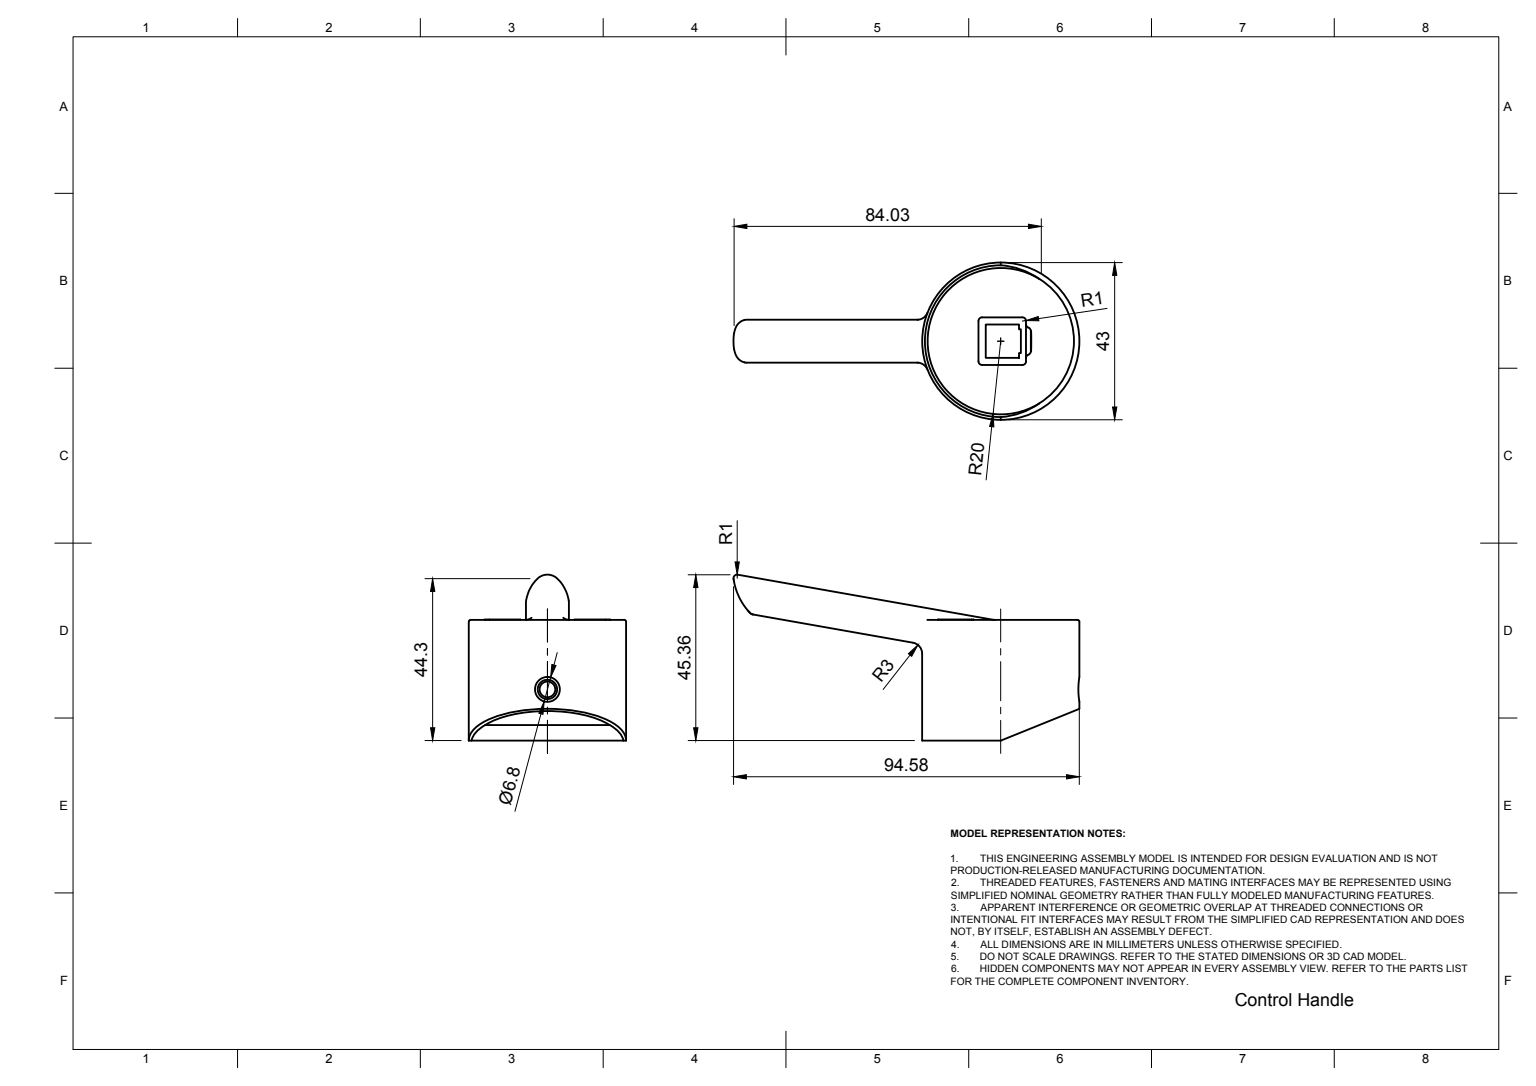
ISO-10303-21;
HEADER;
/* Generated by software containing ST-Developer
 * from STEP Tools, Inc. (www.steptools.com) 
 */

FILE_DESCRIPTION(
/* description */ ('STEP AP214'),
/* implementation_level */ '2;1');

FILE_NAME(
/* name */ 'Control Handle.step',
/* time_stamp */ '2026-10-05T23:18:41-07:00',
/* author */ (''),
/* organization */ (''),
/* preprocessor_version */ 'ST-DEVELOPER v20.2',
/* originating_system */ 'Autodesk Translation Framework v15.15.0.0',
/* authorisation */ '');

FILE_SCHEMA (('AUTOMOTIVE_DESIGN { 1 0 10303 214 3 1 1 }'));
ENDSEC;

DATA;
#10=MECHANICAL_DESIGN_GEOMETRIC_PRESENTATION_REPRESENTATION('',(#101),#221662);
#63=MANIFOLD_SOLID_BREP('Body1',#79323);
#75=SHAPE_REPRESENTATION_RELATIONSHIP('SRR','None',#221710,#88);
#88=ADVANCED_BREP_SHAPE_REPRESENTATION('',(#63),#221650);
#101=STYLED_ITEM('',(#221783),#63);
#176=B_SPLINE_SURFACE_WITH_KNOTS('',3,3,((#159336,#159337,#159338,#159339),
(#159340,#159341,#159342,#159343),(#159344,#159345,#159346,#159347),(#159348,
#159349,#159350,#159351),(#159352,#159353,#159354,#159355),(#159356,#159357,
#159358,#159359),(#159360,#159361,#159362,#159363),(#159364,#159365,#159366,
#159367),(#159368,#159369,#159370,#159371),(#159372,#159373,#159374,#159375),
(#159376,#159377,#159378,#159379),(#159380,#159381,#159382,#159383),(#159384,
#159385,#159386,#159387),(#159388,#159389,#159390,#159391),(#159392,#159393,
#159394,#159395),(#159396,#159397,#159398,#159399)),.UNSPECIFIED.,.F.,.F.,
 .F.,(4,1,1,1,1,1,1,1,1,1,1,1,1,4),(4,4),(0.,0.0631871049823428,0.143694780613763,
0.224202456245058,0.304710131876457,0.385217807507856,0.465725483139255,
0.54623315877055,0.626740834401949,0.707248510033348,0.787756185664748,
0.868263861296042,0.948771536927442,1.),(0.,1.),.UNSPECIFIED.);
#177=B_SPLINE_SURFACE_WITH_KNOTS('',3,3,((#159424,#159425,#159426,#159427),
(#159428,#159429,#159430,#159431),(#159432,#159433,#159434,#159435),(#159436,
#159437,#159438,#159439),(#159440,#159441,#159442,#159443),(#159444,#159445,
#159446,#159447),(#159448,#159449,#159450,#159451),(#159452,#159453,#159454,
#159455),(#159456,#159457,#159458,#159459),(#159460,#159461,#159462,#159463),
(#159464,#159465,#159466,#159467),(#159468,#159469,#159470,#159471),(#159472,
#159473,#159474,#159475),(#159476,#159477,#159478,#159479),(#159480,#159481,
#159482,#159483),(#159484,#159485,#159486,#159487)),.UNSPECIFIED.,.F.,.F.,
 .F.,(4,1,1,1,1,1,1,1,1,1,1,1,1,4),(4,4),(0.,0.063187150036898,0.143694817475814,
0.224202484914604,0.304710152353498,0.385217819792393,0.465725487231287,
0.546233154670077,0.626740822108972,0.707248489547867,0.787756156986761,
0.868263824425551,0.948771491864446,1.),(0.,1.),.UNSPECIFIED.);
#178=B_SPLINE_SURFACE_WITH_KNOTS('',3,1,((#159815,#159816),(#159817,#159818),
(#159819,#159820),(#159821,#159822)),.UNSPECIFIED.,.F.,.F.,.F.,(4,4),(2,
2),(0.00340538980800498,1.),(0.,1.18214433782264),.UNSPECIFIED.);
#269=FACE_BOUND('',#24594,.T.);
#270=FACE_BOUND('',#24605,.T.);
#271=FACE_BOUND('',#24611,.T.);
#272=FACE_BOUND('',#24616,.T.);
#273=FACE_BOUND('',#24644,.T.);
#274=FACE_BOUND('',#24645,.T.);
#1766=(
BOUNDED_CURVE()
B_SPLINE_CURVE(3,(#159803,#159804,#159805,#159806,#159807,#159808,#159809,
#159810,#159811,#159812,#159813),.UNSPECIFIED.,.F.,.F.)
B_SPLINE_CURVE_WITH_KNOTS((4,1,1,1,1,1,1,1,4),(0.,0.141779774422697,0.288564186808889,
0.419637721811095,0.537332459847568,0.657407795649981,0.783847578789506,
0.908572898255855,1.),.UNSPECIFIED.)
CURVE()
GEOMETRIC_REPRESENTATION_ITEM()
RATIONAL_B_SPLINE_CURVE((1.03357883859121,1.03357883859121,1.03357883859121,
1.03357883859121,1.03357883859121,1.03357883859121,1.03357883859121,1.03357883859121,
1.03357883859121,1.03357883859121,1.03357883859121))
REPRESENTATION_ITEM('')
);
#1767=(
BOUNDED_CURVE()
B_SPLINE_CURVE(3,(#159870,#159871,#159872,#159873,#159874,#159875,#159876),
 .UNSPECIFIED.,.F.,.F.)
B_SPLINE_CURVE_WITH_KNOTS((4,1,1,1,4),(0.,0.224667526957694,0.481948378364901,
0.749503179488002,1.),.UNSPECIFIED.)
CURVE()
GEOMETRIC_REPRESENTATION_ITEM()
RATIONAL_B_SPLINE_CURVE((1.24731983145218,1.24731983145218,1.24731983145218,
1.24731983145218,1.24731983145218,1.24731983145218,1.24731983145218))
REPRESENTATION_ITEM('')
);
#1768=(
BOUNDED_CURVE()
B_SPLINE_CURVE(3,(#159878,#159879,#159880,#159881,#159882,#159883,#159884,
#159885,#159886,#159887),.UNSPECIFIED.,.F.,.F.)
B_SPLINE_CURVE_WITH_KNOTS((4,1,1,1,1,1,1,4),(0.,0.122671457527971,0.275186389436719,
0.426161388513612,0.576657904418794,0.727651491077518,0.880206170558277,
1.),.UNSPECIFIED.)
CURVE()
GEOMETRIC_REPRESENTATION_ITEM()
RATIONAL_B_SPLINE_CURVE((1.26434380601904,1.26434380601904,1.26434380601904,
1.26434380601904,1.26434380601904,1.26434380601904,1.26434380601904,1.26434380601904,
1.26434380601904,1.26434380601904))
REPRESENTATION_ITEM('')
);
#1769=(
BOUNDED_CURVE()
B_SPLINE_CURVE(3,(#159888,#159889,#159890,#159891,#159892,#159893,#159894),
 .UNSPECIFIED.,.F.,.F.)
B_SPLINE_CURVE_WITH_KNOTS((4,1,1,1,4),(0.,0.253269801031687,0.52066383235046,
0.77788908313976,0.999999610731203),.UNSPECIFIED.)
CURVE()
GEOMETRIC_REPRESENTATION_ITEM()
RATIONAL_B_SPLINE_CURVE((1.24732214149726,1.24732214149726,1.24732214149726,
1.24732214149726,1.24732214149726,1.24732214149726,1.24732214149726))
REPRESENTATION_ITEM('')
);
#1878=TOROIDAL_SURFACE('',#80380,21.,0.5);
#1879=TOROIDAL_SURFACE('',#80400,18.5,1.5);
#1880=TOROIDAL_SURFACE('',#80403,2.866784855558,1.5);
#1881=TOROIDAL_SURFACE('',#80406,2.866784855558,1.5);
#1882=TOROIDAL_SURFACE('',#80441,2.866784855558,1.5);
#1883=TOROIDAL_SURFACE('',#80446,2.866784855558,1.5);
#1884=TOROIDAL_SURFACE('',#80451,2.866784855558,1.5);
#1885=TOROIDAL_SURFACE('',#80473,2.866784855558,1.5);
#1924=CONICAL_SURFACE('',#80396,20.37470056578,0.174533028825274);
#1925=CONICAL_SURFACE('',#80430,1.183506656857,0.0174532924999985);
#1926=CONICAL_SURFACE('',#80434,1.183506656857,0.0174532924999985);
#1927=CONICAL_SURFACE('',#80455,1.183506656857,0.0174532924999985);
#1928=CONICAL_SURFACE('',#80460,0.816493292676001,0.0174532924999985);
#1929=CONICAL_SURFACE('',#80464,1.189214422822,0.0174532924999985);
#1930=CONICAL_SURFACE('',#80467,1.189214422821,0.0174532924999985);
#1931=CONICAL_SURFACE('',#80476,1.183506656857,0.0174532924999985);
#1932=CONICAL_SURFACE('',#80479,0.816493289244397,0.0174532924999985);
#2150=CYLINDRICAL_SURFACE('',#80384,21.5);
#2151=CYLINDRICAL_SURFACE('',#80388,15.00000000001);
#2152=CYLINDRICAL_SURFACE('',#80389,20.);
#2153=CYLINDRICAL_SURFACE('',#80395,3.40000000000001);
#2154=CYLINDRICAL_SURFACE('',#80409,2.15);
#2155=CYLINDRICAL_SURFACE('',#80412,19.);
#2156=CYLINDRICAL_SURFACE('',#80417,17.5);
#2157=CYLINDRICAL_SURFACE('',#80423,19.);
#2158=CYLINDRICAL_SURFACE('',#80426,17.5);
#2159=CYLINDRICAL_SURFACE('',#80438,1.50000000000001);
#2160=CYLINDRICAL_SURFACE('',#80444,1.50000000000001);
#2161=CYLINDRICAL_SURFACE('',#80449,1.50000000000001);
#2162=CYLINDRICAL_SURFACE('',#80458,1.50000000000001);
#2163=CYLINDRICAL_SURFACE('',#80469,1.50000000000001);
#2164=CYLINDRICAL_SURFACE('',#80471,1.50000000000001);
#2165=CYLINDRICAL_SURFACE('',#80500,2.50000000000001);
#2166=CYLINDRICAL_SURFACE('',#80503,2.50000000000001);
#2167=CYLINDRICAL_SURFACE('',#80507,10.);
#2168=CYLINDRICAL_SURFACE('',#80512,10.);
#2169=CYLINDRICAL_SURFACE('',#80514,4.00000000000099);
#2615=(
BOUNDED_SURFACE()
B_SPLINE_SURFACE(3,3,((#159279,#159280,#159281,#159282,#159283,#159284,
#159285,#159286,#159287,#159288,#159289,#159290,#159291),(#159292,#159293,
#159294,#159295,#159296,#159297,#159298,#159299,#159300,#159301,#159302,
#159303,#159304),(#159305,#159306,#159307,#159308,#159309,#159310,#159311,
#159312,#159313,#159314,#159315,#159316,#159317),(#159318,#159319,#159320,
#159321,#159322,#159323,#159324,#159325,#159326,#159327,#159328,#159329,
#159330)),.UNSPECIFIED.,.F.,.F.,.F.)
B_SPLINE_SURFACE_WITH_KNOTS((4,4),(4,1,1,1,1,1,1,1,1,1,4),(0.,1.),(0.,0.0348134269562723,
0.158608211677217,0.280646015430893,0.400635489137686,0.518375328151176,
0.633927632286859,0.74698660160379,0.85748053072882,0.966231997819705,1.),
 .UNSPECIFIED.)
GEOMETRIC_REPRESENTATION_ITEM()
RATIONAL_B_SPLINE_SURFACE(((1.216775993711,1.216775993711,1.216775993711,
1.216775993711,1.216775993711,1.216775993711,1.216775993711,1.216775993711,
1.216775993711,1.216775993711,1.216775993711,1.216775993711,1.216775993711),
(0.9277413354296,0.9277413354296,0.9277413354296,0.9277413354296,0.9277413354296,
0.9277413354296,0.9277413354296,0.9277413354296,0.9277413354296,0.9277413354296,
0.9277413354296,0.9277413354296,0.9277413354296),(0.9277413354296,0.9277413354296,
0.9277413354296,0.9277413354296,0.9277413354296,0.9277413354296,0.9277413354296,
0.9277413354296,0.9277413354296,0.9277413354296,0.9277413354296,0.9277413354296,
0.9277413354296),(1.216775993711,1.216775993711,1.216775993711,1.216775993711,
1.216775993711,1.216775993711,1.216775993711,1.216775993711,1.216775993711,
1.216775993711,1.216775993711,1.216775993711,1.216775993711)))
REPRESENTATION_ITEM('')
SURFACE()
);
#2616=(
BOUNDED_SURFACE()
B_SPLINE_SURFACE(3,3,((#159523,#159524,#159525,#159526,#159527,#159528,
#159529,#159530,#159531,#159532,#159533,#159534,#159535),(#159536,#159537,
#159538,#159539,#159540,#159541,#159542,#159543,#159544,#159545,#159546,
#159547,#159548),(#159549,#159550,#159551,#159552,#159553,#159554,#159555,
#159556,#159557,#159558,#159559,#159560,#159561),(#159562,#159563,#159564,
#159565,#159566,#159567,#159568,#159569,#159570,#159571,#159572,#159573,
#159574)),.UNSPECIFIED.,.F.,.F.,.F.)
B_SPLINE_SURFACE_WITH_KNOTS((4,4),(4,1,1,1,1,1,1,1,1,1,4),(0.,1.),(0.,0.0348134437205886,
0.158607302135055,0.280647732326047,0.400637496360499,0.518378147625292,
0.633929635661477,0.746988357647408,0.857493579740769,0.966231987897078,
1.),.UNSPECIFIED.)
GEOMETRIC_REPRESENTATION_ITEM()
RATIONAL_B_SPLINE_SURFACE(((1.216775996933,1.216775996933,1.216775996933,
1.216775996933,1.216775996933,1.216775996933,1.216775996933,1.216775996933,
1.216775996933,1.216775996933,1.216775996933,1.216775996933,1.216775996933),
(0.9277413343557,0.9277413343557,0.9277413343557,0.9277413343557,0.9277413343557,
0.9277413343557,0.9277413343557,0.9277413343557,0.9277413343557,0.9277413343557,
0.9277413343557,0.9277413343557,0.9277413343557),(0.9277413343557,0.9277413343557,
0.9277413343557,0.9277413343557,0.9277413343557,0.9277413343557,0.9277413343557,
0.9277413343557,0.9277413343557,0.9277413343557,0.9277413343557,0.9277413343557,
0.9277413343557),(1.216775996933,1.216775996933,1.216775996933,1.216775996933,
1.216775996933,1.216775996933,1.216775996933,1.216775996933,1.216775996933,
1.216775996933,1.216775996933,1.216775996933,1.216775996933)))
REPRESENTATION_ITEM('')
SURFACE()
);
#2617=(
BOUNDED_SURFACE()
B_SPLINE_SURFACE(3,3,((#159756,#159757,#159758,#159759,#159760,#159761,
#159762,#159763,#159764,#159765,#159766),(#159767,#159768,#159769,#159770,
#159771,#159772,#159773,#159774,#159775,#159776,#159777),(#159778,#159779,
#159780,#159781,#159782,#159783,#159784,#159785,#159786,#159787,#159788),
(#159789,#159790,#159791,#159792,#159793,#159794,#159795,#159796,#159797,
#159798,#159799)),.UNSPECIFIED.,.F.,.F.,.F.)
B_SPLINE_SURFACE_WITH_KNOTS((4,4),(4,1,1,1,1,1,1,1,4),(0.,1.),(0.,0.148763869419657,
0.292686130252006,0.421203860344306,0.536603666842246,0.654337651793038,
0.778311983622731,0.900605282133238,1.),.UNSPECIFIED.)
GEOMETRIC_REPRESENTATION_ITEM()
RATIONAL_B_SPLINE_SURFACE(((1.068703746667,1.068703746667,1.068703746667,
1.068703746667,1.068703746667,1.068703746667,1.068703746667,1.068703746667,
1.068703746667,1.068703746667,1.068703746667),(0.9770987511109,0.9770987511109,
0.9770987511109,0.9770987511109,0.9770987511109,0.9770987511109,0.9770987511109,
0.9770987511109,0.9770987511109,0.9770987511109,0.9770987511109),(0.9770987511109,
0.9770987511109,0.9770987511109,0.9770987511109,0.9770987511109,0.9770987511109,
0.9770987511109,0.9770987511109,0.9770987511109,0.9770987511109,0.9770987511109),
(1.068703746667,1.068703746667,1.068703746667,1.068703746667,1.068703746667,
1.068703746667,1.068703746667,1.068703746667,1.068703746667,1.068703746667,
1.068703746667)))
REPRESENTATION_ITEM('')
SURFACE()
);
#2618=(
BOUNDED_SURFACE()
B_SPLINE_SURFACE(3,3,((#159895,#159896,#159897,#159898,#159899,#159900,
#159901,#159902,#159903,#159904),(#159905,#159906,#159907,#159908,#159909,
#159910,#159911,#159912,#159913,#159914),(#159915,#159916,#159917,#159918,
#159919,#159920,#159921,#159922,#159923,#159924),(#159925,#159926,#159927,
#159928,#159929,#159930,#159931,#159932,#159933,#159934)),.UNSPECIFIED.,
 .F.,.F.,.F.)
B_SPLINE_SURFACE_WITH_KNOTS((4,4),(4,1,1,1,1,1,1,4),(0.,1.),(0.,0.0982957502815311,
0.222717520122402,0.361997328765986,0.517413543628817,0.685998740299415,
0.858955544446863,1.),.UNSPECIFIED.)
GEOMETRIC_REPRESENTATION_ITEM()
RATIONAL_B_SPLINE_SURFACE(((1.298412003099,1.298412003099,1.298412003099,
1.298412003099,1.298412003099,1.298412003099,1.298412003099,1.298412003099,
1.298412003099,1.298412003099),(0.9005293323002,0.9005293323002,0.9005293323002,
0.9005293323002,0.9005293323002,0.9005293323002,0.9005293323002,0.9005293323002,
0.9005293323002,0.9005293323002),(0.9005293323002,0.9005293323002,0.9005293323002,
0.9005293323002,0.9005293323002,0.9005293323002,0.9005293323002,0.9005293323002,
0.9005293323002,0.9005293323002),(1.298412003099,1.298412003099,1.298412003099,
1.298412003099,1.298412003099,1.298412003099,1.298412003099,1.298412003099,
1.298412003099,1.298412003099)))
REPRESENTATION_ITEM('')
SURFACE()
);
#2619=(
BOUNDED_SURFACE()
B_SPLINE_SURFACE(3,3,((#160037,#160038,#160039,#160040,#160041,#160042,
#160043,#160044,#160045,#160046,#160047),(#160048,#160049,#160050,#160051,
#160052,#160053,#160054,#160055,#160056,#160057,#160058),(#160059,#160060,
#160061,#160062,#160063,#160064,#160065,#160066,#160067,#160068,#160069),
(#160070,#160071,#160072,#160073,#160074,#160075,#160076,#160077,#160078,
#160079,#160080)),.UNSPECIFIED.,.F.,.F.,.F.)
B_SPLINE_SURFACE_WITH_KNOTS((4,4),(4,1,1,1,1,1,1,1,4),(0.,1.),(0.,0.113847052245463,
0.256880770340595,0.393447274181346,0.529715276691642,0.664740251429543,
0.79675578013572,0.925830065497239,1.),.UNSPECIFIED.)
GEOMETRIC_REPRESENTATION_ITEM()
RATIONAL_B_SPLINE_SURFACE(((1.14428616678,1.14428616678,1.14428616678,1.14428616678,
1.14428616678,1.14428616678,1.14428616678,1.14428616678,1.14428616678,1.14428616678,
1.14428616678),(0.9519046110735,0.9519046110735,0.9519046110735,0.9519046110735,
0.9519046110735,0.9519046110735,0.9519046110735,0.9519046110735,0.9519046110735,
0.9519046110735,0.9519046110735),(0.9519046110735,0.9519046110735,0.9519046110735,
0.9519046110735,0.9519046110735,0.9519046110735,0.9519046110735,0.9519046110735,
0.9519046110735,0.9519046110735,0.9519046110735),(1.14428616678,1.14428616678,
1.14428616678,1.14428616678,1.14428616678,1.14428616678,1.14428616678,1.14428616678,
1.14428616678,1.14428616678,1.14428616678)))
REPRESENTATION_ITEM('')
SURFACE()
);
#2620=(
BOUNDED_SURFACE()
B_SPLINE_SURFACE(3,3,((#160180,#160181,#160182,#160183,#160184,#160185,
#160186,#160187,#160188,#160189,#160190),(#160191,#160192,#160193,#160194,
#160195,#160196,#160197,#160198,#160199,#160200,#160201),(#160202,#160203,
#160204,#160205,#160206,#160207,#160208,#160209,#160210,#160211,#160212),
(#160213,#160214,#160215,#160216,#160217,#160218,#160219,#160220,#160221,
#160222,#160223)),.UNSPECIFIED.,.F.,.F.,.F.)
B_SPLINE_SURFACE_WITH_KNOTS((4,4),(4,1,1,1,1,1,1,1,4),(0.,1.),(0.,0.0944145406001002,
0.22382893510453,0.356121659603939,0.491296333098967,0.627233999913856,
0.763922934472171,0.907653635910875,1.),.UNSPECIFIED.)
GEOMETRIC_REPRESENTATION_ITEM()
RATIONAL_B_SPLINE_SURFACE(((1.144284885867,1.144284885867,1.144284885867,
1.144284885867,1.144284885867,1.144284885867,1.144284885867,1.144284885867,
1.144284885867,1.144284885867,1.144284885867),(0.9519050380443,0.9519050380443,
0.9519050380443,0.9519050380443,0.9519050380443,0.9519050380443,0.9519050380443,
0.9519050380443,0.9519050380443,0.9519050380443,0.9519050380443),(0.9519050380443,
0.9519050380443,0.9519050380443,0.9519050380443,0.9519050380443,0.9519050380443,
0.9519050380443,0.9519050380443,0.9519050380443,0.9519050380443,0.9519050380443),
(1.144284885867,1.144284885867,1.144284885867,1.144284885867,1.144284885867,
1.144284885867,1.144284885867,1.144284885867,1.144284885867,1.144284885867,
1.144284885867)))
REPRESENTATION_ITEM('')
SURFACE()
);
#2621=(
BOUNDED_SURFACE()
B_SPLINE_SURFACE(3,3,((#160430,#160431,#160432,#160433,#160434,#160435,
#160436,#160437,#160438,#160439),(#160440,#160441,#160442,#160443,#160444,
#160445,#160446,#160447,#160448,#160449),(#160450,#160451,#160452,#160453,
#160454,#160455,#160456,#160457,#160458,#160459),(#160460,#160461,#160462,
#160463,#160464,#160465,#160466,#160467,#160468,#160469)),.UNSPECIFIED.,
 .F.,.F.,.F.)
B_SPLINE_SURFACE_WITH_KNOTS((4,4),(4,1,1,1,1,1,1,4),(0.,1.),(0.,0.146101495488384,
0.319452627218425,0.487967212214235,0.642996851728068,0.781791002263477,
0.905806643913708,1.),.UNSPECIFIED.)
GEOMETRIC_REPRESENTATION_ITEM()
RATIONAL_B_SPLINE_SURFACE(((1.298413325381,1.298413325381,1.298413325381,
1.298413325381,1.298413325381,1.298413325381,1.298413325381,1.298413325381,
1.298413325381,1.298413325381),(0.9005288915396,0.9005288915396,0.9005288915396,
0.9005288915396,0.9005288915396,0.9005288915396,0.9005288915396,0.9005288915396,
0.9005288915396,0.9005288915396),(0.9005288915396,0.9005288915396,0.9005288915396,
0.9005288915396,0.9005288915396,0.9005288915396,0.9005288915396,0.9005288915396,
0.9005288915396,0.9005288915396),(1.298413325381,1.298413325381,1.298413325381,
1.298413325381,1.298413325381,1.298413325381,1.298413325381,1.298413325381,
1.298413325381,1.298413325381)))
REPRESENTATION_ITEM('')
SURFACE()
);
#2622=(
BOUNDED_SURFACE()
B_SPLINE_SURFACE(3,3,((#160471,#160472,#160473,#160474,#160475,#160476,
#160477),(#160478,#160479,#160480,#160481,#160482,#160483,#160484),(#160485,
#160486,#160487,#160488,#160489,#160490,#160491),(#160492,#160493,#160494,
#160495,#160496,#160497,#160498)),.UNSPECIFIED.,.F.,.F.,.F.)
B_SPLINE_SURFACE_WITH_KNOTS((4,4),(4,1,1,1,4),(0.,1.),(0.,0.230593160213399,
0.482348490956705,0.744157121798399,1.),.UNSPECIFIED.)
GEOMETRIC_REPRESENTATION_ITEM()
RATIONAL_B_SPLINE_SURFACE(((1.353838625123,1.353838625123,1.353838625123,
1.353838625123,1.353838625123,1.353838625123,1.353838625123),(0.8820537916258,
0.8820537916258,0.8820537916258,0.8820537916258,0.8820537916258,0.8820537916258,
0.8820537916258),(0.8820537916258,0.8820537916258,0.8820537916258,0.8820537916258,
0.8820537916258,0.8820537916258,0.8820537916258),(1.353838625123,1.353838625123,
1.353838625123,1.353838625123,1.353838625123,1.353838625123,1.353838625123)))
REPRESENTATION_ITEM('')
SURFACE()
);
#2623=(
BOUNDED_SURFACE()
B_SPLINE_SURFACE(3,3,((#160516,#160517,#160518,#160519,#160520,#160521,
#160522,#160523,#160524,#160525),(#160526,#160527,#160528,#160529,#160530,
#160531,#160532,#160533,#160534,#160535),(#160536,#160537,#160538,#160539,
#160540,#160541,#160542,#160543,#160544,#160545),(#160546,#160547,#160548,
#160549,#160550,#160551,#160552,#160553,#160554,#160555)),.UNSPECIFIED.,
 .F.,.F.,.F.)
B_SPLINE_SURFACE_WITH_KNOTS((4,4),(4,1,1,1,1,1,1,4),(0.,1.),(0.,0.13457163316798,
0.282274649724905,0.428486319030034,0.574234601524777,0.720464271965091,
0.868205782040083,1.),.UNSPECIFIED.)
GEOMETRIC_REPRESENTATION_ITEM()
RATIONAL_B_SPLINE_SURFACE(((1.375941287385,1.375941287385,1.375941287385,
1.375941287385,1.375941287385,1.375941287385,1.375941287385,1.375941287385,
1.375941287385,1.375941287385),(0.8746862375382,0.8746862375382,0.8746862375382,
0.8746862375382,0.8746862375382,0.8746862375382,0.8746862375382,0.8746862375382,
0.8746862375382,0.8746862375382),(0.8746862375382,0.8746862375382,0.8746862375382,
0.8746862375382,0.8746862375382,0.8746862375382,0.8746862375382,0.8746862375382,
0.8746862375382,0.8746862375382),(1.375941287385,1.375941287385,1.375941287385,
1.375941287385,1.375941287385,1.375941287385,1.375941287385,1.375941287385,
1.375941287385,1.375941287385)))
REPRESENTATION_ITEM('')
SURFACE()
);
#2624=(
BOUNDED_SURFACE()
B_SPLINE_SURFACE(3,3,((#160619,#160620,#160621,#160622,#160623,#160624,
#160625),(#160626,#160627,#160628,#160629,#160630,#160631,#160632),(#160633,
#160634,#160635,#160636,#160637,#160638,#160639),(#160640,#160641,#160642,
#160643,#160644,#160645,#160646)),.UNSPECIFIED.,.F.,.F.,.F.)
B_SPLINE_SURFACE_WITH_KNOTS((4,4),(4,1,1,1,4),(0.,1.),(0.,0.266221048065604,
0.525168076403688,0.774267556960161,1.),.UNSPECIFIED.)
GEOMETRIC_REPRESENTATION_ITEM()
RATIONAL_B_SPLINE_SURFACE(((1.35383923737,1.35383923737,1.35383923737,1.35383923737,
1.35383923737,1.35383923737,1.35383923737),(0.8820535875433,0.8820535875433,
0.8820535875433,0.8820535875433,0.8820535875433,0.8820535875433,0.8820535875433),
(0.8820535875433,0.8820535875433,0.8820535875433,0.8820535875433,0.8820535875433,
0.8820535875433,0.8820535875433),(1.35383923737,1.35383923737,1.35383923737,
1.35383923737,1.35383923737,1.35383923737,1.35383923737)))
REPRESENTATION_ITEM('')
SURFACE()
);
#2625=(
BOUNDED_SURFACE()
B_SPLINE_SURFACE(3,3,((#160766,#160767,#160768,#160769,#160770,#160771),
(#160772,#160773,#160774,#160775,#160776,#160777),(#160778,#160779,#160780,
#160781,#160782,#160783),(#160784,#160785,#160786,#160787,#160788,#160789)),
 .UNSPECIFIED.,.F.,.F.,.F.)
B_SPLINE_SURFACE_WITH_KNOTS((4,4),(4,1,1,4),(0.,1.),(0.,0.343001553297945,
0.735822721578711,1.),.UNSPECIFIED.)
GEOMETRIC_REPRESENTATION_ITEM()
RATIONAL_B_SPLINE_SURFACE(((1.133911518843,1.133911518843,1.133911518843,
1.133911518843,1.133911518843,1.133911518843),(0.9553628270522,0.9553628270522,
0.9553628270522,0.9553628270522,0.9553628270522,0.9553628270522),(0.9553628270522,
0.9553628270522,0.9553628270522,0.9553628270522,0.9553628270522,0.9553628270522),
(1.133911518843,1.133911518843,1.133911518843,1.133911518843,1.133911518843,
1.133911518843)))
REPRESENTATION_ITEM('')
SURFACE()
);
#2626=(
BOUNDED_SURFACE()
B_SPLINE_SURFACE(3,3,((#160791,#160792,#160793,#160794,#160795,#160796),
(#160797,#160798,#160799,#160800,#160801,#160802),(#160803,#160804,#160805,
#160806,#160807,#160808),(#160809,#160810,#160811,#160812,#160813,#160814)),
 .UNSPECIFIED.,.F.,.F.,.F.)
B_SPLINE_SURFACE_WITH_KNOTS((4,4),(4,1,1,4),(0.,1.),(0.,0.326783840018485,
0.677637015410791,1.),.UNSPECIFIED.)
GEOMETRIC_REPRESENTATION_ITEM()
RATIONAL_B_SPLINE_SURFACE(((1.154127816646,1.154127816646,1.154127816646,
1.154127816646,1.154127816646,1.154127816646),(0.948624061118,0.948624061118,
0.948624061118,0.948624061118,0.948624061118,0.948624061118),(0.948624061118,
0.948624061118,0.948624061118,0.948624061118,0.948624061118,0.948624061118),
(1.154127816646,1.154127816646,1.154127816646,1.154127816646,1.154127816646,
1.154127816646)))
REPRESENTATION_ITEM('')
SURFACE()
);
#2627=(
BOUNDED_SURFACE()
B_SPLINE_SURFACE(3,3,((#160816,#160817,#160818,#160819,#160820,#160821),
(#160822,#160823,#160824,#160825,#160826,#160827),(#160828,#160829,#160830,
#160831,#160832,#160833),(#160834,#160835,#160836,#160837,#160838,#160839)),
 .UNSPECIFIED.,.F.,.F.,.F.)
B_SPLINE_SURFACE_WITH_KNOTS((4,4),(4,1,1,4),(0.,1.),(0.,0.325921012985495,
0.684444108359778,1.),.UNSPECIFIED.)
GEOMETRIC_REPRESENTATION_ITEM()
RATIONAL_B_SPLINE_SURFACE(((1.154128041374,1.154128041374,1.154128041374,
1.154128041374,1.154128041374,1.154128041374),(0.9486239862088,0.9486239862088,
0.9486239862088,0.9486239862088,0.9486239862088,0.9486239862088),(0.9486239862088,
0.9486239862088,0.9486239862088,0.9486239862088,0.9486239862088,0.9486239862088),
(1.154128041374,1.154128041374,1.154128041374,1.154128041374,1.154128041374,
1.154128041374)))
REPRESENTATION_ITEM('')
SURFACE()
);
#2628=(
BOUNDED_SURFACE()
B_SPLINE_SURFACE(3,3,((#160840,#160841,#160842,#160843,#160844,#160845),
(#160846,#160847,#160848,#160849,#160850,#160851),(#160852,#160853,#160854,
#160855,#160856,#160857),(#160858,#160859,#160860,#160861,#160862,#160863)),
 .UNSPECIFIED.,.F.,.F.,.F.)
B_SPLINE_SURFACE_WITH_KNOTS((4,4),(4,1,1,4),(0.,1.),(0.,0.298212289448515,
0.67415586424402,1.),.UNSPECIFIED.)
GEOMETRIC_REPRESENTATION_ITEM()
RATIONAL_B_SPLINE_SURFACE(((1.133911518295,1.133911518295,1.133911518295,
1.133911518295,1.133911518295,1.133911518295),(0.955362827235,0.955362827235,
0.955362827235,0.955362827235,0.955362827235,0.955362827235),(0.955362827235,
0.955362827235,0.955362827235,0.955362827235,0.955362827235,0.955362827235),
(1.133911518295,1.133911518295,1.133911518295,1.133911518295,1.133911518295,
1.133911518295)))
REPRESENTATION_ITEM('')
SURFACE()
);
#2629=(
BOUNDED_SURFACE()
B_SPLINE_SURFACE(3,3,((#161268,#161269,#161270,#161271,#161272,#161273,
#161274,#161275,#161276,#161277,#161278,#161279,#161280,#161281,#161282,
#161283,#161284,#161285,#161286,#161287,#161288,#161289,#161290,#161291,
#161292,#161293,#161294,#161295,#161296,#161297,#161298,#161299,#161300,
#161301,#161302,#161303,#161304,#161305,#161306,#161307),(#161308,#161309,
#161310,#161311,#161312,#161313,#161314,#161315,#161316,#161317,#161318,
#161319,#161320,#161321,#161322,#161323,#161324,#161325,#161326,#161327,
#161328,#161329,#161330,#161331,#161332,#161333,#161334,#161335,#161336,
#161337,#161338,#161339,#161340,#161341,#161342,#161343,#161344,#161345,
#161346,#161347),(#161348,#161349,#161350,#161351,#161352,#161353,#161354,
#161355,#161356,#161357,#161358,#161359,#161360,#161361,#161362,#161363,
#161364,#161365,#161366,#161367,#161368,#161369,#161370,#161371,#161372,
#161373,#161374,#161375,#161376,#161377,#161378,#161379,#161380,#161381,
#161382,#161383,#161384,#161385,#161386,#161387),(#161388,#161389,#161390,
#161391,#161392,#161393,#161394,#161395,#161396,#161397,#161398,#161399,
#161400,#161401,#161402,#161403,#161404,#161405,#161406,#161407,#161408,
#161409,#161410,#161411,#161412,#161413,#161414,#161415,#161416,#161417,
#161418,#161419,#161420,#161421,#161422,#161423,#161424,#161425,#161426,
#161427)),.UNSPECIFIED.,.F.,.F.,.F.)
B_SPLINE_SURFACE_WITH_KNOTS((4,4),(4,1,1,1,1,1,1,1,1,1,1,1,1,1,1,1,1,1,
1,1,1,1,1,1,1,1,1,1,1,1,1,1,1,1,1,1,1,4),(0.,1.),(0.,0.0080855657193485,
0.0596218558242468,0.106852501388389,0.150184164955898,0.19003235366263,
0.226816246755187,0.260884487830858,0.292377213220895,0.321411667226958,
0.348115402080392,0.372633477126632,0.395157121664735,0.415908415220206,
0.434997267820443,0.452409696784467,0.468313480733662,0.482712550753752,
0.495419214437213,0.507133333503985,0.519448003687265,0.533357648922,0.548832281415337,
0.566241232560042,0.585544933168279,0.606300542403394,0.628001557637231,
0.650281261920833,0.673235965567153,0.698456243264167,0.725991202217506,
0.755882932612454,0.78864738633083,0.824762418308521,0.864558914403212,
0.908348167961349,0.956921864249176,1.),.UNSPECIFIED.)
GEOMETRIC_REPRESENTATION_ITEM()
RATIONAL_B_SPLINE_SURFACE(((1.046091568931,1.046091568931,1.046091568931,
1.046091568931,1.046091568931,1.046091568931,1.046091568931,1.046091568931,
1.046091568931,1.046091568931,1.046091568931,1.046091568931,1.046091568931,
1.046091568931,1.046091568931,1.046091568931,1.046091568931,1.046091568931,
1.046091568931,1.046091568931,1.046091568931,1.046091568931,1.046091568931,
1.046091568931,1.046091568931,1.046091568931,1.046091568931,1.046091568931,
1.046091568931,1.046091568931,1.046091568931,1.046091568931,1.046091568931,
1.046091568931,1.046091568931,1.046091568931,1.046091568931,1.046091568931,
1.046091568931,1.046091568931),(0.9846361436895,0.9846361436895,0.9846361436895,
0.9846361436895,0.9846361436895,0.9846361436895,0.9846361436895,0.9846361436895,
0.9846361436895,0.9846361436895,0.9846361436895,0.9846361436895,0.9846361436895,
0.9846361436895,0.9846361436895,0.9846361436895,0.9846361436895,0.9846361436895,
0.9846361436895,0.9846361436895,0.9846361436895,0.9846361436895,0.9846361436895,
0.9846361436895,0.9846361436895,0.9846361436895,0.9846361436895,0.9846361436895,
0.9846361436895,0.9846361436895,0.9846361436895,0.9846361436895,0.9846361436895,
0.9846361436895,0.9846361436895,0.9846361436895,0.9846361436895,0.9846361436895,
0.9846361436895,0.9846361436895),(0.9846361436895,0.9846361436895,0.9846361436895,
0.9846361436895,0.9846361436895,0.9846361436895,0.9846361436895,0.9846361436895,
0.9846361436895,0.9846361436895,0.9846361436895,0.9846361436895,0.9846361436895,
0.9846361436895,0.9846361436895,0.9846361436895,0.9846361436895,0.9846361436895,
0.9846361436895,0.9846361436895,0.9846361436895,0.9846361436895,0.9846361436895,
0.9846361436895,0.9846361436895,0.9846361436895,0.9846361436895,0.9846361436895,
0.9846361436895,0.9846361436895,0.9846361436895,0.9846361436895,0.9846361436895,
0.9846361436895,0.9846361436895,0.9846361436895,0.9846361436895,0.9846361436895,
0.9846361436895,0.9846361436895),(1.046091568931,1.046091568931,1.046091568931,
1.046091568931,1.046091568931,1.046091568931,1.046091568931,1.046091568931,
1.046091568931,1.046091568931,1.046091568931,1.046091568931,1.046091568931,
1.046091568931,1.046091568931,1.046091568931,1.046091568931,1.046091568931,
1.046091568931,1.046091568931,1.046091568931,1.046091568931,1.046091568931,
1.046091568931,1.046091568931,1.046091568931,1.046091568931,1.046091568931,
1.046091568931,1.046091568931,1.046091568931,1.046091568931,1.046091568931,
1.046091568931,1.046091568931,1.046091568931,1.046091568931,1.046091568931,
1.046091568931,1.046091568931)))
REPRESENTATION_ITEM('')
SURFACE()
);
#2630=(
BOUNDED_SURFACE()
B_SPLINE_SURFACE(3,3,((#161772,#161773,#161774,#161775,#161776,#161777),
(#161778,#161779,#161780,#161781,#161782,#161783),(#161784,#161785,#161786,
#161787,#161788,#161789),(#161790,#161791,#161792,#161793,#161794,#161795)),
 .UNSPECIFIED.,.F.,.F.,.F.)
B_SPLINE_SURFACE_WITH_KNOTS((4,4),(4,1,1,4),(0.,1.),(0.,0.297847735602895,
0.685768611894679,1.),.UNSPECIFIED.)
GEOMETRIC_REPRESENTATION_ITEM()
RATIONAL_B_SPLINE_SURFACE(((1.064510917442,1.064510917442,1.064510917442,
1.064510917442,1.064510917442,1.064510917442),(0.9784963608528,0.9784963608528,
0.9784963608528,0.9784963608528,0.9784963608528,0.9784963608528),(0.9784963608528,
0.9784963608528,0.9784963608528,0.9784963608528,0.9784963608528,0.9784963608528),
(1.064510917442,1.064510917442,1.064510917442,1.064510917442,1.064510917442,
1.064510917442)))
REPRESENTATION_ITEM('')
SURFACE()
);
#2631=(
BOUNDED_SURFACE()
B_SPLINE_SURFACE(3,3,((#161798,#161799,#161800,#161801,#161802,#161803,
#161804,#161805,#161806,#161807,#161808,#161809,#161810,#161811),(#161812,
#161813,#161814,#161815,#161816,#161817,#161818,#161819,#161820,#161821,
#161822,#161823,#161824,#161825),(#161826,#161827,#161828,#161829,#161830,
#161831,#161832,#161833,#161834,#161835,#161836,#161837,#161838,#161839),
(#161840,#161841,#161842,#161843,#161844,#161845,#161846,#161847,#161848,
#161849,#161850,#161851,#161852,#161853)),.UNSPECIFIED.,.F.,.F.,.F.)
B_SPLINE_SURFACE_WITH_KNOTS((4,4),(4,1,1,1,1,1,1,1,1,1,1,4),(0.,1.),(0.,
0.0507109297548065,0.123516716092259,0.193792769620065,0.266862729149513,
0.34659901892772,0.435171212264714,0.53358024119019,0.644372653483454,0.767724369233791,
0.895033447798833,1.),.UNSPECIFIED.)
GEOMETRIC_REPRESENTATION_ITEM()
RATIONAL_B_SPLINE_SURFACE(((1.133915806589,1.133915806589,1.133915806589,
1.133915806589,1.133915806589,1.133915806589,1.133915806589,1.133915806589,
1.133915806589,1.133915806589,1.133915806589,1.133915806589,1.133915806589,
1.133915806589),(0.9553613978037,0.9553613978037,0.9553613978037,0.9553613978037,
0.9553613978037,0.9553613978037,0.9553613978037,0.9553613978037,0.9553613978037,
0.9553613978037,0.9553613978037,0.9553613978037,0.9553613978037,0.9553613978037),
(0.9553613978037,0.9553613978037,0.9553613978037,0.9553613978037,0.9553613978037,
0.9553613978037,0.9553613978037,0.9553613978037,0.9553613978037,0.9553613978037,
0.9553613978037,0.9553613978037,0.9553613978037,0.9553613978037),(1.133915806589,
1.133915806589,1.133915806589,1.133915806589,1.133915806589,1.133915806589,
1.133915806589,1.133915806589,1.133915806589,1.133915806589,1.133915806589,
1.133915806589,1.133915806589,1.133915806589)))
REPRESENTATION_ITEM('')
SURFACE()
);
#2632=(
BOUNDED_SURFACE()
B_SPLINE_SURFACE(3,3,((#161854,#161855,#161856,#161857,#161858,#161859,
#161860,#161861,#161862,#161863,#161864,#161865,#161866,#161867),(#161868,
#161869,#161870,#161871,#161872,#161873,#161874,#161875,#161876,#161877,
#161878,#161879,#161880,#161881),(#161882,#161883,#161884,#161885,#161886,
#161887,#161888,#161889,#161890,#161891,#161892,#161893,#161894,#161895),
(#161896,#161897,#161898,#161899,#161900,#161901,#161902,#161903,#161904,
#161905,#161906,#161907,#161908,#161909)),.UNSPECIFIED.,.F.,.F.,.F.)
B_SPLINE_SURFACE_WITH_KNOTS((4,4),(4,1,1,1,1,1,1,1,1,1,1,4),(0.,1.),(0.,
0.104814911231639,0.230943732857245,0.351656664711374,0.461900769684698,
0.561079572404948,0.649863357676646,0.729556548498204,0.802369461782467,
0.872320141269624,0.94477376676948,1.),.UNSPECIFIED.)
GEOMETRIC_REPRESENTATION_ITEM()
RATIONAL_B_SPLINE_SURFACE(((1.133915819794,1.133915819794,1.133915819794,
1.133915819794,1.133915819794,1.133915819794,1.133915819794,1.133915819794,
1.133915819794,1.133915819794,1.133915819794,1.133915819794,1.133915819794,
1.133915819794),(0.955361393402,0.955361393402,0.955361393402,0.955361393402,
0.955361393402,0.955361393402,0.955361393402,0.955361393402,0.955361393402,
0.955361393402,0.955361393402,0.955361393402,0.955361393402,0.955361393402),
(0.955361393402,0.955361393402,0.955361393402,0.955361393402,0.955361393402,
0.955361393402,0.955361393402,0.955361393402,0.955361393402,0.955361393402,
0.955361393402,0.955361393402,0.955361393402,0.955361393402),(1.133915819794,
1.133915819794,1.133915819794,1.133915819794,1.133915819794,1.133915819794,
1.133915819794,1.133915819794,1.133915819794,1.133915819794,1.133915819794,
1.133915819794,1.133915819794,1.133915819794)))
REPRESENTATION_ITEM('')
SURFACE()
);
#2633=(
BOUNDED_SURFACE()
B_SPLINE_SURFACE(3,3,((#161911,#161912,#161913,#161914,#161915,#161916),
(#161917,#161918,#161919,#161920,#161921,#161922),(#161923,#161924,#161925,
#161926,#161927,#161928),(#161929,#161930,#161931,#161932,#161933,#161934)),
 .UNSPECIFIED.,.F.,.F.,.F.)
B_SPLINE_SURFACE_WITH_KNOTS((4,4),(4,1,1,4),(0.,1.),(0.,0.325174256189807,
0.72869537342957,1.),.UNSPECIFIED.)
GEOMETRIC_REPRESENTATION_ITEM()
RATIONAL_B_SPLINE_SURFACE(((1.064511164288,1.064511164288,1.064511164288,
1.064511164288,1.064511164288,1.064511164288),(0.9784962785707,0.9784962785707,
0.9784962785707,0.9784962785707,0.9784962785707,0.9784962785707),(0.9784962785707,
0.9784962785707,0.9784962785707,0.9784962785707,0.9784962785707,0.9784962785707),
(1.064511164288,1.064511164288,1.064511164288,1.064511164288,1.064511164288,
1.064511164288)))
REPRESENTATION_ITEM('')
SURFACE()
);
#2683=ELLIPSE('',#80385,23.1884969675686,21.5);
#2684=ELLIPSE('',#80387,23.1884969675686,21.5);
#2685=ELLIPSE('',#80391,21.5706948535507,20.0000000000001);
#2686=ELLIPSE('',#80394,21.5706948535507,20.0000000000001);
#2687=ELLIPSE('',#80397,22.4931093186433,20.8022577124141);
#2688=ELLIPSE('',#80399,22.4931093186513,20.8022577124259);
#2689=ELLIPSE('',#80461,1.38995187870583,0.982694699824574);
#2690=ELLIPSE('',#80465,1.42205238917504,1.00538969185979);
#2691=ELLIPSE('',#80468,1.42205238916912,1.00538969185822);
#2692=ELLIPSE('',#80480,1.38995186236733,0.982694649787225);
#2693=ELLIPSE('',#80508,57.0184616553497,7.46584982016915);
#2694=ELLIPSE('',#80513,64.4723561020752,8.58068888240209);
#2695=ELLIPSE('',#80518,60.7406503949971,10.3416271531119);
#2696=ELLIPSE('',#80520,62.3232622923384,10.641597160497);
#2956=LINE('',#158442,#10023);
#2957=LINE('',#158463,#10024);
#2958=LINE('',#158665,#10025);
#2959=LINE('',#158710,#10026);
#2960=LINE('',#158718,#10027);
#2961=LINE('',#158739,#10028);
#2962=LINE('',#158764,#10029);
#2963=LINE('',#159026,#10030);
#2964=LINE('',#159059,#10031);
#2965=LINE('',#159061,#10032);
#2966=LINE('',#159063,#10033);
#2967=LINE('',#159064,#10034);
#2968=LINE('',#159070,#10035);
#2969=LINE('',#159074,#10036);
#2970=LINE('',#159078,#10037);
#2971=LINE('',#159080,#10038);
#2972=LINE('',#159086,#10039);
#2973=LINE('',#159089,#10040);
#2974=LINE('',#159092,#10041);
#2975=LINE('',#159094,#10042);
#2976=LINE('',#159098,#10043);
#2977=LINE('',#159099,#10044);
#2978=LINE('',#159102,#10045);
#2979=LINE('',#159105,#10046);
#2980=LINE('',#159109,#10047);
#2981=LINE('',#159111,#10048);
#2982=LINE('',#159113,#10049);
#2983=LINE('',#159114,#10050);
#2984=LINE('',#159119,#10051);
#2985=LINE('',#159123,#10052);
#2986=LINE('',#159125,#10053);
#2987=LINE('',#159126,#10054);
#2988=LINE('',#159131,#10055);
#2989=LINE('',#159135,#10056);
#2990=LINE('',#159137,#10057);
#2991=LINE('',#159138,#10058);
#2992=LINE('',#159144,#10059);
#2993=LINE('',#159152,#10060);
#2994=LINE('',#159160,#10061);
#2995=LINE('',#159169,#10062);
#2996=LINE('',#159173,#10063);
#2997=LINE('',#159175,#10064);
#2998=LINE('',#159176,#10065);
#2999=LINE('',#159334,#10066);
#3000=LINE('',#159510,#10067);
#3001=LINE('',#159512,#10068);
#3002=LINE('',#159516,#10069);
#3003=LINE('',#159517,#10070);
#3004=LINE('',#159518,#10071);
#3005=LINE('',#159522,#10072);
#3006=LINE('',#159685,#10073);
#3007=LINE('',#159692,#10074);
#3008=LINE('',#159695,#10075);
#3009=LINE('',#159696,#10076);
#3010=LINE('',#159700,#10077);
#3011=LINE('',#159704,#10078);
#3012=LINE('',#159706,#10079);
#3013=LINE('',#159708,#10080);
#3014=LINE('',#159710,#10081);
#3015=LINE('',#159712,#10082);
#3016=LINE('',#159714,#10083);
#3017=LINE('',#159716,#10084);
#3018=LINE('',#159717,#10085);
#3019=LINE('',#159720,#10086);
#3020=LINE('',#159722,#10087);
#3021=LINE('',#159723,#10088);
#3022=LINE('',#159726,#10089);
#3023=LINE('',#159727,#10090);
#3024=LINE('',#159730,#10091);
#3025=LINE('',#159731,#10092);
#3026=LINE('',#159734,#10093);
#3027=LINE('',#159735,#10094);
#3028=LINE('',#159738,#10095);
#3029=LINE('',#159739,#10096);
#3030=LINE('',#159742,#10097);
#3031=LINE('',#159743,#10098);
#3032=LINE('',#159746,#10099);
#3033=LINE('',#159747,#10100);
#3034=LINE('',#159749,#10101);
#3035=LINE('',#159753,#10102);
#3036=LINE('',#159754,#10103);
#3037=LINE('',#160179,#10104);
#3038=LINE('',#160332,#10105);
#3039=LINE('',#160675,#10106);
#3040=LINE('',#160980,#10107);
#10023=VECTOR('',#88225,21.5);
#10024=VECTOR('',#88226,21.5);
#10025=VECTOR('',#88235,10.);
#10026=VECTOR('',#88236,10.);
#10027=VECTOR('',#88243,20.);
#10028=VECTOR('',#88244,20.);
#10029=VECTOR('',#88253,3.40000000000001);
#10030=VECTOR('',#88282,2.15);
#10031=VECTOR('',#88287,1000.);
#10032=VECTOR('',#88288,1000.);
#10033=VECTOR('',#88289,1000.);
#10034=VECTOR('',#88290,1000.);
#10035=VECTOR('',#88297,1000.);
#10036=VECTOR('',#88302,1000.);
#10037=VECTOR('',#88307,1000.);
#10038=VECTOR('',#88310,1000.);
#10039=VECTOR('',#88315,1000.);
#10040=VECTOR('',#88318,1000.);
#10041=VECTOR('',#88321,1000.);
#10042=VECTOR('',#88322,1000.);
#10043=VECTOR('',#88327,1000.);
#10044=VECTOR('',#88328,1000.);
#10045=VECTOR('',#88331,1000.);
#10046=VECTOR('',#88336,1000.);
#10047=VECTOR('',#88339,1000.);
#10048=VECTOR('',#88340,1000.);
#10049=VECTOR('',#88341,1000.);
#10050=VECTOR('',#88342,1000.);
#10051=VECTOR('',#88347,1000.);
#10052=VECTOR('',#88352,1000.);
#10053=VECTOR('',#88353,1000.);
#10054=VECTOR('',#88354,1000.);
#10055=VECTOR('',#88359,1000.);
#10056=VECTOR('',#88364,1000.);
#10057=VECTOR('',#88365,1000.);
#10058=VECTOR('',#88366,1000.);
#10059=VECTOR('',#88373,1000.);
#10060=VECTOR('',#88384,1000.);
#10061=VECTOR('',#88395,1000.);
#10062=VECTOR('',#88406,1000.);
#10063=VECTOR('',#88411,1000.);
#10064=VECTOR('',#88412,1000.);
#10065=VECTOR('',#88413,1000.);
#10066=VECTOR('',#88420,1000.);
#10067=VECTOR('',#88429,1000.);
#10068=VECTOR('',#88430,1000.);
#10069=VECTOR('',#88435,1000.);
#10070=VECTOR('',#88436,1000.);
#10071=VECTOR('',#88437,1000.);
#10072=VECTOR('',#88444,1000.);
#10073=VECTOR('',#88451,1000.);
#10074=VECTOR('',#88462,1000.);
#10075=VECTOR('',#88465,1000.);
#10076=VECTOR('',#88466,1000.);
#10077=VECTOR('',#88473,1000.);
#10078=VECTOR('',#88476,1000.);
#10079=VECTOR('',#88477,1000.);
#10080=VECTOR('',#88478,1000.);
#10081=VECTOR('',#88479,1000.);
#10082=VECTOR('',#88480,1000.);
#10083=VECTOR('',#88481,1000.);
#10084=VECTOR('',#88482,1000.);
#10085=VECTOR('',#88483,1000.);
#10086=VECTOR('',#88486,1000.);
#10087=VECTOR('',#88487,1000.);
#10088=VECTOR('',#88488,1000.);
#10089=VECTOR('',#88491,1000.);
#10090=VECTOR('',#88492,1000.);
#10091=VECTOR('',#88495,1000.);
#10092=VECTOR('',#88496,1000.);
#10093=VECTOR('',#88499,1000.);
#10094=VECTOR('',#88500,1000.);
#10095=VECTOR('',#88503,1000.);
#10096=VECTOR('',#88504,1000.);
#10097=VECTOR('',#88507,1000.);
#10098=VECTOR('',#88508,1000.);
#10099=VECTOR('',#88511,1000.);
#10100=VECTOR('',#88512,1000.);
#10101=VECTOR('',#88515,1000.);
#10102=VECTOR('',#88522,1000.);
#10103=VECTOR('',#88523,1000.);
#10104=VECTOR('',#88538,1000.);
#10105=VECTOR('',#88545,1000.);
#10106=VECTOR('',#88554,1000.);
#10107=VECTOR('',#88567,1000.);
#16916=PLANE('',#80411);
#16917=PLANE('',#80415);
#16918=PLANE('',#80419);
#16919=PLANE('',#80420);
#16920=PLANE('',#80425);
#16921=PLANE('',#80428);
#16922=PLANE('',#80429);
#16923=PLANE('',#80433);
#16924=PLANE('',#80437);
#16925=PLANE('',#80457);
#16926=PLANE('',#80466);
#16927=PLANE('',#80478);
#16928=PLANE('',#80481);
#16929=PLANE('',#80482);
#16930=PLANE('',#80483);
#16931=PLANE('',#80484);
#16932=PLANE('',#80485);
#16933=PLANE('',#80486);
#16934=PLANE('',#80487);
#16935=PLANE('',#80488);
#16936=PLANE('',#80489);
#16937=PLANE('',#80490);
#16938=PLANE('',#80491);
#16939=PLANE('',#80492);
#16940=PLANE('',#80493);
#16941=PLANE('',#80494);
#16942=PLANE('',#80521);
#20515=FACE_OUTER_BOUND('',#24554,.T.);
#20516=FACE_OUTER_BOUND('',#24555,.T.);
#20517=FACE_OUTER_BOUND('',#24556,.T.);
#20518=FACE_OUTER_BOUND('',#24557,.T.);
#20519=FACE_OUTER_BOUND('',#24558,.T.);
#20520=FACE_OUTER_BOUND('',#24559,.T.);
#20521=FACE_OUTER_BOUND('',#24560,.T.);
#20522=FACE_OUTER_BOUND('',#24561,.T.);
#20523=FACE_OUTER_BOUND('',#24562,.T.);
#20524=FACE_OUTER_BOUND('',#24563,.T.);
#20525=FACE_OUTER_BOUND('',#24564,.T.);
#20526=FACE_OUTER_BOUND('',#24565,.T.);
#20527=FACE_OUTER_BOUND('',#24566,.T.);
#20528=FACE_OUTER_BOUND('',#24567,.T.);
#20529=FACE_OUTER_BOUND('',#24568,.T.);
#20530=FACE_OUTER_BOUND('',#24569,.T.);
#20531=FACE_OUTER_BOUND('',#24570,.T.);
#20532=FACE_OUTER_BOUND('',#24571,.T.);
#20533=FACE_OUTER_BOUND('',#24572,.T.);
#20534=FACE_OUTER_BOUND('',#24573,.T.);
#20535=FACE_OUTER_BOUND('',#24574,.T.);
#20536=FACE_OUTER_BOUND('',#24575,.T.);
#20537=FACE_OUTER_BOUND('',#24576,.T.);
#20538=FACE_OUTER_BOUND('',#24577,.T.);
#20539=FACE_OUTER_BOUND('',#24578,.T.);
#20540=FACE_OUTER_BOUND('',#24579,.T.);
#20541=FACE_OUTER_BOUND('',#24580,.T.);
#20542=FACE_OUTER_BOUND('',#24581,.T.);
#20543=FACE_OUTER_BOUND('',#24582,.T.);
#20544=FACE_OUTER_BOUND('',#24583,.T.);
#20545=FACE_OUTER_BOUND('',#24584,.T.);
#20546=FACE_OUTER_BOUND('',#24585,.T.);
#20547=FACE_OUTER_BOUND('',#24586,.T.);
#20548=FACE_OUTER_BOUND('',#24587,.T.);
#20549=FACE_OUTER_BOUND('',#24588,.T.);
#20550=FACE_OUTER_BOUND('',#24589,.T.);
#20551=FACE_OUTER_BOUND('',#24590,.T.);
#20552=FACE_OUTER_BOUND('',#24591,.T.);
#20553=FACE_OUTER_BOUND('',#24592,.T.);
#20554=FACE_OUTER_BOUND('',#24593,.T.);
#20555=FACE_OUTER_BOUND('',#24595,.T.);
#20556=FACE_OUTER_BOUND('',#24596,.T.);
#20557=FACE_OUTER_BOUND('',#24597,.T.);
#20558=FACE_OUTER_BOUND('',#24598,.T.);
#20559=FACE_OUTER_BOUND('',#24599,.T.);
#20560=FACE_OUTER_BOUND('',#24600,.T.);
#20561=FACE_OUTER_BOUND('',#24601,.T.);
#20562=FACE_OUTER_BOUND('',#24602,.T.);
#20563=FACE_OUTER_BOUND('',#24603,.T.);
#20564=FACE_OUTER_BOUND('',#24604,.T.);
#20565=FACE_OUTER_BOUND('',#24606,.T.);
#20566=FACE_OUTER_BOUND('',#24607,.T.);
#20567=FACE_OUTER_BOUND('',#24608,.T.);
#20568=FACE_OUTER_BOUND('',#24609,.T.);
#20569=FACE_OUTER_BOUND('',#24610,.T.);
#20570=FACE_OUTER_BOUND('',#24612,.T.);
#20571=FACE_OUTER_BOUND('',#24613,.T.);
#20572=FACE_OUTER_BOUND('',#24614,.T.);
#20573=FACE_OUTER_BOUND('',#24615,.T.);
#20574=FACE_OUTER_BOUND('',#24617,.T.);
#20575=FACE_OUTER_BOUND('',#24618,.T.);
#20576=FACE_OUTER_BOUND('',#24619,.T.);
#20577=FACE_OUTER_BOUND('',#24620,.T.);
#20578=FACE_OUTER_BOUND('',#24621,.T.);
#20579=FACE_OUTER_BOUND('',#24622,.T.);
#20580=FACE_OUTER_BOUND('',#24623,.T.);
#20581=FACE_OUTER_BOUND('',#24624,.T.);
#20582=FACE_OUTER_BOUND('',#24625,.T.);
#20583=FACE_OUTER_BOUND('',#24626,.T.);
#20584=FACE_OUTER_BOUND('',#24627,.T.);
#20585=FACE_OUTER_BOUND('',#24628,.T.);
#20586=FACE_OUTER_BOUND('',#24629,.T.);
#20587=FACE_OUTER_BOUND('',#24630,.T.);
#20588=FACE_OUTER_BOUND('',#24631,.T.);
#20589=FACE_OUTER_BOUND('',#24632,.T.);
#20590=FACE_OUTER_BOUND('',#24633,.T.);
#20591=FACE_OUTER_BOUND('',#24634,.T.);
#20592=FACE_OUTER_BOUND('',#24635,.T.);
#20593=FACE_OUTER_BOUND('',#24636,.T.);
#20594=FACE_OUTER_BOUND('',#24637,.T.);
#20595=FACE_OUTER_BOUND('',#24638,.T.);
#20596=FACE_OUTER_BOUND('',#24639,.T.);
#20597=FACE_OUTER_BOUND('',#24640,.T.);
#20598=FACE_OUTER_BOUND('',#24641,.T.);
#20599=FACE_OUTER_BOUND('',#24642,.T.);
#20600=FACE_OUTER_BOUND('',#24643,.T.);
#24554=EDGE_LOOP('',(#55523,#55524,#55525,#55526,#55527));
#24555=EDGE_LOOP('',(#55528,#55529,#55530,#55531,#55532,#55533,#55534,#55535,
#55536,#55537,#55538,#55539,#55540,#55541,#55542,#55543,#55544));
#24556=EDGE_LOOP('',(#55545,#55546,#55547,#55548,#55549,#55550));
#24557=EDGE_LOOP('',(#55551,#55552,#55553,#55554,#55555,#55556,#55557,#55558,
#55559,#55560,#55561));
#24558=EDGE_LOOP('',(#55562,#55563,#55564,#55565,#55566,#55567));
#24559=EDGE_LOOP('',(#55568,#55569,#55570,#55571));
#24560=EDGE_LOOP('',(#55572,#55573,#55574,#55575,#55576));
#24561=EDGE_LOOP('',(#55577,#55578,#55579,#55580,#55581));
#24562=EDGE_LOOP('',(#55582,#55583,#55584,#55585,#55586));
#24563=EDGE_LOOP('',(#55587,#55588,#55589,#55590,#55591));
#24564=EDGE_LOOP('',(#55592,#55593,#55594,#55595));
#24565=EDGE_LOOP('',(#55596,#55597,#55598,#55599));
#24566=EDGE_LOOP('',(#55600,#55601,#55602,#55603));
#24567=EDGE_LOOP('',(#55604,#55605,#55606,#55607));
#24568=EDGE_LOOP('',(#55608,#55609,#55610,#55611));
#24569=EDGE_LOOP('',(#55612,#55613,#55614,#55615));
#24570=EDGE_LOOP('',(#55616,#55617,#55618,#55619));
#24571=EDGE_LOOP('',(#55620,#55621,#55622,#55623));
#24572=EDGE_LOOP('',(#55624,#55625,#55626,#55627));
#24573=EDGE_LOOP('',(#55628,#55629,#55630,#55631));
#24574=EDGE_LOOP('',(#55632,#55633,#55634,#55635));
#24575=EDGE_LOOP('',(#55636,#55637,#55638,#55639));
#24576=EDGE_LOOP('',(#55640,#55641,#55642,#55643));
#24577=EDGE_LOOP('',(#55644,#55645,#55646,#55647));
#24578=EDGE_LOOP('',(#55648,#55649,#55650,#55651));
#24579=EDGE_LOOP('',(#55652,#55653,#55654,#55655));
#24580=EDGE_LOOP('',(#55656,#55657,#55658,#55659));
#24581=EDGE_LOOP('',(#55660,#55661,#55662,#55663));
#24582=EDGE_LOOP('',(#55664,#55665,#55666,#55667));
#24583=EDGE_LOOP('',(#55668,#55669,#55670,#55671));
#24584=EDGE_LOOP('',(#55672,#55673,#55674,#55675));
#24585=EDGE_LOOP('',(#55676,#55677,#55678,#55679));
#24586=EDGE_LOOP('',(#55680,#55681,#55682,#55683));
#24587=EDGE_LOOP('',(#55684,#55685,#55686,#55687));
#24588=EDGE_LOOP('',(#55688,#55689,#55690));
#24589=EDGE_LOOP('',(#55691,#55692,#55693,#55694));
#24590=EDGE_LOOP('',(#55695,#55696,#55697,#55698));
#24591=EDGE_LOOP('',(#55699,#55700,#55701,#55702));
#24592=EDGE_LOOP('',(#55703,#55704,#55705,#55706));
#24593=EDGE_LOOP('',(#55707,#55708,#55709,#55710));
#24594=EDGE_LOOP('',(#55711,#55712));
#24595=EDGE_LOOP('',(#55713,#55714,#55715,#55716));
#24596=EDGE_LOOP('',(#55717,#55718,#55719,#55720));
#24597=EDGE_LOOP('',(#55721,#55722,#55723));
#24598=EDGE_LOOP('',(#55724,#55725,#55726,#55727));
#24599=EDGE_LOOP('',(#55728,#55729,#55730,#55731));
#24600=EDGE_LOOP('',(#55732,#55733,#55734,#55735));
#24601=EDGE_LOOP('',(#55736,#55737,#55738,#55739));
#24602=EDGE_LOOP('',(#55740,#55741,#55742,#55743));
#24603=EDGE_LOOP('',(#55744,#55745,#55746,#55747,#55748,#55749));
#24604=EDGE_LOOP('',(#55750,#55751,#55752,#55753,#55754,#55755,#55756,#55757,
#55758,#55759));
#24605=EDGE_LOOP('',(#55760,#55761,#55762,#55763,#55764,#55765,#55766,#55767));
#24606=EDGE_LOOP('',(#55768,#55769,#55770,#55771));
#24607=EDGE_LOOP('',(#55772,#55773,#55774,#55775));
#24608=EDGE_LOOP('',(#55776,#55777,#55778,#55779));
#24609=EDGE_LOOP('',(#55780,#55781,#55782,#55783));
#24610=EDGE_LOOP('',(#55784,#55785,#55786,#55787));
#24611=EDGE_LOOP('',(#55788));
#24612=EDGE_LOOP('',(#55789,#55790,#55791,#55792));
#24613=EDGE_LOOP('',(#55793,#55794,#55795,#55796));
#24614=EDGE_LOOP('',(#55797,#55798,#55799,#55800));
#24615=EDGE_LOOP('',(#55801));
#24616=EDGE_LOOP('',(#55802,#55803,#55804,#55805,#55806,#55807,#55808,#55809,
#55810,#55811,#55812,#55813,#55814,#55815));
#24617=EDGE_LOOP('',(#55816,#55817,#55818,#55819,#55820,#55821,#55822,#55823));
#24618=EDGE_LOOP('',(#55824,#55825,#55826,#55827,#55828,#55829,#55830,#55831));
#24619=EDGE_LOOP('',(#55832,#55833,#55834,#55835));
#24620=EDGE_LOOP('',(#55836,#55837,#55838,#55839,#55840));
#24621=EDGE_LOOP('',(#55841,#55842,#55843,#55844,#55845,#55846));
#24622=EDGE_LOOP('',(#55847,#55848,#55849,#55850));
#24623=EDGE_LOOP('',(#55851,#55852,#55853,#55854));
#24624=EDGE_LOOP('',(#55855,#55856,#55857,#55858));
#24625=EDGE_LOOP('',(#55859,#55860,#55861,#55862));
#24626=EDGE_LOOP('',(#55863,#55864,#55865,#55866));
#24627=EDGE_LOOP('',(#55867,#55868,#55869,#55870));
#24628=EDGE_LOOP('',(#55871,#55872,#55873,#55874));
#24629=EDGE_LOOP('',(#55875,#55876,#55877,#55878));
#24630=EDGE_LOOP('',(#55879,#55880,#55881,#55882));
#24631=EDGE_LOOP('',(#55883,#55884,#55885,#55886,#55887,#55888));
#24632=EDGE_LOOP('',(#55889,#55890,#55891,#55892));
#24633=EDGE_LOOP('',(#55893,#55894,#55895,#55896));
#24634=EDGE_LOOP('',(#55897,#55898,#55899,#55900));
#24635=EDGE_LOOP('',(#55901,#55902,#55903,#55904));
#24636=EDGE_LOOP('',(#55905,#55906,#55907,#55908,#55909,#55910));
#24637=EDGE_LOOP('',(#55911,#55912,#55913,#55914));
#24638=EDGE_LOOP('',(#55915,#55916,#55917,#55918));
#24639=EDGE_LOOP('',(#55919,#55920,#55921,#55922));
#24640=EDGE_LOOP('',(#55923,#55924,#55925,#55926));
#24641=EDGE_LOOP('',(#55927,#55928,#55929,#55930));
#24642=EDGE_LOOP('',(#55931,#55932,#55933,#55934));
#24643=EDGE_LOOP('',(#55935,#55936,#55937,#55938));
#24644=EDGE_LOOP('',(#55939,#55940,#55941,#55942));
#24645=EDGE_LOOP('',(#55943,#55944,#55945,#55946));
#30078=B_SPLINE_CURVE_WITH_KNOTS('',3,(#158211,#158212,#158213,#158214,
#158215,#158216,#158217,#158218,#158219,#158220,#158221,#158222,#158223,
#158224,#158225,#158226,#158227,#158228,#158229,#158230,#158231,#158232,
#158233,#158234,#158235,#158236,#158237,#158238,#158239,#158240,#158241,
#158242,#158243,#158244,#158245,#158246,#158247,#158248,#158249,#158250),
 .UNSPECIFIED.,.F.,.F.,(4,3,3,3,3,3,3,3,3,3,3,3,3,4),(2.84045680779053E-7,
0.0708895786428518,0.143736697789595,0.219098426622223,0.25,0.341086442232413,
0.42712793766834,0.5,0.591704542904046,0.681910213301737,0.75,0.837802729425135,
0.925712313270966,1.),.UNSPECIFIED.);
#30079=B_SPLINE_CURVE_WITH_KNOTS('',3,(#158254,#158255,#158256,#158257,
#158258,#158259,#158260,#158261,#158262,#158263,#158264,#158265,#158266,
#158267,#158268,#158269,#158270,#158271,#158272,#158273,#158274,#158275,
#158276,#158277,#158278,#158279,#158280,#158281,#158282,#158283,#158284,
#158285,#158286,#158287,#158288,#158289,#158290,#158291,#158292,#158293),
 .UNSPECIFIED.,.F.,.F.,(4,3,3,3,3,3,3,3,3,3,3,3,3,4),(1.58810254343732E-6,
0.0878641086721794,0.175637059567264,0.25,0.340009209441351,0.431407081049676,
0.5,0.585248315379607,0.675577235252377,0.75,0.82515554011605,0.898549327885159,
0.968977560346211,0.999999710276602),.UNSPECIFIED.);
#30080=B_SPLINE_CURVE_WITH_KNOTS('',3,(#158298,#158299,#158300,#158301,
#158302,#158303,#158304,#158305,#158306,#158307,#158308,#158309,#158310,
#158311,#158312,#158313,#158314,#158315,#158316),.UNSPECIFIED.,.F.,.F.,
(4,3,3,3,3,3,4),(0.,0.181023284717183,0.362342525582545,0.544428388735039,
0.727084718844238,0.910885371459506,1.),.UNSPECIFIED.);
#30081=B_SPLINE_CURVE_WITH_KNOTS('',3,(#158318,#158319,#158320,#158321,
#158322,#158323,#158324,#158325,#158326,#158327,#158328,#158329,#158330,
#158331,#158332,#158333,#158334,#158335,#158336,#158337,#158338,#158339,
#158340,#158341,#158342,#158343,#158344,#158345,#158346,#158347,#158348,
#158349,#158350,#158351,#158352,#158353,#158354,#158355,#158356,#158357,
#158358,#158359,#158360,#158361,#158362,#158363,#158364,#158365,#158366,
#158367,#158368,#158369,#158370,#158371,#158372,#158373,#158374,#158375,
#158376,#158377,#158378,#158379,#158380,#158381,#158382,#158383,#158384,
#158385,#158386,#158387,#158388,#158389,#158390,#158391,#158392,#158393,
#158394,#158395,#158396,#158397,#158398,#158399,#158400,#158401,#158402,
#158403,#158404,#158405,#158406,#158407,#158408,#158409,#158410,#158411,
#158412,#158413,#158414,#158415,#158416,#158417,#158418,#158419,#158420,
#158421,#158422,#158423,#158424,#158425,#158426,#158427),.UNSPECIFIED.,
 .F.,.F.,(4,2,2,2,2,2,1,2,2,2,2,2,2,1,2,2,2,2,1,2,2,2,2,1,1,2,2,2,2,2,1,
2,2,2,2,1,2,2,2,1,1,1,2,2,2,2,1,1,1,1,2,2,2,2,2,2,2,2,1,1,2,2,4),(0.,0.0625000000001419,
0.0937500000002126,0.125000000000283,0.187500000000425,0.21875000000049,
0.234375000000523,0.24218750000054,0.250000000000556,0.281250000000613,
0.296875000000641,0.312500000000669,0.343750000000725,0.359375000000754,
0.367187500000772,0.375000000000791,0.406250000000858,0.421875000000896,
0.429687500000909,0.43359375000091,0.437500000000912,0.46875000000088,0.484375000000864,
0.492187500000856,0.496093750000852,0.498046875000846,0.500000000000841,
0.531250000000882,0.546875000000903,0.550781250000911,0.554687500000918,
0.56250000000094,0.578125000000991,0.585937500001011,0.587890625001022,
0.589843750001033,0.593750000001075,0.60937500000126,0.617187500001356,
0.621093750001404,0.623046875001428,0.62402343750144,0.624511718751444,
0.625000000001447,0.687500000000793,0.718750000000462,0.734375000000297,
0.742187500000214,0.746093750000173,0.748046875000155,0.749023437500146,
0.750000000000137,0.781250000000108,0.796875000000098,0.804687500000092,
0.812500000000087,0.843750000000052,0.859375000000034,0.867187500000022,
0.87109375000002,0.873046875000015,0.87500000000001,1.),.UNSPECIFIED.);
#30082=B_SPLINE_CURVE_WITH_KNOTS('',3,(#158428,#158429,#158430,#158431,
#158432,#158433,#158434,#158435,#158436,#158437,#158438,#158439,#158440),
 .UNSPECIFIED.,.F.,.F.,(4,3,3,3,4),(2.68456744279971E-6,0.320124870241623,
0.652764750436627,0.752696531034302,0.999999999255413),.UNSPECIFIED.);
#30083=B_SPLINE_CURVE_WITH_KNOTS('',3,(#158444,#158445,#158446,#158447,
#158448,#158449,#158450,#158451,#158452,#158453,#158454,#158455,#158456,
#158457,#158458,#158459,#158460,#158461),.UNSPECIFIED.,.F.,.F.,(4,2,2,2,
2,2,2,2,4),(0.51322060328706,0.641524368772129,0.769828134257199,0.898134670047327,
1.02644120583745,1.15474774162758,1.28305427741771,1.41135804290278,1.53966180838785),
 .UNSPECIFIED.);
#30084=B_SPLINE_CURVE_WITH_KNOTS('',3,(#158469,#158470,#158471,#158472,
#158473,#158474,#158475,#158476,#158477,#158478,#158479,#158480,#158481,
#158482,#158483,#158484,#158485,#158486,#158487),.UNSPECIFIED.,.F.,.F.,
(4,2,2,2,3,2,2,2,4),(1.53966180838785,1.66796557393431,1.79626933948077,
1.92457587533228,2.0528824111838,2.18118894703532,2.30949548288683,2.43779924843329,
2.56610301397975),.UNSPECIFIED.);
#30085=B_SPLINE_CURVE_WITH_KNOTS('',3,(#158489,#158490,#158491,#158492,
#158493,#158494,#158495,#158496,#158497,#158498),.UNSPECIFIED.,.F.,.F.,
(4,3,3,4),(0.,0.403447226841839,0.793186801599581,1.),.UNSPECIFIED.);
#30086=B_SPLINE_CURVE_WITH_KNOTS('',3,(#158500,#158501,#158502,#158503,
#158504,#158505,#158506,#158507,#158508,#158509,#158510,#158511,#158512,
#158513,#158514,#158515,#158516,#158517,#158518,#158519,#158520,#158521,
#158522,#158523,#158524,#158525,#158526,#158527,#158528,#158529,#158530,
#158531,#158532,#158533,#158534,#158535,#158536,#158537,#158538,#158539,
#158540,#158541,#158542,#158543,#158544,#158545,#158546,#158547,#158548,
#158549,#158550,#158551,#158552,#158553,#158554,#158555,#158556,#158557,
#158558,#158559,#158560,#158561,#158562,#158563,#158564,#158565,#158566,
#158567,#158568,#158569,#158570,#158571,#158572,#158573,#158574,#158575,
#158576,#158577,#158578,#158579,#158580,#158581,#158582,#158583,#158584,
#158585,#158586,#158587,#158588,#158589,#158590,#158591,#158592,#158593,
#158594,#158595,#158596,#158597,#158598,#158599,#158600,#158601,#158602,
#158603,#158604,#158605,#158606,#158607,#158608),.UNSPECIFIED.,.F.,.F.,
(4,3,3,3,3,3,3,3,3,3,3,3,3,3,3,3,3,3,3,3,3,3,3,3,3,3,3,3,3,3,3,3,3,3,3,
3,4),(0.,0.0624999999999996,0.0937499999999992,0.109374999999997,0.123111553381916,
0.124999999999994,0.187499999999983,0.218749999999978,0.234374999999976,
0.242187499999971,0.246093749999972,0.248046874999973,0.249999999999973,
0.297621066886665,0.346682799104137,0.374999999999908,0.424324169177522,
0.437499999999879,0.468749999999865,0.484374999999863,0.492187499999863,
0.496093749999862,0.499999999999862,0.556713517041172,0.562499999999931,
0.612693929493909,0.624999999999999,0.674000499948216,0.687500000000068,
0.718750000000097,0.734375000000107,0.742187500000111,0.750000000000116,
0.815478788185251,0.878658773482917,0.939329386741458,1.),.UNSPECIFIED.);
#30087=B_SPLINE_CURVE_WITH_KNOTS('',3,(#158609,#158610,#158611,#158612,
#158613,#158614,#158615,#158616,#158617,#158618,#158619,#158620,#158621,
#158622,#158623,#158624,#158625,#158626,#158627),.UNSPECIFIED.,.F.,.F.,
(4,3,3,3,3,3,4),(9.58549878410965E-9,0.18399938603316,0.367063643664044,
0.549112471565754,0.730714957127349,0.911898041126138,1.),.UNSPECIFIED.);
#30088=B_SPLINE_CURVE_WITH_KNOTS('',3,(#158631,#158632,#158633,#158634,
#158635,#158636,#158637,#158638,#158639,#158640,#158641,#158642,#158643,
#158644,#158645,#158646),.UNSPECIFIED.,.F.,.F.,(4,3,3,3,3,4),(0.,0.232374498505923,
0.466846360420569,0.702548243138269,0.940039941077079,1.),.UNSPECIFIED.);
#30089=B_SPLINE_CURVE_WITH_KNOTS('',3,(#158648,#158649,#158650,#158651,
#158652,#158653,#158654,#158655,#158656,#158657,#158658,#158659,#158660,
#158661,#158662,#158663),.UNSPECIFIED.,.F.,.F.,(4,3,3,3,3,4),(0.,0.25,0.485488277204038,
0.719726015794557,0.952254864143456,1.),.UNSPECIFIED.);
#30090=B_SPLINE_CURVE_WITH_KNOTS('',3,(#158667,#158668,#158669,#158670,
#158671,#158672,#158673,#158674,#158675,#158676,#158677,#158678,#158679,
#158680),.UNSPECIFIED.,.F.,.F.,(4,2,2,1,1,1,1,2,4),(0.,0.232087643384168,
0.348131465076251,0.406153375922293,0.435164331345314,0.449669809056824,
0.456922547912579,0.460548917340457,0.464175286768335),.UNSPECIFIED.);
#30091=B_SPLINE_CURVE_WITH_KNOTS('',3,(#158682,#158683,#158684,#158685,
#158686,#158687,#158688,#158689,#158690,#158691,#158692,#158693,#158694,
#158695,#158696,#158697,#158698,#158699,#158700,#158701,#158702,#158703,
#158704,#158705,#158706,#158707,#158708,#158709),.UNSPECIFIED.,.F.,.F.,
(4,3,3,3,3,3,3,3,3,4),(0.464175286768335,0.507402740532681,0.575182101073047,
0.642961461613413,0.711443014313486,0.779924567013559,0.846485208441788,
0.909070904439081,0.97458738612463,1.),.UNSPECIFIED.);
#30092=B_SPLINE_CURVE_WITH_KNOTS('',3,(#158720,#158721,#158722,#158723,
#158724,#158725,#158726,#158727,#158728,#158729,#158730,#158731,#158732,
#158733,#158734,#158735,#158736,#158737),.UNSPECIFIED.,.F.,.F.,(4,2,2,2,
2,2,2,2,4),(0.51336686968484,0.64170672987966,0.77004659007448,0.89839016472208,
1.02673373936968,1.15507731401728,1.28342088866488,1.4117607488597,1.54010060905452),
 .UNSPECIFIED.);
#30093=B_SPLINE_CURVE_WITH_KNOTS('',3,(#158743,#158744,#158745,#158746,
#158747,#158748,#158749,#158750,#158751,#158752,#158753,#158754,#158755,
#158756,#158757,#158758,#158759,#158760,#158761),.UNSPECIFIED.,.F.,.F.,
(4,2,2,2,3,2,2,2,4),(-0.513366869684842,-0.385027009490022,-0.256687149295202,
-0.128343574647601,0.,0.1283435746476,0.256687149295201,0.38502700949002,
0.51336686968484),.UNSPECIFIED.);
#30094=B_SPLINE_CURVE_WITH_KNOTS('',3,(#158778,#158779,#158780,#158781,
#158782,#158783,#158784,#158785,#158786,#158787,#158788,#158789,#158790,
#158791,#158792,#158793,#158794,#158795,#158796,#158797,#158798,#158799,
#158800,#158801,#158802,#158803,#158804,#158805),.UNSPECIFIED.,.F.,.F.,
(4,3,3,3,3,3,3,3,3,4),(0.,0.0692777929336496,0.139135815966921,0.209342132953863,
0.25,0.334195898995659,0.41802748141099,0.5,0.583268776058614,0.611956694219027),
 .UNSPECIFIED.);
#30095=B_SPLINE_CURVE_WITH_KNOTS('',3,(#158807,#158808,#158809,#158810,
#158811),.UNSPECIFIED.,.F.,.F.,(4,1,4),(0.61195669421903,0.75,1.),
 .UNSPECIFIED.);
#30096=B_SPLINE_CURVE_WITH_KNOTS('',3,(#158813,#158814,#158815,#158816,
#158817,#158818,#158819,#158820,#158821,#158822,#158823,#158824,#158825,
#158826,#158827,#158828,#158829,#158830,#158831,#158832,#158833,#158834,
#158835,#158836,#158837,#158838,#158839,#158840,#158841,#158842,#158843,
#158844,#158845,#158846,#158847,#158848,#158849,#158850,#158851,#158852,
#158853,#158854,#158855,#158856,#158857,#158858,#158859,#158860,#158861),
 .UNSPECIFIED.,.F.,.F.,(4,3,3,3,3,3,3,3,3,3,3,3,3,3,3,3,4),(3.20680933356649E-11,
0.0721626588620015,0.144249523483548,0.216264815990394,0.25,0.3125,0.37457156013175,
0.437285780065875,0.5,0.566086889009772,0.632312810085566,0.698659995783495,
0.75,0.816474333249973,0.883044627621702,0.949906691452303,0.999998850808007),
 .UNSPECIFIED.);
#30097=B_SPLINE_CURVE_WITH_KNOTS('',3,(#158868,#158869,#158870,#158871,
#158872),.UNSPECIFIED.,.F.,.F.,(4,1,4),(0.,0.25,0.389921870034298),
 .UNSPECIFIED.);
#30098=B_SPLINE_CURVE_WITH_KNOTS('',3,(#158874,#158875,#158876,#158877,
#158878,#158879,#158880,#158881,#158882,#158883,#158884,#158885,#158886,
#158887,#158888,#158889,#158890,#158891,#158892,#158893,#158894,#158895,
#158896,#158897,#158898,#158899,#158900,#158901),.UNSPECIFIED.,.F.,.F.,
(4,3,3,3,3,3,3,3,3,4),(0.389921870034299,0.47318252991096,0.5,0.583741991428506,
0.667878721710084,0.75,0.820206723618715,0.890218982451227,0.959387708460516,
1.),.UNSPECIFIED.);
#30099=B_SPLINE_CURVE_WITH_KNOTS('',3,(#158906,#158907,#158908,#158909,
#158910,#158911,#158912,#158913,#158914,#158915,#158916,#158917,#158918,
#158919,#158920,#158921,#158922,#158923,#158924,#158925,#158926,#158927,
#158928,#158929,#158930,#158931,#158932,#158933,#158934,#158935,#158936,
#158937,#158938,#158939,#158940,#158941,#158942,#158943,#158944,#158945,
#158946,#158947,#158948,#158949,#158950,#158951,#158952,#158953,#158954,
#158955,#158956,#158957,#158958,#158959,#158960,#158961,#158962,#158963,
#158964,#158965,#158966,#158967,#158968,#158969,#158970,#158971,#158972,
#158973,#158974,#158975,#158976,#158977,#158978,#158979,#158980,#158981,
#158982,#158983,#158984,#158985,#158986,#158987,#158988,#158989,#158990,
#158991,#158992,#158993),.UNSPECIFIED.,.F.,.F.,(4,3,3,3,3,3,3,3,3,3,3,3,
3,3,3,3,3,3,3,3,3,3,3,3,3,3,3,3,3,4),(1.32079360702953E-6,0.0634845576880265,
0.125515787929973,0.187757893964395,0.249999999998816,0.307401094352583,
0.363909034203173,0.419246044651787,0.437499999997953,0.468749999997809,
0.484374999997749,0.492187499997707,0.496093749997697,0.499293107485499,
0.499999999997688,0.53960553479907,0.578426698983766,0.615841437993178,
0.652408482162967,0.687620805096765,0.718749999998711,0.734374999998786,
0.742609120743371,0.749999999998861,0.791313621232325,0.833775310097632,
0.87810969517575,0.923492227091124,0.970483197925126,0.999999999951529),
 .UNSPECIFIED.);
#30100=B_SPLINE_CURVE_WITH_KNOTS('',3,(#158997,#158998,#158999,#159000,
#159001,#159002,#159003,#159004,#159005,#159006,#159007,#159008,#159009,
#159010,#159011,#159012,#159013,#159014,#159015,#159016,#159017,#159018,
#159019,#159020,#159021,#159022,#159023,#159024),.UNSPECIFIED.,.F.,.F.,
(4,2,2,2,2,2,2,2,2,2,2,2,2,4),(2.81817193270301E-5,0.0404457711470591,0.0821080166266323,
0.110432701109432,0.148650946238688,0.169579357071198,0.211681646196492,
0.296346265170852,0.338302678525459,0.422553326948518,0.464657288078779,
0.549286472942467,0.61432552910643,0.676705893035455),.UNSPECIFIED.);
#30101=B_SPLINE_CURVE_WITH_KNOTS('',3,(#159028,#159029,#159030,#159031,
#159032,#159033,#159034,#159035,#159036,#159037,#159038,#159039,#159040,
#159041,#159042,#159043,#159044,#159045,#159046,#159047,#159048,#159049,
#159050,#159051,#159052,#159053,#159054,#159055),.UNSPECIFIED.,.F.,.F.,
(4,2,2,2,2,2,2,2,2,2,2,2,2,4),(2.89082885123981E-5,0.0404449424899443,0.0821047169019943,
0.110431583524439,0.148652542514045,0.169585165239432,0.211678148580102,
0.296322903616727,0.338268652222239,0.422497424572656,0.464590884909859,
0.549204383970884,0.614271515124411,0.676678486418186),.UNSPECIFIED.);
#30102=B_SPLINE_CURVE_WITH_KNOTS('',3,(#159178,#159179,#159180,#159181),
 .UNSPECIFIED.,.F.,.F.,(4,4),(6.8213951312265E-9,1.),.UNSPECIFIED.);
#30103=B_SPLINE_CURVE_WITH_KNOTS('',3,(#159182,#159183,#159184,#159185,
#159186,#159187,#159188,#159189,#159190,#159191,#159192,#159193,#159194,
#159195,#159196,#159197,#159198,#159199,#159200,#159201,#159202,#159203,
#159204,#159205,#159206,#159207,#159208,#159209,#159210,#159211,#159212,
#159213,#159214,#159215,#159216,#159217,#159218,#159219,#159220,#159221,
#159222,#159223,#159224,#159225,#159226,#159227,#159228,#159229,#159230,
#159231,#159232,#159233,#159234,#159235,#159236,#159237,#159238,#159239,
#159240,#159241,#159242,#159243,#159244,#159245,#159246,#159247,#159248,
#159249,#159250,#159251,#159252,#159253,#159254,#159255,#159256,#159257,
#159258,#159259,#159260,#159261,#159262,#159263,#159264,#159265,#159266,
#159267,#159268,#159269,#159270,#159271,#159272,#159273,#159274,#159275,
#159276,#159277,#159278),.UNSPECIFIED.,.F.,.F.,(4,3,3,3,3,3,3,3,3,3,3,3,
3,3,3,3,3,3,3,3,3,3,3,3,3,3,3,3,3,3,3,3,4),(1.50075895639123E-11,0.000238979584925606,
0.0558987779250573,0.0977547066978565,0.142061784128592,0.187141708528323,
0.20732602029247,0.249999999999667,0.299653723551624,0.335843648311373,
0.37499999999951,0.427633424273377,0.437499999999434,0.468749999999395,
0.484374999999356,0.492187499999339,0.496093749999349,0.499650467854497,
0.49999999999936,0.500176177799037,0.554344798352206,0.606121874922227,
0.61934335806653,0.670016874088742,0.719933839051705,0.742243911611287,
0.74999999999968,0.800995588371744,0.854431348938874,0.868854865545914,
0.922079159827303,0.977549834363125,1.),.UNSPECIFIED.);
#30104=B_SPLINE_CURVE_WITH_KNOTS('',3,(#159404,#159405,#159406,#159407,
#159408,#159409,#159410,#159411,#159412,#159413,#159414,#159415,#159416,
#159417,#159418,#159419,#159420,#159421,#159422,#159423),.UNSPECIFIED.,
 .F.,.F.,(4,2,2,2,2,2,2,2,2,4),(3.59015293165016E-5,0.104891984779917,0.190225981061743,
0.26444222512504,0.33832214678602,0.41214617480156,0.486142936498696,0.573670416532694,
0.630728791195145,0.686453015103136),.UNSPECIFIED.);
#30105=B_SPLINE_CURVE_WITH_KNOTS('',3,(#159488,#159489,#159490,#159491,
#159492,#159493,#159494,#159495,#159496,#159497,#159498,#159499,#159500,
#159501,#159502,#159503,#159504,#159505,#159506,#159507),.UNSPECIFIED.,
 .F.,.F.,(4,2,2,2,2,2,2,2,2,4),(3.6508494893667E-5,0.104892585500239,0.190226574989672,
0.264442813369599,0.338322729362654,0.412146751705904,0.486143507715768,
0.5736709810378,0.630729019146168,0.686453571241528),.UNSPECIFIED.);
#30106=B_SPLINE_CURVE_WITH_KNOTS('',3,(#159576,#159577,#159578,#159579,
#159580,#159581,#159582,#159583,#159584,#159585,#159586,#159587,#159588,
#159589,#159590,#159591,#159592,#159593,#159594,#159595,#159596,#159597,
#159598,#159599,#159600,#159601,#159602,#159603,#159604,#159605,#159606,
#159607,#159608,#159609,#159610,#159611,#159612,#159613,#159614,#159615,
#159616,#159617,#159618,#159619,#159620,#159621,#159622,#159623,#159624,
#159625,#159626,#159627,#159628,#159629,#159630,#159631,#159632,#159633,
#159634,#159635,#159636,#159637,#159638,#159639,#159640,#159641,#159642,
#159643,#159644,#159645,#159646,#159647,#159648,#159649,#159650,#159651,
#159652,#159653,#159654,#159655,#159656,#159657,#159658,#159659,#159660,
#159661,#159662,#159663,#159664,#159665,#159666,#159667,#159668,#159669,
#159670,#159671,#159672,#159673,#159674,#159675),.UNSPECIFIED.,.F.,.F.,
(4,3,3,3,3,3,3,3,3,3,3,3,3,3,3,3,3,3,3,3,3,3,3,3,3,3,3,3,3,3,3,3,3,4),(0.,
0.0557515009067887,0.109134396540876,0.131151604238023,0.184820483632369,
0.235915446823191,0.250000000000389,0.257780850626982,0.307754474945911,
0.358372863084605,0.375000000000583,0.380667131633151,0.432389024101429,
0.437500000000679,0.468750000000728,0.484375000000739,0.492187500000756,
0.496093750000777,0.499385919082227,0.49972917749395,0.500000000000798,
0.555330908565005,0.609768022337765,0.660505155979448,0.664205136110525,
0.713728196959825,0.750000000000399,0.792718751150899,0.837891574655351,
0.882239272625951,0.902271834341869,0.955075233491463,0.999761056440961,
0.999999999988578),.UNSPECIFIED.);
#30107=B_SPLINE_CURVE_WITH_KNOTS('',3,(#159679,#159680,#159681,#159682),
 .UNSPECIFIED.,.F.,.F.,(4,4),(0.,0.999999998785804),.UNSPECIFIED.);
#30108=B_SPLINE_CURVE_WITH_KNOTS('',3,(#159824,#159825,#159826,#159827,
#159828,#159829,#159830,#159831,#159832,#159833,#159834,#159835,#159836,
#159837,#159838,#159839,#159840,#159841,#159842,#159843,#159844,#159845),
 .UNSPECIFIED.,.F.,.F.,(4,3,3,3,3,3,3,4),(0.,0.0750543931589244,0.206343465886641,
0.353310648156244,0.51730486526382,0.695194909544737,0.877697846671489,
0.999999999887282),.UNSPECIFIED.);
#30109=B_SPLINE_CURVE_WITH_KNOTS('',3,(#159847,#159848,#159849,#159850,
#159851,#159852,#159853,#159854,#159855,#159856,#159857,#159858,#159859,
#159860,#159861,#159862,#159863,#159864,#159865,#159866,#159867,#159868),
 .UNSPECIFIED.,.F.,.F.,(4,3,3,3,3,3,3,4),(0.,0.127557126282854,0.310458518240933,
0.488256908441061,0.651827440567707,0.798268038187216,0.929115949337431,
1.),.UNSPECIFIED.);
#30110=B_SPLINE_CURVE_WITH_KNOTS('',3,(#159937,#159938,#159939,#159940,
#159941,#159942,#159943,#159944,#159945,#159946,#159947,#159948,#159949,
#159950,#159951,#159952,#159953,#159954,#159955,#159956,#159957,#159958,
#159959,#159960,#159961,#159962,#159963,#159964,#159965,#159966,#159967,
#159968,#159969,#159970,#159971,#159972,#159973,#159974,#159975,#159976,
#159977,#159978,#159979,#159980,#159981,#159982,#159983,#159984,#159985,
#159986,#159987,#159988,#159989,#159990,#159991,#159992,#159993,#159994,
#159995,#159996,#159997,#159998,#159999,#160000,#160001,#160002,#160003,
#160004,#160005,#160006,#160007,#160008,#160009,#160010,#160011,#160012,
#160013,#160014,#160015,#160016,#160017,#160018,#160019,#160020,#160021,
#160022,#160023,#160024,#160025,#160026,#160027,#160028,#160029,#160030,
#160031,#160032,#160033,#160034,#160035,#160036),.UNSPECIFIED.,.F.,.F.,
(4,3,3,3,3,3,3,3,3,3,3,3,3,3,3,3,3,3,3,3,3,3,3,3,3,3,3,3,3,3,3,3,3,4),(0.,
0.0637983485556601,0.126550304599327,0.188275152299192,0.249999999999057,
0.308956613413127,0.367063086841327,0.424032424344218,0.43749999999836,
0.468749999998245,0.484374999998192,0.492187499998172,0.496093749998165,
0.498046874998163,0.499999999998161,0.53394514537071,0.567537891023036,
0.60037914982785,0.632691384971143,0.664083874098615,0.687499999998855,
0.718749999998964,0.734374999999016,0.74218749999905,0.747353760782758,
0.749999999999083,0.785423610256769,0.821544299578016,0.858755278828813,
0.874999999999542,0.913784018887876,0.953334061394135,0.993917181375185,
0.999999999998668),.UNSPECIFIED.);
#30111=B_SPLINE_CURVE_WITH_KNOTS('',3,(#160083,#160084,#160085,#160086,
#160087,#160088,#160089,#160090,#160091,#160092,#160093,#160094,#160095,
#160096,#160097,#160098,#160099,#160100,#160101,#160102,#160103,#160104,
#160105,#160106,#160107,#160108,#160109,#160110,#160111,#160112,#160113,
#160114,#160115,#160116,#160117,#160118,#160119,#160120,#160121,#160122,
#160123,#160124,#160125,#160126,#160127,#160128,#160129,#160130,#160131,
#160132,#160133,#160134,#160135,#160136,#160137,#160138,#160139,#160140,
#160141,#160142,#160143,#160144,#160145,#160146,#160147,#160148,#160149,
#160150,#160151,#160152,#160153,#160154,#160155,#160156,#160157,#160158,
#160159,#160160,#160161,#160162,#160163,#160164,#160165,#160166,#160167,
#160168,#160169,#160170,#160171,#160172,#160173,#160174,#160175,#160176),
 .UNSPECIFIED.,.F.,.F.,(4,3,3,3,3,3,3,3,3,3,3,3,3,3,3,3,3,3,3,3,3,3,3,3,
3,3,3,3,3,3,3,4),(0.,0.0712138616603836,0.0959974304540653,0.163570456441593,
0.230073164868291,0.238936586100471,0.249999999999584,0.32929390933836,
0.374999999999386,0.376333406220443,0.437499999999286,0.468749999999227,
0.484374999999198,0.492187499999174,0.496093749999172,0.499075981956204,
0.499999999999169,0.522267304887566,0.573723493912687,0.62315099740726,
0.669708470515297,0.700946575201161,0.745077730004171,0.749999999999585,
0.791696967031908,0.832303089116417,0.838388393259743,0.878729024470567,
0.918083425162144,0.953549722072797,0.991458140984172,0.999999999987821),
 .UNSPECIFIED.);
#30112=B_SPLINE_CURVE_WITH_KNOTS('',3,(#160226,#160227,#160228,#160229,
#160230,#160231,#160232,#160233,#160234,#160235,#160236,#160237,#160238,
#160239,#160240,#160241,#160242,#160243,#160244,#160245,#160246,#160247,
#160248,#160249,#160250,#160251,#160252,#160253,#160254,#160255,#160256,
#160257,#160258,#160259,#160260,#160261,#160262,#160263,#160264,#160265,
#160266,#160267,#160268,#160269,#160270,#160271,#160272,#160273,#160274,
#160275,#160276,#160277,#160278,#160279,#160280,#160281,#160282,#160283,
#160284,#160285,#160286,#160287,#160288,#160289,#160290,#160291,#160292,
#160293,#160294,#160295,#160296,#160297,#160298,#160299,#160300,#160301,
#160302,#160303,#160304,#160305,#160306,#160307,#160308,#160309,#160310,
#160311,#160312,#160313,#160314,#160315,#160316,#160317,#160318,#160319,
#160320,#160321,#160322,#160323,#160324,#160325,#160326,#160327,#160328),
 .UNSPECIFIED.,.F.,.F.,(4,3,3,3,3,3,3,3,3,3,3,3,3,3,3,3,3,3,3,3,3,3,3,3,
3,3,3,3,3,3,3,3,3,3,4),(0.,0.029481217809345,0.0602385454853888,0.0686801150520231,
0.100978168772228,0.125000000000109,0.159373975577551,0.187500000000164,
0.194690117654056,0.200802070347523,0.203125000000173,0.218750000000182,
0.222426540538282,0.25000000000021,0.293843807324644,0.338816651531641,
0.353275723840616,0.375000000000334,0.423151004836134,0.437500000000387,
0.468750000000404,0.484375000000411,0.492187500000405,0.497285529739406,
0.500000000000398,0.507014931348073,0.584324663738214,0.644386345777789,
0.714267082163826,0.750000000000199,0.781872567237418,0.849296687796906,
0.917966672394119,0.925357651915143,0.999999999997567),.UNSPECIFIED.);
#30113=B_SPLINE_CURVE_WITH_KNOTS('',3,(#160333,#160334,#160335,#160336,
#160337,#160338,#160339,#160340,#160341,#160342,#160343,#160344,#160345,
#160346,#160347,#160348,#160349,#160350,#160351,#160352,#160353,#160354,
#160355,#160356,#160357,#160358,#160359,#160360,#160361,#160362,#160363,
#160364,#160365,#160366,#160367,#160368,#160369,#160370,#160371,#160372,
#160373,#160374,#160375,#160376,#160377,#160378,#160379,#160380,#160381,
#160382,#160383,#160384,#160385,#160386,#160387,#160388,#160389,#160390,
#160391,#160392,#160393,#160394,#160395,#160396,#160397,#160398,#160399,
#160400,#160401,#160402,#160403,#160404,#160405,#160406,#160407,#160408,
#160409,#160410,#160411,#160412,#160413,#160414,#160415,#160416,#160417,
#160418,#160419,#160420,#160421,#160422,#160423,#160424,#160425,#160426,
#160427,#160428,#160429),.UNSPECIFIED.,.F.,.F.,(4,3,3,3,3,3,3,3,3,3,3,3,
3,3,3,3,3,3,3,3,3,3,3,3,3,3,3,3,3,3,3,3,4),(5.99380613808649E-13,0.0403188271445495,
0.0798755860320985,0.118348163388507,0.125000000000114,0.162224576751813,
0.19831761361769,0.218750000000206,0.234375000000222,0.242187500000228,
0.247459770958609,0.250000000000234,0.279672982211991,0.310049892003495,
0.341912419002755,0.374007078695027,0.406978512859473,0.437500000000535,
0.468750000000584,0.484375000000598,0.492187500000601,0.496093750000596,
0.498046875000589,0.500000000000582,0.555864552409697,0.613054399144187,
0.671034612436339,0.73022202415885,0.750000000000291,0.812500000000179,
0.874695238678225,0.938574052066678,0.999999999999844),.UNSPECIFIED.);
#30114=B_SPLINE_CURVE_WITH_KNOTS('',3,(#160501,#160502,#160503,#160504,
#160505,#160506,#160507,#160508,#160509,#160510,#160511,#160512,#160513,
#160514,#160515),.UNSPECIFIED.,.F.,.F.,(4,2,2,1,1,1,2,2,4),(0.,0.249999999999863,
0.37499999999979,0.437499999999753,0.468749999999736,0.484374999999732,
0.492187499999731,0.499999999999731,1.),.UNSPECIFIED.);
#30115=B_SPLINE_CURVE_WITH_KNOTS('',3,(#160558,#160559,#160560,#160561,
#160562,#160563,#160564,#160565,#160566,#160567,#160568,#160569,#160570,
#160571,#160572,#160573,#160574,#160575,#160576,#160577,#160578,#160579,
#160580,#160581,#160582,#160583,#160584,#160585,#160586,#160587,#160588,
#160589,#160590,#160591,#160592,#160593,#160594,#160595,#160596,#160597,
#160598,#160599,#160600,#160601,#160602,#160603,#160604,#160605,#160606,
#160607,#160608,#160609,#160610,#160611,#160612,#160613,#160614,#160615,
#160616,#160617,#160618),.UNSPECIFIED.,.F.,.F.,(4,3,3,3,3,3,3,3,3,3,3,3,
3,3,3,3,3,3,3,3,4),(1.12835699204868E-7,0.0630290528050693,0.120826709348546,
0.186129648127262,0.25,0.273112941507023,0.341600487464973,0.411837351393341,
0.425308806931081,0.495917670505428,0.5,0.570579142873041,0.57752795855047,
0.647780195209018,0.716295689304132,0.72972590512184,0.75,0.816009649590574,
0.882019299181147,0.945231797138478,1.),.UNSPECIFIED.);
#30116=B_SPLINE_CURVE_WITH_KNOTS('',3,(#160647,#160648,#160649,#160650,
#160651,#160652,#160653,#160654,#160655,#160656,#160657,#160658,#160659,
#160660,#160661),.UNSPECIFIED.,.F.,.F.,(4,2,2,1,1,1,2,2,4),(0.,0.249999999999984,
0.374999999999977,0.437499999999977,0.468749999999978,0.484374999999972,
0.492187499999968,0.499999999999964,1.),.UNSPECIFIED.);
#30117=B_SPLINE_CURVE_WITH_KNOTS('',3,(#160664,#160665,#160666,#160667,
#160668,#160669,#160670,#160671,#160672,#160673),.UNSPECIFIED.,.F.,.F.,
(4,3,3,4),(0.,0.3333333333333,0.6666666666667,0.999999999699132),
 .UNSPECIFIED.);
#30118=B_SPLINE_CURVE_WITH_KNOTS('',3,(#160678,#160679,#160680,#160681,
#160682,#160683,#160684,#160685,#160686,#160687,#160688,#160689,#160690,
#160691,#160692,#160693,#160694,#160695,#160696,#160697,#160698,#160699,
#160700,#160701,#160702,#160703,#160704,#160705,#160706,#160707,#160708,
#160709,#160710,#160711,#160712,#160713,#160714,#160715,#160716,#160717,
#160718,#160719,#160720,#160721,#160722,#160723,#160724,#160725,#160726,
#160727,#160728,#160729,#160730,#160731,#160732,#160733,#160734,#160735,
#160736,#160737,#160738,#160739,#160740,#160741,#160742,#160743,#160744,
#160745,#160746,#160747,#160748,#160749,#160750,#160751,#160752,#160753,
#160754,#160755,#160756,#160757,#160758,#160759,#160760,#160761,#160762,
#160763,#160764,#160765),.UNSPECIFIED.,.F.,.F.,(4,3,3,3,3,3,3,3,3,3,3,3,
3,3,3,3,3,3,3,3,3,3,3,3,3,3,3,3,3,4),(3.0518593689493E-11,0.0861618174244873,
0.124999999999937,0.1874999999999,0.218749999999882,0.234374999999876,0.242187499999873,
0.249999999999871,0.312499999999858,0.343749999999858,0.359374999999852,
0.374999999999845,0.437499999999816,0.468749999999801,0.484374999999793,
0.492187499999794,0.499999999999796,0.56249999999989,0.593749999999938,
0.609374999999962,0.617187499999974,0.624999999999986,0.687500000000037,
0.718750000000062,0.734375000000069,0.742187500000067,0.749396528653654,
0.750000000000064,0.874999986397288,0.999999972794511),.UNSPECIFIED.);
#30119=B_SPLINE_CURVE_WITH_KNOTS('',3,(#160866,#160867,#160868,#160869,
#160870,#160871,#160872,#160873,#160874,#160875,#160876,#160877,#160878,
#160879,#160880,#160881),.UNSPECIFIED.,.F.,.F.,(4,3,3,3,3,4),(0.,0.279637227187237,
0.3333333333333,0.6666666666667,0.692929821402801,0.999995691343251),
 .UNSPECIFIED.);
#30120=B_SPLINE_CURVE_WITH_KNOTS('',3,(#160884,#160885,#160886,#160887,
#160888,#160889,#160890,#160891,#160892,#160893,#160894,#160895,#160896,
#160897,#160898,#160899,#160900,#160901,#160902,#160903,#160904,#160905,
#160906,#160907,#160908,#160909,#160910,#160911,#160912,#160913,#160914,
#160915,#160916,#160917,#160918,#160919,#160920,#160921,#160922,#160923,
#160924,#160925,#160926,#160927,#160928,#160929,#160930,#160931,#160932,
#160933,#160934,#160935,#160936,#160937,#160938,#160939,#160940,#160941,
#160942,#160943,#160944,#160945,#160946,#160947,#160948,#160949,#160950,
#160951,#160952,#160953,#160954,#160955,#160956,#160957,#160958,#160959,
#160960,#160961,#160962,#160963,#160964,#160965,#160966,#160967,#160968,
#160969,#160970,#160971,#160972,#160973,#160974,#160975,#160976,#160977),
 .UNSPECIFIED.,.F.,.F.,(4,3,3,3,3,3,3,3,3,3,3,3,3,3,3,3,3,3,3,3,3,3,3,3,
3,3,3,3,3,3,3,4),(0.,0.0625000000000142,0.0937500000000213,0.109375000000025,
0.120030834327565,0.125000000000029,0.187500000000019,0.218750000000021,
0.234375000000022,0.242187500000023,0.249602352649526,0.250000000000024,
0.312500000000072,0.343750000000095,0.359375000000101,0.367187500000099,
0.374597896383853,0.375000000000096,0.437500000000043,0.468750000000023,
0.484375000000018,0.498281689012045,0.500000000000012,0.583999870627186,
0.668503420094752,0.687500000000055,0.71875000000006,0.734375000000059,
0.750000000000058,0.836055337224158,0.922187361649025,0.999999999918209),
 .UNSPECIFIED.);
#30121=B_SPLINE_CURVE_WITH_KNOTS('',3,(#160982,#160983,#160984,#160985,
#160986,#160987,#160988,#160989,#160990,#160991,#160992,#160993,#160994,
#160995,#160996,#160997,#160998,#160999,#161000,#161001,#161002,#161003,
#161004,#161005,#161006,#161007,#161008,#161009,#161010,#161011,#161012,
#161013,#161014,#161015,#161016,#161017,#161018,#161019,#161020,#161021,
#161022,#161023,#161024,#161025,#161026,#161027,#161028,#161029,#161030,
#161031,#161032,#161033,#161034,#161035,#161036,#161037,#161038,#161039,
#161040,#161041,#161042,#161043,#161044,#161045,#161046,#161047,#161048,
#161049,#161050,#161051,#161052,#161053,#161054,#161055,#161056,#161057,
#161058,#161059,#161060,#161061,#161062,#161063,#161064,#161065,#161066,
#161067,#161068,#161069,#161070,#161071,#161072,#161073,#161074,#161075,
#161076,#161077,#161078,#161079,#161080,#161081,#161082,#161083,#161084,
#161085,#161086,#161087,#161088,#161089,#161090,#161091,#161092,#161093,
#161094,#161095,#161096,#161097,#161098,#161099,#161100,#161101,#161102,
#161103,#161104,#161105,#161106,#161107,#161108,#161109,#161110,#161111,
#161112,#161113,#161114,#161115,#161116,#161117,#161118,#161119,#161120,
#161121,#161122,#161123,#161124,#161125,#161126,#161127,#161128,#161129,
#161130,#161131,#161132,#161133,#161134,#161135,#161136,#161137,#161138,
#161139,#161140,#161141,#161142,#161143,#161144,#161145,#161146,#161147,
#161148,#161149,#161150,#161151,#161152,#161153,#161154,#161155,#161156,
#161157,#161158,#161159,#161160,#161161,#161162,#161163,#161164,#161165,
#161166,#161167,#161168,#161169,#161170,#161171,#161172,#161173,#161174,
#161175,#161176,#161177,#161178,#161179,#161180,#161181,#161182,#161183,
#161184,#161185,#161186,#161187,#161188,#161189,#161190,#161191,#161192,
#161193,#161194,#161195,#161196,#161197,#161198,#161199,#161200,#161201,
#161202,#161203,#161204,#161205,#161206,#161207,#161208,#161209,#161210,
#161211,#161212,#161213,#161214,#161215,#161216,#161217,#161218,#161219,
#161220,#161221,#161222,#161223,#161224,#161225,#161226,#161227,#161228,
#161229,#161230,#161231,#161232,#161233,#161234,#161235,#161236,#161237,
#161238,#161239,#161240,#161241,#161242,#161243,#161244,#161245,#161246,
#161247,#161248,#161249,#161250,#161251,#161252,#161253,#161254,#161255,
#161256,#161257,#161258,#161259,#161260,#161261,#161262,#161263,#161264,
#161265,#161266,#161267),.UNSPECIFIED.,.F.,.F.,(4,3,3,3,3,3,3,3,3,3,3,3,
3,3,3,3,3,3,3,3,3,3,3,3,3,3,3,3,3,3,3,3,3,3,3,3,3,3,3,3,3,3,3,3,3,3,3,3,
3,3,3,3,3,3,3,3,3,3,3,3,3,3,3,3,3,3,3,3,3,3,3,3,3,3,3,3,3,3,3,3,3,3,3,3,
3,3,3,3,3,3,3,3,3,3,3,4),(1.01228942666207E-13,0.0258517188462294,0.0291944722982846,
0.0539167902517146,0.0583388729783417,0.0819837452472311,0.0867941512072641,
0.109368785932464,0.114710180560498,0.124999999999964,0.14228679457853,
0.162838950593894,0.169724963574536,0.187499999999946,0.197102796308362,
0.215442428354756,0.218749999999937,0.224501124246269,0.234374999999933,
0.242187499999931,0.24609374999993,0.248046874999929,0.249999999999929,
0.251854256678714,0.267164879481683,0.277122765238224,0.291428278200627,
0.302730930762253,0.31600929783533,0.328978329984541,0.340881913919205,
0.35344885723419,0.35614179665251,0.367162819454531,0.374999999999932,0.384425830148499,
0.395213261190277,0.407256750918518,0.414246739447086,0.424887397515132,
0.436707838233527,0.437499999999933,0.445291520326618,0.457020760163276,
0.467982121877994,0.468749999999933,0.475797933560337,0.487960486538108,
0.499999999999934,0.505117363585142,0.518189178195458,0.531700070758596,
0.534549590305634,0.548524795152785,0.559882688873538,0.562499999999935,
0.563805319330323,0.57511664286713,0.585492659469396,0.591852345706755,
0.593749999999936,0.605206908028143,0.609374999999936,0.617187499999937,
0.619227423581006,0.621093749999937,0.623657692195749,0.624999999999937,
0.638897705866528,0.648439480043727,0.663784977517374,0.677550678837764,
0.687499999999947,0.702962444654866,0.705331409608235,0.722208861060543,
0.731604666063896,0.749999999999958,0.756846444820027,0.775981773237512,
0.78257796017835,0.802738978947917,0.80863570172481,0.829821062713248,0.834983243688876,
0.857208050362122,0.861970014046411,0.885261265678161,0.88982978307567,
0.914216652890968,0.91863289448201,0.944143940103395,0.948414026215984,
0.975074204659781,0.979491551762633,0.999999934582838),.UNSPECIFIED.);
#30122=B_SPLINE_CURVE_WITH_KNOTS('',3,(#161432,#161433,#161434,#161435,
#161436,#161437,#161438,#161439,#161440,#161441,#161442,#161443,#161444,
#161445,#161446,#161447,#161448,#161449,#161450,#161451,#161452,#161453,
#161454,#161455,#161456,#161457,#161458,#161459,#161460,#161461,#161462,
#161463,#161464,#161465,#161466,#161467,#161468,#161469,#161470,#161471,
#161472,#161473,#161474,#161475,#161476,#161477,#161478,#161479,#161480,
#161481,#161482,#161483,#161484,#161485,#161486,#161487,#161488,#161489,
#161490,#161491,#161492,#161493,#161494,#161495,#161496,#161497,#161498,
#161499,#161500,#161501,#161502,#161503,#161504,#161505,#161506,#161507,
#161508,#161509,#161510,#161511,#161512,#161513,#161514,#161515,#161516,
#161517,#161518,#161519,#161520,#161521,#161522,#161523,#161524,#161525,
#161526,#161527,#161528,#161529,#161530,#161531,#161532,#161533,#161534,
#161535,#161536,#161537,#161538,#161539,#161540,#161541,#161542,#161543,
#161544,#161545,#161546,#161547,#161548,#161549,#161550,#161551,#161552,
#161553,#161554,#161555,#161556,#161557,#161558,#161559,#161560,#161561,
#161562,#161563,#161564,#161565,#161566,#161567,#161568,#161569,#161570,
#161571,#161572,#161573,#161574,#161575,#161576,#161577,#161578,#161579,
#161580,#161581,#161582,#161583,#161584,#161585,#161586,#161587,#161588,
#161589,#161590,#161591,#161592,#161593,#161594,#161595,#161596,#161597,
#161598,#161599,#161600,#161601,#161602,#161603,#161604,#161605,#161606,
#161607,#161608,#161609,#161610,#161611,#161612,#161613,#161614,#161615,
#161616,#161617,#161618,#161619,#161620,#161621,#161622,#161623,#161624,
#161625,#161626,#161627,#161628,#161629,#161630,#161631,#161632,#161633,
#161634,#161635,#161636,#161637,#161638,#161639,#161640,#161641,#161642,
#161643,#161644,#161645,#161646,#161647,#161648,#161649,#161650,#161651,
#161652,#161653,#161654,#161655,#161656,#161657,#161658,#161659,#161660,
#161661,#161662,#161663,#161664,#161665,#161666,#161667,#161668,#161669,
#161670,#161671,#161672,#161673,#161674,#161675,#161676,#161677,#161678,
#161679,#161680,#161681,#161682,#161683,#161684,#161685,#161686,#161687,
#161688,#161689,#161690,#161691,#161692,#161693,#161694,#161695,#161696,
#161697,#161698,#161699,#161700,#161701,#161702,#161703,#161704,#161705,
#161706,#161707,#161708,#161709,#161710,#161711,#161712,#161713,#161714,
#161715,#161716,#161717,#161718,#161719,#161720,#161721,#161722,#161723,
#161724,#161725,#161726,#161727,#161728,#161729,#161730,#161731,#161732,
#161733,#161734,#161735,#161736,#161737,#161738,#161739,#161740,#161741,
#161742,#161743,#161744,#161745,#161746,#161747,#161748,#161749,#161750,
#161751,#161752,#161753,#161754,#161755,#161756,#161757,#161758,#161759,
#161760,#161761,#161762,#161763,#161764,#161765,#161766,#161767,#161768,
#161769,#161770,#161771),.UNSPECIFIED.,.F.,.F.,(4,3,3,3,3,3,3,3,3,3,3,3,
3,3,3,3,3,3,3,3,3,3,3,3,3,3,3,3,3,3,3,3,3,3,3,3,3,3,3,3,3,3,3,3,3,3,3,3,
3,3,3,3,3,3,3,3,3,3,3,3,3,3,3,3,3,3,3,3,3,3,3,3,3,3,3,3,3,3,3,3,3,3,3,3,
3,3,3,3,3,3,3,3,3,3,3,3,3,3,3,3,3,3,3,3,3,3,3,3,3,3,3,3,3,4),(0.,0.0200355867142946,
0.0273934559852642,0.02777777777778,0.0523571512332771,0.0554778740025501,
0.05555555555556,0.0780129429070063,0.08333333333333,0.0835626833505441,
0.105775578670446,0.1111111111111,0.111647540558516,0.132756838179549,0.1388888888889,
0.139731706177186,0.158229694933432,0.1666666666667,0.16781571188038,0.185503873437475,
0.1944444444444,0.195900322246756,0.212581714497131,0.2222222222222,0.223984844942246,
0.239668353537612,0.25,0.25206969643164,0.266829520339375,0.2777777777778,
0.280154959579243,0.294004855399001,0.3055555555556,0.308238363387252,0.320785848360276,
0.3333333333333,0.33631798841208,0.346836434794149,0.357823186972442,0.3611111111111,
0.364404840781021,0.374276807137445,0.384994346725833,0.3888888888889,0.392483554061635,
0.401252108118,0.410562749498785,0.4166666666667,0.420542409231562,0.427797937356122,
0.435140251960111,0.442644355403895,0.4444444444444,0.448642742632016,0.455753384099796,
0.463226096058239,0.471202663316992,0.4722222222222,0.476778765924896,0.483477707510161,
0.490325972528195,0.497204379959601,0.5,0.504840583711416,0.512744519139026,
0.520447152811956,0.5277777777778,0.532869464526171,0.540810626085051,0.548620408076424,
0.5555555555556,0.561003783620005,0.572168558476653,0.581785957831427,0.5833333333333,
0.589072583566232,0.599528783954322,0.609285938807755,0.6111111111111,0.617146865199343,
0.628017877044121,0.6388888888889,0.645234800695991,0.656989588181199,0.6666666666667,
0.673328052991939,0.687201179480869,0.6944444444444,0.701409633095276,0.716402048341608,
0.7222222222222,0.729573556853193,0.744017066992862,0.75,0.757556694920181,
0.776654469077291,0.7777777777778,0.785669915631699,0.803449019432371,0.8055555555556,
0.813769928908346,0.8333333333333,0.841844335008108,0.8611111111111,0.869925239036782,
0.8888888888889,0.898008744487289,0.9166666666667,0.926101900071302,0.9444444444444,
0.954197326598602,0.9722222222222,0.982241351582234,0.999999988745194),
 .UNSPECIFIED.);
#31123=CIRCLE('',#80381,21.5);
#31124=CIRCLE('',#80382,21.);
#31125=CIRCLE('',#80383,21.5);
#31126=CIRCLE('',#80386,21.5);
#31127=CIRCLE('',#80390,20.);
#31128=CIRCLE('',#80392,20.);
#31129=CIRCLE('',#80393,20.);
#31130=CIRCLE('',#80398,20.74940226558);
#31131=CIRCLE('',#80401,1.5);
#31132=CIRCLE('',#80402,18.49999990017);
#31133=CIRCLE('',#80404,1.367013312824);
#31134=CIRCLE('',#80405,1.50000000000001);
#31135=CIRCLE('',#80407,1.50000000000001);
#31136=CIRCLE('',#80408,1.367013312824);
#31137=CIRCLE('',#80410,2.15);
#31138=CIRCLE('',#80413,19.);
#31139=CIRCLE('',#80414,19.);
#31140=CIRCLE('',#80416,17.5);
#31141=CIRCLE('',#80418,17.5);
#31142=CIRCLE('',#80421,19.);
#31143=CIRCLE('',#80422,17.5);
#31144=CIRCLE('',#80424,19.);
#31145=CIRCLE('',#80427,17.5);
#31146=CIRCLE('',#80431,1.);
#31147=CIRCLE('',#80432,1.367013307544);
#31148=CIRCLE('',#80435,0.999999999999999);
#31149=CIRCLE('',#80436,1.367013307544);
#31150=CIRCLE('',#80439,1.50000000000001);
#31151=CIRCLE('',#80440,1.50000000000001);
#31152=CIRCLE('',#80442,1.50000000000001);
#31153=CIRCLE('',#80443,2.866767200355);
#31154=CIRCLE('',#80445,1.50000000000001);
#31155=CIRCLE('',#80447,1.50000000000001);
#31156=CIRCLE('',#80448,2.866767200355);
#31157=CIRCLE('',#80450,1.50000000000001);
#31158=CIRCLE('',#80452,1.50000000000001);
#31159=CIRCLE('',#80453,1.367013307544);
#31160=CIRCLE('',#80454,2.866767200355);
#31161=CIRCLE('',#80456,0.999999999999999);
#31162=CIRCLE('',#80459,0.6329865970941);
#31163=CIRCLE('',#80462,260.049496473139);
#31164=CIRCLE('',#80463,263.669169655306);
#31165=CIRCLE('',#80470,0.632986597024199);
#31166=CIRCLE('',#80472,1.50000000000001);
#31167=CIRCLE('',#80474,1.367013307544);
#31168=CIRCLE('',#80475,2.866767200355);
#31169=CIRCLE('',#80477,1.);
#31170=CIRCLE('',#80495,0.99994027564094);
#31171=CIRCLE('',#80496,1.00013699839423);
#31172=CIRCLE('',#80497,1.00004072258415);
#31173=CIRCLE('',#80498,2.99994768942185);
#31174=CIRCLE('',#80499,2.99994973931572);
#31175=CIRCLE('',#80501,3.00000436884464);
#31176=CIRCLE('',#80502,2.99998510560444);
#31177=CIRCLE('',#80504,0.999982594817338);
#31178=CIRCLE('',#80505,0.99999946824157);
#31179=CIRCLE('',#80506,0.999999991421499);
#31180=CIRCLE('',#80509,2.999999936398);
#31181=CIRCLE('',#80510,2.999999257509);
#31182=CIRCLE('',#80511,2.999979963362);
#31183=CIRCLE('',#80515,3.000001934398);
#31184=CIRCLE('',#80516,3.00003905154638);
#31185=CIRCLE('',#80517,2.99998878091108);
#31186=CIRCLE('',#80519,3.00001995803758);
#34493=VERTEX_POINT('',#158207);
#34494=VERTEX_POINT('',#158208);
#34495=VERTEX_POINT('',#158210);
#34496=VERTEX_POINT('',#158251);
#34497=VERTEX_POINT('',#158253);
#34498=VERTEX_POINT('',#158296);
#34499=VERTEX_POINT('',#158297);
#34500=VERTEX_POINT('',#158317);
#34501=VERTEX_POINT('',#158441);
#34502=VERTEX_POINT('',#158443);
#34503=VERTEX_POINT('',#158462);
#34504=VERTEX_POINT('',#158464);
#34505=VERTEX_POINT('',#158466);
#34506=VERTEX_POINT('',#158488);
#34507=VERTEX_POINT('',#158499);
#34508=VERTEX_POINT('',#158629);
#34509=VERTEX_POINT('',#158630);
#34510=VERTEX_POINT('',#158647);
#34511=VERTEX_POINT('',#158664);
#34512=VERTEX_POINT('',#158666);
#34513=VERTEX_POINT('',#158681);
#34514=VERTEX_POINT('',#158712);
#34515=VERTEX_POINT('',#158713);
#34516=VERTEX_POINT('',#158715);
#34517=VERTEX_POINT('',#158717);
#34518=VERTEX_POINT('',#158719);
#34519=VERTEX_POINT('',#158738);
#34520=VERTEX_POINT('',#158740);
#34521=VERTEX_POINT('',#158766);
#34522=VERTEX_POINT('',#158768);
#34523=VERTEX_POINT('',#158772);
#34524=VERTEX_POINT('',#158776);
#34525=VERTEX_POINT('',#158777);
#34526=VERTEX_POINT('',#158806);
#34527=VERTEX_POINT('',#158812);
#34528=VERTEX_POINT('',#158862);
#34529=VERTEX_POINT('',#158866);
#34530=VERTEX_POINT('',#158867);
#34531=VERTEX_POINT('',#158873);
#34532=VERTEX_POINT('',#158902);
#34533=VERTEX_POINT('',#158904);
#34534=VERTEX_POINT('',#158995);
#34535=VERTEX_POINT('',#158996);
#34536=VERTEX_POINT('',#159025);
#34537=VERTEX_POINT('',#159057);
#34538=VERTEX_POINT('',#159058);
#34539=VERTEX_POINT('',#159060);
#34540=VERTEX_POINT('',#159062);
#34541=VERTEX_POINT('',#159066);
#34542=VERTEX_POINT('',#159068);
#34543=VERTEX_POINT('',#159072);
#34544=VERTEX_POINT('',#159076);
#34545=VERTEX_POINT('',#159082);
#34546=VERTEX_POINT('',#159083);
#34547=VERTEX_POINT('',#159085);
#34548=VERTEX_POINT('',#159087);
#34549=VERTEX_POINT('',#159091);
#34550=VERTEX_POINT('',#159093);
#34551=VERTEX_POINT('',#159097);
#34552=VERTEX_POINT('',#159101);
#34553=VERTEX_POINT('',#159107);
#34554=VERTEX_POINT('',#159108);
#34555=VERTEX_POINT('',#159110);
#34556=VERTEX_POINT('',#159112);
#34557=VERTEX_POINT('',#159116);
#34558=VERTEX_POINT('',#159118);
#34559=VERTEX_POINT('',#159122);
#34560=VERTEX_POINT('',#159124);
#34561=VERTEX_POINT('',#159128);
#34562=VERTEX_POINT('',#159130);
#34563=VERTEX_POINT('',#159134);
#34564=VERTEX_POINT('',#159136);
#34565=VERTEX_POINT('',#159140);
#34566=VERTEX_POINT('',#159142);
#34567=VERTEX_POINT('',#159146);
#34568=VERTEX_POINT('',#159150);
#34569=VERTEX_POINT('',#159154);
#34570=VERTEX_POINT('',#159158);
#34571=VERTEX_POINT('',#159162);
#34572=VERTEX_POINT('',#159163);
#34573=VERTEX_POINT('',#159168);
#34574=VERTEX_POINT('',#159172);
#34575=VERTEX_POINT('',#159174);
#34576=VERTEX_POINT('',#159333);
#34577=VERTEX_POINT('',#159400);
#34578=VERTEX_POINT('',#159402);
#34579=VERTEX_POINT('',#159509);
#34580=VERTEX_POINT('',#159511);
#34581=VERTEX_POINT('',#159515);
#34582=VERTEX_POINT('',#159575);
#34583=VERTEX_POINT('',#159678);
#34584=VERTEX_POINT('',#159683);
#34585=VERTEX_POINT('',#159690);
#34586=VERTEX_POINT('',#159694);
#34587=VERTEX_POINT('',#159702);
#34588=VERTEX_POINT('',#159703);
#34589=VERTEX_POINT('',#159705);
#34590=VERTEX_POINT('',#159707);
#34591=VERTEX_POINT('',#159709);
#34592=VERTEX_POINT('',#159711);
#34593=VERTEX_POINT('',#159713);
#34594=VERTEX_POINT('',#159715);
#34595=VERTEX_POINT('',#159719);
#34596=VERTEX_POINT('',#159721);
#34597=VERTEX_POINT('',#159725);
#34598=VERTEX_POINT('',#159729);
#34599=VERTEX_POINT('',#159733);
#34600=VERTEX_POINT('',#159737);
#34601=VERTEX_POINT('',#159741);
#34602=VERTEX_POINT('',#159745);
#34603=VERTEX_POINT('',#159800);
#34604=VERTEX_POINT('',#159802);
#34605=VERTEX_POINT('',#159823);
#34606=VERTEX_POINT('',#159846);
#34607=VERTEX_POINT('',#159869);
#34608=VERTEX_POINT('',#159877);
#34609=VERTEX_POINT('',#159935);
#34610=VERTEX_POINT('',#160082);
#34611=VERTEX_POINT('',#160224);
#34612=VERTEX_POINT('',#160331);
#34613=VERTEX_POINT('',#160499);
#34614=VERTEX_POINT('',#160556);
#34615=VERTEX_POINT('',#160663);
#34616=VERTEX_POINT('',#160674);
#34617=VERTEX_POINT('',#160676);
#34618=VERTEX_POINT('',#160864);
#34619=VERTEX_POINT('',#160883);
#34620=VERTEX_POINT('',#160978);
#34621=VERTEX_POINT('',#161428);
#34622=VERTEX_POINT('',#161430);
#42594=EDGE_CURVE('',#34493,#34494,#31123,.T.);
#42595=EDGE_CURVE('',#34495,#34493,#30078,.T.);
#42596=EDGE_CURVE('',#34496,#34495,#31124,.T.);
#42597=EDGE_CURVE('',#34497,#34496,#30079,.T.);
#42598=EDGE_CURVE('',#34494,#34497,#31125,.T.);
#42599=EDGE_CURVE('',#34498,#34499,#30080,.T.);
#42600=EDGE_CURVE('',#34500,#34498,#30081,.T.);
#42601=EDGE_CURVE('',#34493,#34500,#30082,.T.);
#42602=EDGE_CURVE('',#34494,#34501,#2956,.T.);
#42603=EDGE_CURVE('',#34501,#34502,#30083,.T.);
#42604=EDGE_CURVE('',#34502,#34503,#2957,.T.);
#42605=EDGE_CURVE('',#34503,#34504,#2683,.T.);
#42606=EDGE_CURVE('',#34504,#34505,#31126,.T.);
#42607=EDGE_CURVE('',#34505,#34503,#2684,.T.);
#42608=EDGE_CURVE('',#34502,#34501,#30084,.T.);
#42609=EDGE_CURVE('',#34506,#34497,#30085,.T.);
#42610=EDGE_CURVE('',#34507,#34506,#30086,.T.);
#42611=EDGE_CURVE('',#34499,#34507,#30087,.T.);
#42612=EDGE_CURVE('',#34508,#34509,#30088,.T.);
#42613=EDGE_CURVE('',#34509,#34510,#30089,.T.);
#42614=EDGE_CURVE('',#34510,#34511,#2958,.T.);
#42615=EDGE_CURVE('',#34511,#34512,#30090,.T.);
#42616=EDGE_CURVE('',#34512,#34513,#30091,.T.);
#42617=EDGE_CURVE('',#34508,#34513,#2959,.T.);
#42618=EDGE_CURVE('',#34514,#34515,#31127,.T.);
#42619=EDGE_CURVE('',#34516,#34514,#2685,.T.);
#42620=EDGE_CURVE('',#34516,#34517,#2960,.T.);
#42621=EDGE_CURVE('',#34517,#34518,#30092,.T.);
#42622=EDGE_CURVE('',#34518,#34519,#2961,.T.);
#42623=EDGE_CURVE('',#34520,#34519,#31128,.T.);
#42624=EDGE_CURVE('',#34519,#34520,#31129,.T.);
#42625=EDGE_CURVE('',#34518,#34517,#30093,.T.);
#42626=EDGE_CURVE('',#34515,#34516,#2686,.T.);
#42627=EDGE_CURVE('',#34501,#34518,#2962,.T.);
#42628=EDGE_CURVE('',#34515,#34521,#2687,.T.);
#42629=EDGE_CURVE('',#34522,#34521,#31130,.T.);
#42630=EDGE_CURVE('',#34522,#34514,#2688,.T.);
#42631=EDGE_CURVE('',#34520,#34523,#31131,.T.);
#42632=EDGE_CURVE('',#34523,#34523,#31132,.T.);
#42633=EDGE_CURVE('',#34524,#34525,#30094,.T.);
#42634=EDGE_CURVE('',#34525,#34526,#30095,.T.);
#42635=EDGE_CURVE('',#34526,#34527,#30096,.T.);
#42636=EDGE_CURVE('',#34528,#34527,#31133,.T.);
#42637=EDGE_CURVE('',#34524,#34528,#31134,.T.);
#42638=EDGE_CURVE('',#34529,#34530,#30097,.T.);
#42639=EDGE_CURVE('',#34530,#34531,#30098,.T.);
#42640=EDGE_CURVE('',#34531,#34532,#31135,.T.);
#42641=EDGE_CURVE('',#34533,#34532,#31136,.T.);
#42642=EDGE_CURVE('',#34533,#34529,#30099,.T.);
#42643=EDGE_CURVE('',#34534,#34535,#30100,.T.);
#42644=EDGE_CURVE('',#34534,#34536,#2963,.T.);
#42645=EDGE_CURVE('',#34536,#34536,#31137,.T.);
#42646=EDGE_CURVE('',#34535,#34534,#30101,.T.);
#42647=EDGE_CURVE('',#34537,#34538,#2964,.T.);
#42648=EDGE_CURVE('',#34539,#34538,#2965,.T.);
#42649=EDGE_CURVE('',#34540,#34539,#2966,.T.);
#42650=EDGE_CURVE('',#34540,#34537,#2967,.T.);
#42651=EDGE_CURVE('',#34541,#34537,#31138,.T.);
#42652=EDGE_CURVE('',#34542,#34540,#31139,.T.);
#42653=EDGE_CURVE('',#34542,#34541,#2968,.T.);
#42654=EDGE_CURVE('',#34538,#34543,#31140,.T.);
#42655=EDGE_CURVE('',#34543,#34541,#2969,.T.);
#42656=EDGE_CURVE('',#34544,#34539,#31141,.T.);
#42657=EDGE_CURVE('',#34544,#34543,#2970,.T.);
#42658=EDGE_CURVE('',#34544,#34542,#2971,.T.);
#42659=EDGE_CURVE('',#34545,#34546,#31142,.T.);
#42660=EDGE_CURVE('',#34546,#34547,#2972,.T.);
#42661=EDGE_CURVE('',#34547,#34548,#31143,.T.);
#42662=EDGE_CURVE('',#34548,#34545,#2973,.T.);
#42663=EDGE_CURVE('',#34549,#34546,#2974,.T.);
#42664=EDGE_CURVE('',#34550,#34545,#2975,.T.);
#42665=EDGE_CURVE('',#34550,#34549,#31144,.T.);
#42666=EDGE_CURVE('',#34551,#34547,#2976,.T.);
#42667=EDGE_CURVE('',#34549,#34551,#2977,.T.);
#42668=EDGE_CURVE('',#34552,#34548,#2978,.T.);
#42669=EDGE_CURVE('',#34552,#34551,#31145,.T.);
#42670=EDGE_CURVE('',#34552,#34550,#2979,.T.);
#42671=EDGE_CURVE('',#34553,#34554,#2980,.T.);
#42672=EDGE_CURVE('',#34553,#34555,#2981,.T.);
#42673=EDGE_CURVE('',#34555,#34556,#2982,.T.);
#42674=EDGE_CURVE('',#34556,#34554,#2983,.T.);
#42675=EDGE_CURVE('',#34555,#34557,#31146,.T.);
#42676=EDGE_CURVE('',#34557,#34558,#2984,.T.);
#42677=EDGE_CURVE('',#34558,#34556,#31147,.T.);
#42678=EDGE_CURVE('',#34557,#34559,#2985,.T.);
#42679=EDGE_CURVE('',#34559,#34560,#2986,.T.);
#42680=EDGE_CURVE('',#34560,#34558,#2987,.T.);
#42681=EDGE_CURVE('',#34559,#34561,#31148,.T.);
#42682=EDGE_CURVE('',#34561,#34562,#2988,.T.);
#42683=EDGE_CURVE('',#34562,#34560,#31149,.T.);
#42684=EDGE_CURVE('',#34561,#34563,#2989,.T.);
#42685=EDGE_CURVE('',#34563,#34564,#2990,.T.);
#42686=EDGE_CURVE('',#34564,#34562,#2991,.T.);
#42687=EDGE_CURVE('',#34565,#34562,#31150,.T.);
#42688=EDGE_CURVE('',#34566,#34564,#31151,.T.);
#42689=EDGE_CURVE('',#34566,#34565,#2992,.T.);
#42690=EDGE_CURVE('',#34567,#34560,#31152,.T.);
#42691=EDGE_CURVE('',#34565,#34567,#31153,.T.);
#42692=EDGE_CURVE('',#34568,#34558,#31154,.T.);
#42693=EDGE_CURVE('',#34567,#34568,#2993,.T.);
#42694=EDGE_CURVE('',#34569,#34556,#31155,.T.);
#42695=EDGE_CURVE('',#34568,#34569,#31156,.T.);
#42696=EDGE_CURVE('',#34570,#34554,#31157,.T.);
#42697=EDGE_CURVE('',#34569,#34570,#2994,.T.);
#42698=EDGE_CURVE('',#34571,#34572,#31158,.T.);
#42699=EDGE_CURVE('',#34554,#34572,#31159,.T.);
#42700=EDGE_CURVE('',#34570,#34571,#31160,.T.);
#42701=EDGE_CURVE('',#34573,#34572,#2995,.T.);
#42702=EDGE_CURVE('',#34573,#34553,#31161,.T.);
#42703=EDGE_CURVE('',#34572,#34574,#2996,.T.);
#42704=EDGE_CURVE('',#34574,#34575,#2997,.T.);
#42705=EDGE_CURVE('',#34575,#34573,#2998,.T.);
#42706=EDGE_CURVE('',#34571,#34529,#30102,.T.);
#42707=EDGE_CURVE('',#34529,#34574,#30103,.T.);
#42708=EDGE_CURVE('',#34533,#34574,#31162,.T.);
#42709=EDGE_CURVE('',#34533,#34576,#2999,.T.);
#42710=EDGE_CURVE('',#34576,#34575,#2689,.T.);
#42711=EDGE_CURVE('',#34534,#34577,#31163,.T.);
#42712=EDGE_CURVE('',#34535,#34578,#31164,.T.);
#42713=EDGE_CURVE('',#34577,#34578,#30104,.T.);
#42714=EDGE_CURVE('',#34578,#34577,#30105,.T.);
#42715=EDGE_CURVE('',#34579,#34528,#3000,.T.);
#42716=EDGE_CURVE('',#34527,#34580,#3001,.T.);
#42717=EDGE_CURVE('',#34580,#34579,#2690,.T.);
#42718=EDGE_CURVE('',#34581,#34532,#3002,.T.);
#42719=EDGE_CURVE('',#34532,#34528,#3003,.T.);
#42720=EDGE_CURVE('',#34579,#34581,#3004,.T.);
#42721=EDGE_CURVE('',#34581,#34576,#2691,.T.);
#42722=EDGE_CURVE('',#34531,#34524,#3005,.T.);
#42723=EDGE_CURVE('',#34582,#34526,#30106,.T.);
#42724=EDGE_CURVE('',#34582,#34527,#31165,.T.);
#42725=EDGE_CURVE('',#34526,#34583,#30107,.T.);
#42726=EDGE_CURVE('',#34583,#34584,#31166,.T.);
#42727=EDGE_CURVE('',#34582,#34584,#3006,.T.);
#42728=EDGE_CURVE('',#34584,#34564,#31167,.T.);
#42729=EDGE_CURVE('',#34583,#34566,#31168,.T.);
#42730=EDGE_CURVE('',#34563,#34585,#31169,.T.);
#42731=EDGE_CURVE('',#34585,#34584,#3007,.T.);
#42732=EDGE_CURVE('',#34582,#34586,#3008,.T.);
#42733=EDGE_CURVE('',#34585,#34586,#3009,.T.);
#42734=EDGE_CURVE('',#34586,#34580,#2692,.T.);
#42735=EDGE_CURVE('',#34586,#34575,#3010,.T.);
#42736=EDGE_CURVE('',#34587,#34588,#3011,.T.);
#42737=EDGE_CURVE('',#34589,#34587,#3012,.T.);
#42738=EDGE_CURVE('',#34590,#34589,#3013,.T.);
#42739=EDGE_CURVE('',#34591,#34590,#3014,.T.);
#42740=EDGE_CURVE('',#34592,#34591,#3015,.T.);
#42741=EDGE_CURVE('',#34593,#34592,#3016,.T.);
#42742=EDGE_CURVE('',#34594,#34593,#3017,.T.);
#42743=EDGE_CURVE('',#34588,#34594,#3018,.T.);
#42744=EDGE_CURVE('',#34587,#34595,#3019,.T.);
#42745=EDGE_CURVE('',#34588,#34596,#3020,.T.);
#42746=EDGE_CURVE('',#34596,#34595,#3021,.T.);
#42747=EDGE_CURVE('',#34589,#34597,#3022,.T.);
#42748=EDGE_CURVE('',#34595,#34597,#3023,.T.);
#42749=EDGE_CURVE('',#34590,#34598,#3024,.T.);
#42750=EDGE_CURVE('',#34597,#34598,#3025,.T.);
#42751=EDGE_CURVE('',#34591,#34599,#3026,.T.);
#42752=EDGE_CURVE('',#34598,#34599,#3027,.T.);
#42753=EDGE_CURVE('',#34592,#34600,#3028,.T.);
#42754=EDGE_CURVE('',#34599,#34600,#3029,.T.);
#42755=EDGE_CURVE('',#34593,#34601,#3030,.T.);
#42756=EDGE_CURVE('',#34600,#34601,#3031,.T.);
#42757=EDGE_CURVE('',#34594,#34602,#3032,.T.);
#42758=EDGE_CURVE('',#34601,#34602,#3033,.T.);
#42759=EDGE_CURVE('',#34602,#34596,#3034,.T.);
#42760=EDGE_CURVE('',#34522,#34504,#3035,.T.);
#42761=EDGE_CURVE('',#34505,#34521,#3036,.T.);
#42762=EDGE_CURVE('',#34511,#34603,#31170,.T.);
#42763=EDGE_CURVE('',#34603,#34604,#1766,.T.);
#42764=EDGE_CURVE('',#34513,#34604,#31171,.T.);
#42765=EDGE_CURVE('',#34604,#34605,#30108,.T.);
#42766=EDGE_CURVE('',#34606,#34603,#30109,.T.);
#42767=EDGE_CURVE('',#34607,#34606,#1767,.T.);
#42768=EDGE_CURVE('',#34608,#34607,#1768,.T.);
#42769=EDGE_CURVE('',#34605,#34608,#1769,.T.);
#42770=EDGE_CURVE('',#34609,#34605,#31172,.T.);
#42771=EDGE_CURVE('',#34513,#34609,#30110,.T.);
#42772=EDGE_CURVE('',#34498,#34508,#31173,.T.);
#42773=EDGE_CURVE('',#34610,#34508,#30111,.T.);
#42774=EDGE_CURVE('',#34500,#34610,#31174,.T.);
#42775=EDGE_CURVE('',#34610,#34609,#3037,.T.);
#42776=EDGE_CURVE('',#34506,#34611,#31175,.T.);
#42777=EDGE_CURVE('',#34510,#34611,#30112,.T.);
#42778=EDGE_CURVE('',#34507,#34510,#31176,.T.);
#42779=EDGE_CURVE('',#34611,#34612,#3038,.T.);
#42780=EDGE_CURVE('',#34612,#34511,#30113,.T.);
#42781=EDGE_CURVE('',#34612,#34606,#31177,.T.);
#42782=EDGE_CURVE('',#34613,#34607,#31178,.T.);
#42783=EDGE_CURVE('',#34613,#34612,#30114,.T.);
#42784=EDGE_CURVE('',#34614,#34608,#31179,.T.);
#42785=EDGE_CURVE('',#34614,#34613,#30115,.T.);
#42786=EDGE_CURVE('',#34609,#34614,#30116,.T.);
#42787=EDGE_CURVE('',#34615,#34610,#30117,.T.);
#42788=EDGE_CURVE('',#34616,#34614,#3039,.T.);
#42789=EDGE_CURVE('',#34616,#34617,#2693,.T.);
#42790=EDGE_CURVE('',#34617,#34615,#30118,.T.);
#42791=EDGE_CURVE('',#34493,#34615,#31180,.T.);
#42792=EDGE_CURVE('',#34499,#34509,#31181,.T.);
#42793=EDGE_CURVE('',#34497,#34618,#31182,.T.);
#42794=EDGE_CURVE('',#34611,#34618,#30119,.T.);
#42795=EDGE_CURVE('',#34618,#34619,#30120,.T.);
#42796=EDGE_CURVE('',#34619,#34620,#2694,.T.);
#42797=EDGE_CURVE('',#34620,#34613,#3040,.T.);
#42798=EDGE_CURVE('',#34620,#34616,#30121,.T.);
#42799=EDGE_CURVE('',#34621,#34616,#31183,.T.);
#42800=EDGE_CURVE('',#34622,#34620,#31184,.T.);
#42801=EDGE_CURVE('',#34622,#34621,#30122,.T.);
#42802=EDGE_CURVE('',#34495,#34617,#31185,.T.);
#42803=EDGE_CURVE('',#34621,#34495,#2695,.T.);
#42804=EDGE_CURVE('',#34496,#34619,#31186,.T.);
#42805=EDGE_CURVE('',#34496,#34622,#2696,.T.);
#55523=ORIENTED_EDGE('',*,*,#42594,.F.);
#55524=ORIENTED_EDGE('',*,*,#42595,.F.);
#55525=ORIENTED_EDGE('',*,*,#42596,.F.);
#55526=ORIENTED_EDGE('',*,*,#42597,.F.);
#55527=ORIENTED_EDGE('',*,*,#42598,.F.);
#55528=ORIENTED_EDGE('',*,*,#42599,.F.);
#55529=ORIENTED_EDGE('',*,*,#42600,.F.);
#55530=ORIENTED_EDGE('',*,*,#42601,.F.);
#55531=ORIENTED_EDGE('',*,*,#42594,.T.);
#55532=ORIENTED_EDGE('',*,*,#42602,.T.);
#55533=ORIENTED_EDGE('',*,*,#42603,.T.);
#55534=ORIENTED_EDGE('',*,*,#42604,.T.);
#55535=ORIENTED_EDGE('',*,*,#42605,.T.);
#55536=ORIENTED_EDGE('',*,*,#42606,.T.);
#55537=ORIENTED_EDGE('',*,*,#42607,.T.);
#55538=ORIENTED_EDGE('',*,*,#42604,.F.);
#55539=ORIENTED_EDGE('',*,*,#42608,.T.);
#55540=ORIENTED_EDGE('',*,*,#42602,.F.);
#55541=ORIENTED_EDGE('',*,*,#42598,.T.);
#55542=ORIENTED_EDGE('',*,*,#42609,.F.);
#55543=ORIENTED_EDGE('',*,*,#42610,.F.);
#55544=ORIENTED_EDGE('',*,*,#42611,.F.);
#55545=ORIENTED_EDGE('',*,*,#42612,.T.);
#55546=ORIENTED_EDGE('',*,*,#42613,.T.);
#55547=ORIENTED_EDGE('',*,*,#42614,.T.);
#55548=ORIENTED_EDGE('',*,*,#42615,.T.);
#55549=ORIENTED_EDGE('',*,*,#42616,.T.);
#55550=ORIENTED_EDGE('',*,*,#42617,.F.);
#55551=ORIENTED_EDGE('',*,*,#42618,.F.);
#55552=ORIENTED_EDGE('',*,*,#42619,.F.);
#55553=ORIENTED_EDGE('',*,*,#42620,.T.);
#55554=ORIENTED_EDGE('',*,*,#42621,.T.);
#55555=ORIENTED_EDGE('',*,*,#42622,.T.);
#55556=ORIENTED_EDGE('',*,*,#42623,.F.);
#55557=ORIENTED_EDGE('',*,*,#42624,.F.);
#55558=ORIENTED_EDGE('',*,*,#42622,.F.);
#55559=ORIENTED_EDGE('',*,*,#42625,.T.);
#55560=ORIENTED_EDGE('',*,*,#42620,.F.);
#55561=ORIENTED_EDGE('',*,*,#42626,.F.);
#55562=ORIENTED_EDGE('',*,*,#42603,.F.);
#55563=ORIENTED_EDGE('',*,*,#42627,.T.);
#55564=ORIENTED_EDGE('',*,*,#42621,.F.);
#55565=ORIENTED_EDGE('',*,*,#42625,.F.);
#55566=ORIENTED_EDGE('',*,*,#42627,.F.);
#55567=ORIENTED_EDGE('',*,*,#42608,.F.);
#55568=ORIENTED_EDGE('',*,*,#42618,.T.);
#55569=ORIENTED_EDGE('',*,*,#42628,.T.);
#55570=ORIENTED_EDGE('',*,*,#42629,.F.);
#55571=ORIENTED_EDGE('',*,*,#42630,.T.);
#55572=ORIENTED_EDGE('',*,*,#42623,.T.);
#55573=ORIENTED_EDGE('',*,*,#42624,.T.);
#55574=ORIENTED_EDGE('',*,*,#42631,.T.);
#55575=ORIENTED_EDGE('',*,*,#42632,.F.);
#55576=ORIENTED_EDGE('',*,*,#42631,.F.);
#55577=ORIENTED_EDGE('',*,*,#42633,.T.);
#55578=ORIENTED_EDGE('',*,*,#42634,.T.);
#55579=ORIENTED_EDGE('',*,*,#42635,.T.);
#55580=ORIENTED_EDGE('',*,*,#42636,.F.);
#55581=ORIENTED_EDGE('',*,*,#42637,.F.);
#55582=ORIENTED_EDGE('',*,*,#42638,.T.);
#55583=ORIENTED_EDGE('',*,*,#42639,.T.);
#55584=ORIENTED_EDGE('',*,*,#42640,.T.);
#55585=ORIENTED_EDGE('',*,*,#42641,.F.);
#55586=ORIENTED_EDGE('',*,*,#42642,.T.);
#55587=ORIENTED_EDGE('',*,*,#42643,.F.);
#55588=ORIENTED_EDGE('',*,*,#42644,.T.);
#55589=ORIENTED_EDGE('',*,*,#42645,.T.);
#55590=ORIENTED_EDGE('',*,*,#42644,.F.);
#55591=ORIENTED_EDGE('',*,*,#42646,.F.);
#55592=ORIENTED_EDGE('',*,*,#42647,.T.);
#55593=ORIENTED_EDGE('',*,*,#42648,.F.);
#55594=ORIENTED_EDGE('',*,*,#42649,.F.);
#55595=ORIENTED_EDGE('',*,*,#42650,.T.);
#55596=ORIENTED_EDGE('',*,*,#42651,.T.);
#55597=ORIENTED_EDGE('',*,*,#42650,.F.);
#55598=ORIENTED_EDGE('',*,*,#42652,.F.);
#55599=ORIENTED_EDGE('',*,*,#42653,.T.);
#55600=ORIENTED_EDGE('',*,*,#42654,.F.);
#55601=ORIENTED_EDGE('',*,*,#42647,.F.);
#55602=ORIENTED_EDGE('',*,*,#42651,.F.);
#55603=ORIENTED_EDGE('',*,*,#42655,.F.);
#55604=ORIENTED_EDGE('',*,*,#42656,.T.);
#55605=ORIENTED_EDGE('',*,*,#42648,.T.);
#55606=ORIENTED_EDGE('',*,*,#42654,.T.);
#55607=ORIENTED_EDGE('',*,*,#42657,.F.);
#55608=ORIENTED_EDGE('',*,*,#42655,.T.);
#55609=ORIENTED_EDGE('',*,*,#42653,.F.);
#55610=ORIENTED_EDGE('',*,*,#42658,.F.);
#55611=ORIENTED_EDGE('',*,*,#42657,.T.);
#55612=ORIENTED_EDGE('',*,*,#42659,.T.);
#55613=ORIENTED_EDGE('',*,*,#42660,.T.);
#55614=ORIENTED_EDGE('',*,*,#42661,.T.);
#55615=ORIENTED_EDGE('',*,*,#42662,.T.);
#55616=ORIENTED_EDGE('',*,*,#42663,.T.);
#55617=ORIENTED_EDGE('',*,*,#42659,.F.);
#55618=ORIENTED_EDGE('',*,*,#42664,.F.);
#55619=ORIENTED_EDGE('',*,*,#42665,.T.);
#55620=ORIENTED_EDGE('',*,*,#42666,.T.);
#55621=ORIENTED_EDGE('',*,*,#42660,.F.);
#55622=ORIENTED_EDGE('',*,*,#42663,.F.);
#55623=ORIENTED_EDGE('',*,*,#42667,.T.);
#55624=ORIENTED_EDGE('',*,*,#42668,.T.);
#55625=ORIENTED_EDGE('',*,*,#42661,.F.);
#55626=ORIENTED_EDGE('',*,*,#42666,.F.);
#55627=ORIENTED_EDGE('',*,*,#42669,.F.);
#55628=ORIENTED_EDGE('',*,*,#42664,.T.);
#55629=ORIENTED_EDGE('',*,*,#42662,.F.);
#55630=ORIENTED_EDGE('',*,*,#42668,.F.);
#55631=ORIENTED_EDGE('',*,*,#42670,.T.);
#55632=ORIENTED_EDGE('',*,*,#42671,.F.);
#55633=ORIENTED_EDGE('',*,*,#42672,.T.);
#55634=ORIENTED_EDGE('',*,*,#42673,.T.);
#55635=ORIENTED_EDGE('',*,*,#42674,.T.);
#55636=ORIENTED_EDGE('',*,*,#42673,.F.);
#55637=ORIENTED_EDGE('',*,*,#42675,.T.);
#55638=ORIENTED_EDGE('',*,*,#42676,.T.);
#55639=ORIENTED_EDGE('',*,*,#42677,.T.);
#55640=ORIENTED_EDGE('',*,*,#42676,.F.);
#55641=ORIENTED_EDGE('',*,*,#42678,.T.);
#55642=ORIENTED_EDGE('',*,*,#42679,.T.);
#55643=ORIENTED_EDGE('',*,*,#42680,.T.);
#55644=ORIENTED_EDGE('',*,*,#42679,.F.);
#55645=ORIENTED_EDGE('',*,*,#42681,.T.);
#55646=ORIENTED_EDGE('',*,*,#42682,.T.);
#55647=ORIENTED_EDGE('',*,*,#42683,.T.);
#55648=ORIENTED_EDGE('',*,*,#42682,.F.);
#55649=ORIENTED_EDGE('',*,*,#42684,.T.);
#55650=ORIENTED_EDGE('',*,*,#42685,.T.);
#55651=ORIENTED_EDGE('',*,*,#42686,.T.);
#55652=ORIENTED_EDGE('',*,*,#42687,.T.);
#55653=ORIENTED_EDGE('',*,*,#42686,.F.);
#55654=ORIENTED_EDGE('',*,*,#42688,.F.);
#55655=ORIENTED_EDGE('',*,*,#42689,.T.);
#55656=ORIENTED_EDGE('',*,*,#42690,.T.);
#55657=ORIENTED_EDGE('',*,*,#42683,.F.);
#55658=ORIENTED_EDGE('',*,*,#42687,.F.);
#55659=ORIENTED_EDGE('',*,*,#42691,.T.);
#55660=ORIENTED_EDGE('',*,*,#42692,.T.);
#55661=ORIENTED_EDGE('',*,*,#42680,.F.);
#55662=ORIENTED_EDGE('',*,*,#42690,.F.);
#55663=ORIENTED_EDGE('',*,*,#42693,.T.);
#55664=ORIENTED_EDGE('',*,*,#42694,.T.);
#55665=ORIENTED_EDGE('',*,*,#42677,.F.);
#55666=ORIENTED_EDGE('',*,*,#42692,.F.);
#55667=ORIENTED_EDGE('',*,*,#42695,.T.);
#55668=ORIENTED_EDGE('',*,*,#42696,.T.);
#55669=ORIENTED_EDGE('',*,*,#42674,.F.);
#55670=ORIENTED_EDGE('',*,*,#42694,.F.);
#55671=ORIENTED_EDGE('',*,*,#42697,.T.);
#55672=ORIENTED_EDGE('',*,*,#42698,.T.);
#55673=ORIENTED_EDGE('',*,*,#42699,.F.);
#55674=ORIENTED_EDGE('',*,*,#42696,.F.);
#55675=ORIENTED_EDGE('',*,*,#42700,.T.);
#55676=ORIENTED_EDGE('',*,*,#42701,.F.);
#55677=ORIENTED_EDGE('',*,*,#42702,.T.);
#55678=ORIENTED_EDGE('',*,*,#42671,.T.);
#55679=ORIENTED_EDGE('',*,*,#42699,.T.);
#55680=ORIENTED_EDGE('',*,*,#42701,.T.);
#55681=ORIENTED_EDGE('',*,*,#42703,.T.);
#55682=ORIENTED_EDGE('',*,*,#42704,.T.);
#55683=ORIENTED_EDGE('',*,*,#42705,.T.);
#55684=ORIENTED_EDGE('',*,*,#42698,.F.);
#55685=ORIENTED_EDGE('',*,*,#42706,.T.);
#55686=ORIENTED_EDGE('',*,*,#42707,.T.);
#55687=ORIENTED_EDGE('',*,*,#42703,.F.);
#55688=ORIENTED_EDGE('',*,*,#42707,.F.);
#55689=ORIENTED_EDGE('',*,*,#42642,.F.);
#55690=ORIENTED_EDGE('',*,*,#42708,.T.);
#55691=ORIENTED_EDGE('',*,*,#42704,.F.);
#55692=ORIENTED_EDGE('',*,*,#42708,.F.);
#55693=ORIENTED_EDGE('',*,*,#42709,.T.);
#55694=ORIENTED_EDGE('',*,*,#42710,.T.);
#55695=ORIENTED_EDGE('',*,*,#42711,.F.);
#55696=ORIENTED_EDGE('',*,*,#42643,.T.);
#55697=ORIENTED_EDGE('',*,*,#42712,.T.);
#55698=ORIENTED_EDGE('',*,*,#42713,.F.);
#55699=ORIENTED_EDGE('',*,*,#42712,.F.);
#55700=ORIENTED_EDGE('',*,*,#42646,.T.);
#55701=ORIENTED_EDGE('',*,*,#42711,.T.);
#55702=ORIENTED_EDGE('',*,*,#42714,.F.);
#55703=ORIENTED_EDGE('',*,*,#42715,.T.);
#55704=ORIENTED_EDGE('',*,*,#42636,.T.);
#55705=ORIENTED_EDGE('',*,*,#42716,.T.);
#55706=ORIENTED_EDGE('',*,*,#42717,.T.);
#55707=ORIENTED_EDGE('',*,*,#42718,.T.);
#55708=ORIENTED_EDGE('',*,*,#42719,.T.);
#55709=ORIENTED_EDGE('',*,*,#42715,.F.);
#55710=ORIENTED_EDGE('',*,*,#42720,.T.);
#55711=ORIENTED_EDGE('',*,*,#42713,.T.);
#55712=ORIENTED_EDGE('',*,*,#42714,.T.);
#55713=ORIENTED_EDGE('',*,*,#42709,.F.);
#55714=ORIENTED_EDGE('',*,*,#42641,.T.);
#55715=ORIENTED_EDGE('',*,*,#42718,.F.);
#55716=ORIENTED_EDGE('',*,*,#42721,.T.);
#55717=ORIENTED_EDGE('',*,*,#42637,.T.);
#55718=ORIENTED_EDGE('',*,*,#42719,.F.);
#55719=ORIENTED_EDGE('',*,*,#42640,.F.);
#55720=ORIENTED_EDGE('',*,*,#42722,.T.);
#55721=ORIENTED_EDGE('',*,*,#42635,.F.);
#55722=ORIENTED_EDGE('',*,*,#42723,.F.);
#55723=ORIENTED_EDGE('',*,*,#42724,.T.);
#55724=ORIENTED_EDGE('',*,*,#42723,.T.);
#55725=ORIENTED_EDGE('',*,*,#42725,.T.);
#55726=ORIENTED_EDGE('',*,*,#42726,.T.);
#55727=ORIENTED_EDGE('',*,*,#42727,.F.);
#55728=ORIENTED_EDGE('',*,*,#42688,.T.);
#55729=ORIENTED_EDGE('',*,*,#42728,.F.);
#55730=ORIENTED_EDGE('',*,*,#42726,.F.);
#55731=ORIENTED_EDGE('',*,*,#42729,.T.);
#55732=ORIENTED_EDGE('',*,*,#42685,.F.);
#55733=ORIENTED_EDGE('',*,*,#42730,.T.);
#55734=ORIENTED_EDGE('',*,*,#42731,.T.);
#55735=ORIENTED_EDGE('',*,*,#42728,.T.);
#55736=ORIENTED_EDGE('',*,*,#42732,.F.);
#55737=ORIENTED_EDGE('',*,*,#42727,.T.);
#55738=ORIENTED_EDGE('',*,*,#42731,.F.);
#55739=ORIENTED_EDGE('',*,*,#42733,.T.);
#55740=ORIENTED_EDGE('',*,*,#42716,.F.);
#55741=ORIENTED_EDGE('',*,*,#42724,.F.);
#55742=ORIENTED_EDGE('',*,*,#42732,.T.);
#55743=ORIENTED_EDGE('',*,*,#42734,.T.);
#55744=ORIENTED_EDGE('',*,*,#42735,.T.);
#55745=ORIENTED_EDGE('',*,*,#42710,.F.);
#55746=ORIENTED_EDGE('',*,*,#42721,.F.);
#55747=ORIENTED_EDGE('',*,*,#42720,.F.);
#55748=ORIENTED_EDGE('',*,*,#42717,.F.);
#55749=ORIENTED_EDGE('',*,*,#42734,.F.);
#55750=ORIENTED_EDGE('',*,*,#42733,.F.);
#55751=ORIENTED_EDGE('',*,*,#42730,.F.);
#55752=ORIENTED_EDGE('',*,*,#42684,.F.);
#55753=ORIENTED_EDGE('',*,*,#42681,.F.);
#55754=ORIENTED_EDGE('',*,*,#42678,.F.);
#55755=ORIENTED_EDGE('',*,*,#42675,.F.);
#55756=ORIENTED_EDGE('',*,*,#42672,.F.);
#55757=ORIENTED_EDGE('',*,*,#42702,.F.);
#55758=ORIENTED_EDGE('',*,*,#42705,.F.);
#55759=ORIENTED_EDGE('',*,*,#42735,.F.);
#55760=ORIENTED_EDGE('',*,*,#42736,.F.);
#55761=ORIENTED_EDGE('',*,*,#42737,.F.);
#55762=ORIENTED_EDGE('',*,*,#42738,.F.);
#55763=ORIENTED_EDGE('',*,*,#42739,.F.);
#55764=ORIENTED_EDGE('',*,*,#42740,.F.);
#55765=ORIENTED_EDGE('',*,*,#42741,.F.);
#55766=ORIENTED_EDGE('',*,*,#42742,.F.);
#55767=ORIENTED_EDGE('',*,*,#42743,.F.);
#55768=ORIENTED_EDGE('',*,*,#42744,.F.);
#55769=ORIENTED_EDGE('',*,*,#42736,.T.);
#55770=ORIENTED_EDGE('',*,*,#42745,.T.);
#55771=ORIENTED_EDGE('',*,*,#42746,.T.);
#55772=ORIENTED_EDGE('',*,*,#42747,.F.);
#55773=ORIENTED_EDGE('',*,*,#42737,.T.);
#55774=ORIENTED_EDGE('',*,*,#42744,.T.);
#55775=ORIENTED_EDGE('',*,*,#42748,.T.);
#55776=ORIENTED_EDGE('',*,*,#42749,.F.);
#55777=ORIENTED_EDGE('',*,*,#42738,.T.);
#55778=ORIENTED_EDGE('',*,*,#42747,.T.);
#55779=ORIENTED_EDGE('',*,*,#42750,.T.);
#55780=ORIENTED_EDGE('',*,*,#42751,.F.);
#55781=ORIENTED_EDGE('',*,*,#42739,.T.);
#55782=ORIENTED_EDGE('',*,*,#42749,.T.);
#55783=ORIENTED_EDGE('',*,*,#42752,.T.);
#55784=ORIENTED_EDGE('',*,*,#42753,.F.);
#55785=ORIENTED_EDGE('',*,*,#42740,.T.);
#55786=ORIENTED_EDGE('',*,*,#42751,.T.);
#55787=ORIENTED_EDGE('',*,*,#42754,.T.);
#55788=ORIENTED_EDGE('',*,*,#42645,.F.);
#55789=ORIENTED_EDGE('',*,*,#42755,.F.);
#55790=ORIENTED_EDGE('',*,*,#42741,.T.);
#55791=ORIENTED_EDGE('',*,*,#42753,.T.);
#55792=ORIENTED_EDGE('',*,*,#42756,.T.);
#55793=ORIENTED_EDGE('',*,*,#42757,.F.);
#55794=ORIENTED_EDGE('',*,*,#42742,.T.);
#55795=ORIENTED_EDGE('',*,*,#42755,.T.);
#55796=ORIENTED_EDGE('',*,*,#42758,.T.);
#55797=ORIENTED_EDGE('',*,*,#42745,.F.);
#55798=ORIENTED_EDGE('',*,*,#42743,.T.);
#55799=ORIENTED_EDGE('',*,*,#42757,.T.);
#55800=ORIENTED_EDGE('',*,*,#42759,.T.);
#55801=ORIENTED_EDGE('',*,*,#42632,.T.);
#55802=ORIENTED_EDGE('',*,*,#42697,.F.);
#55803=ORIENTED_EDGE('',*,*,#42695,.F.);
#55804=ORIENTED_EDGE('',*,*,#42693,.F.);
#55805=ORIENTED_EDGE('',*,*,#42691,.F.);
#55806=ORIENTED_EDGE('',*,*,#42689,.F.);
#55807=ORIENTED_EDGE('',*,*,#42729,.F.);
#55808=ORIENTED_EDGE('',*,*,#42725,.F.);
#55809=ORIENTED_EDGE('',*,*,#42634,.F.);
#55810=ORIENTED_EDGE('',*,*,#42633,.F.);
#55811=ORIENTED_EDGE('',*,*,#42722,.F.);
#55812=ORIENTED_EDGE('',*,*,#42639,.F.);
#55813=ORIENTED_EDGE('',*,*,#42638,.F.);
#55814=ORIENTED_EDGE('',*,*,#42706,.F.);
#55815=ORIENTED_EDGE('',*,*,#42700,.F.);
#55816=ORIENTED_EDGE('',*,*,#42758,.F.);
#55817=ORIENTED_EDGE('',*,*,#42756,.F.);
#55818=ORIENTED_EDGE('',*,*,#42754,.F.);
#55819=ORIENTED_EDGE('',*,*,#42752,.F.);
#55820=ORIENTED_EDGE('',*,*,#42750,.F.);
#55821=ORIENTED_EDGE('',*,*,#42748,.F.);
#55822=ORIENTED_EDGE('',*,*,#42746,.F.);
#55823=ORIENTED_EDGE('',*,*,#42759,.F.);
#55824=ORIENTED_EDGE('',*,*,#42626,.T.);
#55825=ORIENTED_EDGE('',*,*,#42619,.T.);
#55826=ORIENTED_EDGE('',*,*,#42630,.F.);
#55827=ORIENTED_EDGE('',*,*,#42760,.T.);
#55828=ORIENTED_EDGE('',*,*,#42605,.F.);
#55829=ORIENTED_EDGE('',*,*,#42607,.F.);
#55830=ORIENTED_EDGE('',*,*,#42761,.T.);
#55831=ORIENTED_EDGE('',*,*,#42628,.F.);
#55832=ORIENTED_EDGE('',*,*,#42606,.F.);
#55833=ORIENTED_EDGE('',*,*,#42760,.F.);
#55834=ORIENTED_EDGE('',*,*,#42629,.T.);
#55835=ORIENTED_EDGE('',*,*,#42761,.F.);
#55836=ORIENTED_EDGE('',*,*,#42762,.T.);
#55837=ORIENTED_EDGE('',*,*,#42763,.T.);
#55838=ORIENTED_EDGE('',*,*,#42764,.F.);
#55839=ORIENTED_EDGE('',*,*,#42616,.F.);
#55840=ORIENTED_EDGE('',*,*,#42615,.F.);
#55841=ORIENTED_EDGE('',*,*,#42765,.F.);
#55842=ORIENTED_EDGE('',*,*,#42763,.F.);
#55843=ORIENTED_EDGE('',*,*,#42766,.F.);
#55844=ORIENTED_EDGE('',*,*,#42767,.F.);
#55845=ORIENTED_EDGE('',*,*,#42768,.F.);
#55846=ORIENTED_EDGE('',*,*,#42769,.F.);
#55847=ORIENTED_EDGE('',*,*,#42764,.T.);
#55848=ORIENTED_EDGE('',*,*,#42765,.T.);
#55849=ORIENTED_EDGE('',*,*,#42770,.F.);
#55850=ORIENTED_EDGE('',*,*,#42771,.F.);
#55851=ORIENTED_EDGE('',*,*,#42772,.T.);
#55852=ORIENTED_EDGE('',*,*,#42773,.F.);
#55853=ORIENTED_EDGE('',*,*,#42774,.F.);
#55854=ORIENTED_EDGE('',*,*,#42600,.T.);
#55855=ORIENTED_EDGE('',*,*,#42617,.T.);
#55856=ORIENTED_EDGE('',*,*,#42771,.T.);
#55857=ORIENTED_EDGE('',*,*,#42775,.F.);
#55858=ORIENTED_EDGE('',*,*,#42773,.T.);
#55859=ORIENTED_EDGE('',*,*,#42776,.T.);
#55860=ORIENTED_EDGE('',*,*,#42777,.F.);
#55861=ORIENTED_EDGE('',*,*,#42778,.F.);
#55862=ORIENTED_EDGE('',*,*,#42610,.T.);
#55863=ORIENTED_EDGE('',*,*,#42779,.T.);
#55864=ORIENTED_EDGE('',*,*,#42780,.T.);
#55865=ORIENTED_EDGE('',*,*,#42614,.F.);
#55866=ORIENTED_EDGE('',*,*,#42777,.T.);
#55867=ORIENTED_EDGE('',*,*,#42781,.T.);
#55868=ORIENTED_EDGE('',*,*,#42766,.T.);
#55869=ORIENTED_EDGE('',*,*,#42762,.F.);
#55870=ORIENTED_EDGE('',*,*,#42780,.F.);
#55871=ORIENTED_EDGE('',*,*,#42782,.T.);
#55872=ORIENTED_EDGE('',*,*,#42767,.T.);
#55873=ORIENTED_EDGE('',*,*,#42781,.F.);
#55874=ORIENTED_EDGE('',*,*,#42783,.F.);
#55875=ORIENTED_EDGE('',*,*,#42784,.T.);
#55876=ORIENTED_EDGE('',*,*,#42768,.T.);
#55877=ORIENTED_EDGE('',*,*,#42782,.F.);
#55878=ORIENTED_EDGE('',*,*,#42785,.F.);
#55879=ORIENTED_EDGE('',*,*,#42770,.T.);
#55880=ORIENTED_EDGE('',*,*,#42769,.T.);
#55881=ORIENTED_EDGE('',*,*,#42784,.F.);
#55882=ORIENTED_EDGE('',*,*,#42786,.F.);
#55883=ORIENTED_EDGE('',*,*,#42787,.T.);
#55884=ORIENTED_EDGE('',*,*,#42775,.T.);
#55885=ORIENTED_EDGE('',*,*,#42786,.T.);
#55886=ORIENTED_EDGE('',*,*,#42788,.F.);
#55887=ORIENTED_EDGE('',*,*,#42789,.T.);
#55888=ORIENTED_EDGE('',*,*,#42790,.T.);
#55889=ORIENTED_EDGE('',*,*,#42774,.T.);
#55890=ORIENTED_EDGE('',*,*,#42787,.F.);
#55891=ORIENTED_EDGE('',*,*,#42791,.F.);
#55892=ORIENTED_EDGE('',*,*,#42601,.T.);
#55893=ORIENTED_EDGE('',*,*,#42792,.T.);
#55894=ORIENTED_EDGE('',*,*,#42612,.F.);
#55895=ORIENTED_EDGE('',*,*,#42772,.F.);
#55896=ORIENTED_EDGE('',*,*,#42599,.T.);
#55897=ORIENTED_EDGE('',*,*,#42778,.T.);
#55898=ORIENTED_EDGE('',*,*,#42613,.F.);
#55899=ORIENTED_EDGE('',*,*,#42792,.F.);
#55900=ORIENTED_EDGE('',*,*,#42611,.T.);
#55901=ORIENTED_EDGE('',*,*,#42793,.T.);
#55902=ORIENTED_EDGE('',*,*,#42794,.F.);
#55903=ORIENTED_EDGE('',*,*,#42776,.F.);
#55904=ORIENTED_EDGE('',*,*,#42609,.T.);
#55905=ORIENTED_EDGE('',*,*,#42795,.T.);
#55906=ORIENTED_EDGE('',*,*,#42796,.T.);
#55907=ORIENTED_EDGE('',*,*,#42797,.T.);
#55908=ORIENTED_EDGE('',*,*,#42783,.T.);
#55909=ORIENTED_EDGE('',*,*,#42779,.F.);
#55910=ORIENTED_EDGE('',*,*,#42794,.T.);
#55911=ORIENTED_EDGE('',*,*,#42788,.T.);
#55912=ORIENTED_EDGE('',*,*,#42785,.T.);
#55913=ORIENTED_EDGE('',*,*,#42797,.F.);
#55914=ORIENTED_EDGE('',*,*,#42798,.T.);
#55915=ORIENTED_EDGE('',*,*,#42799,.T.);
#55916=ORIENTED_EDGE('',*,*,#42798,.F.);
#55917=ORIENTED_EDGE('',*,*,#42800,.F.);
#55918=ORIENTED_EDGE('',*,*,#42801,.T.);
#55919=ORIENTED_EDGE('',*,*,#42802,.T.);
#55920=ORIENTED_EDGE('',*,*,#42789,.F.);
#55921=ORIENTED_EDGE('',*,*,#42799,.F.);
#55922=ORIENTED_EDGE('',*,*,#42803,.T.);
#55923=ORIENTED_EDGE('',*,*,#42791,.T.);
#55924=ORIENTED_EDGE('',*,*,#42790,.F.);
#55925=ORIENTED_EDGE('',*,*,#42802,.F.);
#55926=ORIENTED_EDGE('',*,*,#42595,.T.);
#55927=ORIENTED_EDGE('',*,*,#42804,.T.);
#55928=ORIENTED_EDGE('',*,*,#42795,.F.);
#55929=ORIENTED_EDGE('',*,*,#42793,.F.);
#55930=ORIENTED_EDGE('',*,*,#42597,.T.);
#55931=ORIENTED_EDGE('',*,*,#42800,.T.);
#55932=ORIENTED_EDGE('',*,*,#42796,.F.);
#55933=ORIENTED_EDGE('',*,*,#42804,.F.);
#55934=ORIENTED_EDGE('',*,*,#42805,.T.);
#55935=ORIENTED_EDGE('',*,*,#42596,.T.);
#55936=ORIENTED_EDGE('',*,*,#42803,.F.);
#55937=ORIENTED_EDGE('',*,*,#42801,.F.);
#55938=ORIENTED_EDGE('',*,*,#42805,.F.);
#55939=ORIENTED_EDGE('',*,*,#42652,.T.);
#55940=ORIENTED_EDGE('',*,*,#42649,.T.);
#55941=ORIENTED_EDGE('',*,*,#42656,.F.);
#55942=ORIENTED_EDGE('',*,*,#42658,.T.);
#55943=ORIENTED_EDGE('',*,*,#42669,.T.);
#55944=ORIENTED_EDGE('',*,*,#42667,.F.);
#55945=ORIENTED_EDGE('',*,*,#42665,.F.);
#55946=ORIENTED_EDGE('',*,*,#42670,.F.);
#75945=ADVANCED_FACE('',(#20515),#1878,.T.);
#75946=ADVANCED_FACE('',(#20516),#2150,.T.);
#75947=ADVANCED_FACE('',(#20517),#2151,.T.);
#75948=ADVANCED_FACE('',(#20518),#2152,.F.);
#75949=ADVANCED_FACE('',(#20519),#2153,.F.);
#75950=ADVANCED_FACE('',(#20520),#1924,.F.);
#75951=ADVANCED_FACE('',(#20521),#1879,.F.);
#75952=ADVANCED_FACE('',(#20522),#1880,.F.);
#75953=ADVANCED_FACE('',(#20523),#1881,.F.);
#75954=ADVANCED_FACE('',(#20524),#2154,.F.);
#75955=ADVANCED_FACE('',(#20525),#16916,.F.);
#75956=ADVANCED_FACE('',(#20526),#2155,.T.);
#75957=ADVANCED_FACE('',(#20527),#16917,.F.);
#75958=ADVANCED_FACE('',(#20528),#2156,.F.);
#75959=ADVANCED_FACE('',(#20529),#16918,.F.);
#75960=ADVANCED_FACE('',(#20530),#16919,.T.);
#75961=ADVANCED_FACE('',(#20531),#2157,.T.);
#75962=ADVANCED_FACE('',(#20532),#16920,.T.);
#75963=ADVANCED_FACE('',(#20533),#2158,.F.);
#75964=ADVANCED_FACE('',(#20534),#16921,.T.);
#75965=ADVANCED_FACE('',(#20535),#16922,.T.);
#75966=ADVANCED_FACE('',(#20536),#1925,.T.);
#75967=ADVANCED_FACE('',(#20537),#16923,.T.);
#75968=ADVANCED_FACE('',(#20538),#1926,.T.);
#75969=ADVANCED_FACE('',(#20539),#16924,.T.);
#75970=ADVANCED_FACE('',(#20540),#2159,.F.);
#75971=ADVANCED_FACE('',(#20541),#1882,.F.);
#75972=ADVANCED_FACE('',(#20542),#2160,.F.);
#75973=ADVANCED_FACE('',(#20543),#1883,.F.);
#75974=ADVANCED_FACE('',(#20544),#2161,.F.);
#75975=ADVANCED_FACE('',(#20545),#1884,.F.);
#75976=ADVANCED_FACE('',(#20546),#1927,.T.);
#75977=ADVANCED_FACE('',(#20547),#16925,.T.);
#75978=ADVANCED_FACE('',(#20548),#2162,.F.);
#75979=ADVANCED_FACE('',(#20549),#2615,.F.);
#75980=ADVANCED_FACE('',(#20550),#1928,.F.);
#75981=ADVANCED_FACE('',(#20551),#176,.F.);
#75982=ADVANCED_FACE('',(#20552),#177,.F.);
#75983=ADVANCED_FACE('',(#20553),#1929,.T.);
#75984=ADVANCED_FACE('',(#20554,#269),#16926,.T.);
#75985=ADVANCED_FACE('',(#20555),#1930,.T.);
#75986=ADVANCED_FACE('',(#20556),#2163,.F.);
#75987=ADVANCED_FACE('',(#20557),#2616,.F.);
#75988=ADVANCED_FACE('',(#20558),#2164,.F.);
#75989=ADVANCED_FACE('',(#20559),#1885,.F.);
#75990=ADVANCED_FACE('',(#20560),#1931,.T.);
#75991=ADVANCED_FACE('',(#20561),#16927,.T.);
#75992=ADVANCED_FACE('',(#20562),#1932,.F.);
#75993=ADVANCED_FACE('',(#20563),#16928,.F.);
#75994=ADVANCED_FACE('',(#20564,#270),#16929,.T.);
#75995=ADVANCED_FACE('',(#20565),#16930,.T.);
#75996=ADVANCED_FACE('',(#20566),#16931,.T.);
#75997=ADVANCED_FACE('',(#20567),#16932,.T.);
#75998=ADVANCED_FACE('',(#20568),#16933,.T.);
#75999=ADVANCED_FACE('',(#20569,#271),#16934,.T.);
#76000=ADVANCED_FACE('',(#20570),#16935,.T.);
#76001=ADVANCED_FACE('',(#20571),#16936,.T.);
#76002=ADVANCED_FACE('',(#20572),#16937,.T.);
#76003=ADVANCED_FACE('',(#20573,#272),#16938,.F.);
#76004=ADVANCED_FACE('',(#20574),#16939,.F.);
#76005=ADVANCED_FACE('',(#20575),#16940,.F.);
#76006=ADVANCED_FACE('',(#20576),#16941,.F.);
#76007=ADVANCED_FACE('',(#20577),#2617,.T.);
#76008=ADVANCED_FACE('',(#20578),#178,.F.);
#76009=ADVANCED_FACE('',(#20579),#2618,.T.);
#76010=ADVANCED_FACE('',(#20580),#2619,.F.);
#76011=ADVANCED_FACE('',(#20581),#2165,.T.);
#76012=ADVANCED_FACE('',(#20582),#2620,.F.);
#76013=ADVANCED_FACE('',(#20583),#2166,.T.);
#76014=ADVANCED_FACE('',(#20584),#2621,.T.);
#76015=ADVANCED_FACE('',(#20585),#2622,.T.);
#76016=ADVANCED_FACE('',(#20586),#2623,.T.);
#76017=ADVANCED_FACE('',(#20587),#2624,.T.);
#76018=ADVANCED_FACE('',(#20588),#2167,.T.);
#76019=ADVANCED_FACE('',(#20589),#2625,.F.);
#76020=ADVANCED_FACE('',(#20590),#2626,.F.);
#76021=ADVANCED_FACE('',(#20591),#2627,.F.);
#76022=ADVANCED_FACE('',(#20592),#2628,.F.);
#76023=ADVANCED_FACE('',(#20593),#2168,.T.);
#76024=ADVANCED_FACE('',(#20594),#2169,.T.);
#76025=ADVANCED_FACE('',(#20595),#2629,.F.);
#76026=ADVANCED_FACE('',(#20596),#2630,.F.);
#76027=ADVANCED_FACE('',(#20597),#2631,.F.);
#76028=ADVANCED_FACE('',(#20598),#2632,.F.);
#76029=ADVANCED_FACE('',(#20599),#2633,.F.);
#76030=ADVANCED_FACE('',(#20600,#273,#274),#16942,.T.);
#79323=CLOSED_SHELL('',(#75945,#75946,#75947,#75948,#75949,#75950,#75951,
#75952,#75953,#75954,#75955,#75956,#75957,#75958,#75959,#75960,#75961,#75962,
#75963,#75964,#75965,#75966,#75967,#75968,#75969,#75970,#75971,#75972,#75973,
#75974,#75975,#75976,#75977,#75978,#75979,#75980,#75981,#75982,#75983,#75984,
#75985,#75986,#75987,#75988,#75989,#75990,#75991,#75992,#75993,#75994,#75995,
#75996,#75997,#75998,#75999,#76000,#76001,#76002,#76003,#76004,#76005,#76006,
#76007,#76008,#76009,#76010,#76011,#76012,#76013,#76014,#76015,#76016,#76017,
#76018,#76019,#76020,#76021,#76022,#76023,#76024,#76025,#76026,#76027,#76028,
#76029,#76030));
#80379=AXIS2_PLACEMENT_3D('',#158205,#88213,#88214);
#80380=AXIS2_PLACEMENT_3D('',#158206,#88215,#88216);
#80381=AXIS2_PLACEMENT_3D('',#158209,#88217,#88218);
#80382=AXIS2_PLACEMENT_3D('',#158252,#88219,#88220);
#80383=AXIS2_PLACEMENT_3D('',#158294,#88221,#88222);
#80384=AXIS2_PLACEMENT_3D('',#158295,#88223,#88224);
#80385=AXIS2_PLACEMENT_3D('',#158465,#88227,#88228);
#80386=AXIS2_PLACEMENT_3D('',#158467,#88229,#88230);
#80387=AXIS2_PLACEMENT_3D('',#158468,#88231,#88232);
#80388=AXIS2_PLACEMENT_3D('',#158628,#88233,#88234);
#80389=AXIS2_PLACEMENT_3D('',#158711,#88237,#88238);
#80390=AXIS2_PLACEMENT_3D('',#158714,#88239,#88240);
#80391=AXIS2_PLACEMENT_3D('',#158716,#88241,#88242);
#80392=AXIS2_PLACEMENT_3D('',#158741,#88245,#88246);
#80393=AXIS2_PLACEMENT_3D('',#158742,#88247,#88248);
#80394=AXIS2_PLACEMENT_3D('',#158762,#88249,#88250);
#80395=AXIS2_PLACEMENT_3D('',#158763,#88251,#88252);
#80396=AXIS2_PLACEMENT_3D('',#158765,#88254,#88255);
#80397=AXIS2_PLACEMENT_3D('',#158767,#88256,#88257);
#80398=AXIS2_PLACEMENT_3D('',#158769,#88258,#88259);
#80399=AXIS2_PLACEMENT_3D('',#158770,#88260,#88261);
#80400=AXIS2_PLACEMENT_3D('',#158771,#88262,#88263);
#80401=AXIS2_PLACEMENT_3D('',#158773,#88264,#88265);
#80402=AXIS2_PLACEMENT_3D('',#158774,#88266,#88267);
#80403=AXIS2_PLACEMENT_3D('',#158775,#88268,#88269);
#80404=AXIS2_PLACEMENT_3D('',#158863,#88270,#88271);
#80405=AXIS2_PLACEMENT_3D('',#158864,#88272,#88273);
#80406=AXIS2_PLACEMENT_3D('',#158865,#88274,#88275);
#80407=AXIS2_PLACEMENT_3D('',#158903,#88276,#88277);
#80408=AXIS2_PLACEMENT_3D('',#158905,#88278,#88279);
#80409=AXIS2_PLACEMENT_3D('',#158994,#88280,#88281);
#80410=AXIS2_PLACEMENT_3D('',#159027,#88283,#88284);
#80411=AXIS2_PLACEMENT_3D('',#159056,#88285,#88286);
#80412=AXIS2_PLACEMENT_3D('',#159065,#88291,#88292);
#80413=AXIS2_PLACEMENT_3D('',#159067,#88293,#88294);
#80414=AXIS2_PLACEMENT_3D('',#159069,#88295,#88296);
#80415=AXIS2_PLACEMENT_3D('',#159071,#88298,#88299);
#80416=AXIS2_PLACEMENT_3D('',#159073,#88300,#88301);
#80417=AXIS2_PLACEMENT_3D('',#159075,#88303,#88304);
#80418=AXIS2_PLACEMENT_3D('',#159077,#88305,#88306);
#80419=AXIS2_PLACEMENT_3D('',#159079,#88308,#88309);
#80420=AXIS2_PLACEMENT_3D('',#159081,#88311,#88312);
#80421=AXIS2_PLACEMENT_3D('',#159084,#88313,#88314);
#80422=AXIS2_PLACEMENT_3D('',#159088,#88316,#88317);
#80423=AXIS2_PLACEMENT_3D('',#159090,#88319,#88320);
#80424=AXIS2_PLACEMENT_3D('',#159095,#88323,#88324);
#80425=AXIS2_PLACEMENT_3D('',#159096,#88325,#88326);
#80426=AXIS2_PLACEMENT_3D('',#159100,#88329,#88330);
#80427=AXIS2_PLACEMENT_3D('',#159103,#88332,#88333);
#80428=AXIS2_PLACEMENT_3D('',#159104,#88334,#88335);
#80429=AXIS2_PLACEMENT_3D('',#159106,#88337,#88338);
#80430=AXIS2_PLACEMENT_3D('',#159115,#88343,#88344);
#80431=AXIS2_PLACEMENT_3D('',#159117,#88345,#88346);
#80432=AXIS2_PLACEMENT_3D('',#159120,#88348,#88349);
#80433=AXIS2_PLACEMENT_3D('',#159121,#88350,#88351);
#80434=AXIS2_PLACEMENT_3D('',#159127,#88355,#88356);
#80435=AXIS2_PLACEMENT_3D('',#159129,#88357,#88358);
#80436=AXIS2_PLACEMENT_3D('',#159132,#88360,#88361);
#80437=AXIS2_PLACEMENT_3D('',#159133,#88362,#88363);
#80438=AXIS2_PLACEMENT_3D('',#159139,#88367,#88368);
#80439=AXIS2_PLACEMENT_3D('',#159141,#88369,#88370);
#80440=AXIS2_PLACEMENT_3D('',#159143,#88371,#88372);
#80441=AXIS2_PLACEMENT_3D('',#159145,#88374,#88375);
#80442=AXIS2_PLACEMENT_3D('',#159147,#88376,#88377);
#80443=AXIS2_PLACEMENT_3D('',#159148,#88378,#88379);
#80444=AXIS2_PLACEMENT_3D('',#159149,#88380,#88381);
#80445=AXIS2_PLACEMENT_3D('',#159151,#88382,#88383);
#80446=AXIS2_PLACEMENT_3D('',#159153,#88385,#88386);
#80447=AXIS2_PLACEMENT_3D('',#159155,#88387,#88388);
#80448=AXIS2_PLACEMENT_3D('',#159156,#88389,#88390);
#80449=AXIS2_PLACEMENT_3D('',#159157,#88391,#88392);
#80450=AXIS2_PLACEMENT_3D('',#159159,#88393,#88394);
#80451=AXIS2_PLACEMENT_3D('',#159161,#88396,#88397);
#80452=AXIS2_PLACEMENT_3D('',#159164,#88398,#88399);
#80453=AXIS2_PLACEMENT_3D('',#159165,#88400,#88401);
#80454=AXIS2_PLACEMENT_3D('',#159166,#88402,#88403);
#80455=AXIS2_PLACEMENT_3D('',#159167,#88404,#88405);
#80456=AXIS2_PLACEMENT_3D('',#159170,#88407,#88408);
#80457=AXIS2_PLACEMENT_3D('',#159171,#88409,#88410);
#80458=AXIS2_PLACEMENT_3D('',#159177,#88414,#88415);
#80459=AXIS2_PLACEMENT_3D('',#159331,#88416,#88417);
#80460=AXIS2_PLACEMENT_3D('',#159332,#88418,#88419);
#80461=AXIS2_PLACEMENT_3D('',#159335,#88421,#88422);
#80462=AXIS2_PLACEMENT_3D('',#159401,#88423,#88424);
#80463=AXIS2_PLACEMENT_3D('',#159403,#88425,#88426);
#80464=AXIS2_PLACEMENT_3D('',#159508,#88427,#88428);
#80465=AXIS2_PLACEMENT_3D('',#159513,#88431,#88432);
#80466=AXIS2_PLACEMENT_3D('',#159514,#88433,#88434);
#80467=AXIS2_PLACEMENT_3D('',#159519,#88438,#88439);
#80468=AXIS2_PLACEMENT_3D('',#159520,#88440,#88441);
#80469=AXIS2_PLACEMENT_3D('',#159521,#88442,#88443);
#80470=AXIS2_PLACEMENT_3D('',#159676,#88445,#88446);
#80471=AXIS2_PLACEMENT_3D('',#159677,#88447,#88448);
#80472=AXIS2_PLACEMENT_3D('',#159684,#88449,#88450);
#80473=AXIS2_PLACEMENT_3D('',#159686,#88452,#88453);
#80474=AXIS2_PLACEMENT_3D('',#159687,#88454,#88455);
#80475=AXIS2_PLACEMENT_3D('',#159688,#88456,#88457);
#80476=AXIS2_PLACEMENT_3D('',#159689,#88458,#88459);
#80477=AXIS2_PLACEMENT_3D('',#159691,#88460,#88461);
#80478=AXIS2_PLACEMENT_3D('',#159693,#88463,#88464);
#80479=AXIS2_PLACEMENT_3D('',#159697,#88467,#88468);
#80480=AXIS2_PLACEMENT_3D('',#159698,#88469,#88470);
#80481=AXIS2_PLACEMENT_3D('',#159699,#88471,#88472);
#80482=AXIS2_PLACEMENT_3D('',#159701,#88474,#88475);
#80483=AXIS2_PLACEMENT_3D('',#159718,#88484,#88485);
#80484=AXIS2_PLACEMENT_3D('',#159724,#88489,#88490);
#80485=AXIS2_PLACEMENT_3D('',#159728,#88493,#88494);
#80486=AXIS2_PLACEMENT_3D('',#159732,#88497,#88498);
#80487=AXIS2_PLACEMENT_3D('',#159736,#88501,#88502);
#80488=AXIS2_PLACEMENT_3D('',#159740,#88505,#88506);
#80489=AXIS2_PLACEMENT_3D('',#159744,#88509,#88510);
#80490=AXIS2_PLACEMENT_3D('',#159748,#88513,#88514);
#80491=AXIS2_PLACEMENT_3D('',#159750,#88516,#88517);
#80492=AXIS2_PLACEMENT_3D('',#159751,#88518,#88519);
#80493=AXIS2_PLACEMENT_3D('',#159752,#88520,#88521);
#80494=AXIS2_PLACEMENT_3D('',#159755,#88524,#88525);
#80495=AXIS2_PLACEMENT_3D('',#159801,#88526,#88527);
#80496=AXIS2_PLACEMENT_3D('',#159814,#88528,#88529);
#80497=AXIS2_PLACEMENT_3D('',#159936,#88530,#88531);
#80498=AXIS2_PLACEMENT_3D('',#160081,#88532,#88533);
#80499=AXIS2_PLACEMENT_3D('',#160177,#88534,#88535);
#80500=AXIS2_PLACEMENT_3D('',#160178,#88536,#88537);
#80501=AXIS2_PLACEMENT_3D('',#160225,#88539,#88540);
#80502=AXIS2_PLACEMENT_3D('',#160329,#88541,#88542);
#80503=AXIS2_PLACEMENT_3D('',#160330,#88543,#88544);
#80504=AXIS2_PLACEMENT_3D('',#160470,#88546,#88547);
#80505=AXIS2_PLACEMENT_3D('',#160500,#88548,#88549);
#80506=AXIS2_PLACEMENT_3D('',#160557,#88550,#88551);
#80507=AXIS2_PLACEMENT_3D('',#160662,#88552,#88553);
#80508=AXIS2_PLACEMENT_3D('',#160677,#88555,#88556);
#80509=AXIS2_PLACEMENT_3D('',#160790,#88557,#88558);
#80510=AXIS2_PLACEMENT_3D('',#160815,#88559,#88560);
#80511=AXIS2_PLACEMENT_3D('',#160865,#88561,#88562);
#80512=AXIS2_PLACEMENT_3D('',#160882,#88563,#88564);
#80513=AXIS2_PLACEMENT_3D('',#160979,#88565,#88566);
#80514=AXIS2_PLACEMENT_3D('',#160981,#88568,#88569);
#80515=AXIS2_PLACEMENT_3D('',#161429,#88570,#88571);
#80516=AXIS2_PLACEMENT_3D('',#161431,#88572,#88573);
#80517=AXIS2_PLACEMENT_3D('',#161796,#88574,#88575);
#80518=AXIS2_PLACEMENT_3D('',#161797,#88576,#88577);
#80519=AXIS2_PLACEMENT_3D('',#161910,#88578,#88579);
#80520=AXIS2_PLACEMENT_3D('',#161935,#88580,#88581);
#80521=AXIS2_PLACEMENT_3D('',#161936,#88582,#88583);
#88213=DIRECTION('axis',(0.,0.,1.));
#88214=DIRECTION('refdir',(1.,0.,0.));
#88215=DIRECTION('center_axis',(0.173648177666903,-6.04203006598724E-18,
0.984807753012213));
#88216=DIRECTION('ref_axis',(-0.984756463038268,-0.0102058657879588,0.173639133860657));
#88217=DIRECTION('center_axis',(-0.173648177666902,-4.61141851223429E-16,
-0.984807753012213));
#88218=DIRECTION('ref_axis',(0.927511157342012,-0.336119036715289,-0.163545241947503));
#88219=DIRECTION('center_axis',(0.173648177666903,-1.85288922023609E-16,
0.984807753012213));
#88220=DIRECTION('ref_axis',(0.942703464213078,0.289274509623319,-0.166224055548075));
#88221=DIRECTION('center_axis',(-0.173648177666902,-4.61141851223429E-16,
-0.984807753012213));
#88222=DIRECTION('ref_axis',(0.927511157342012,-0.336119036715289,-0.163545241947503));
#88223=DIRECTION('center_axis',(0.173648177666902,-1.50111279695127E-18,
0.984807753012213));
#88224=DIRECTION('ref_axis',(0.984806496090504,0.00159769267247521,-0.173647956037692));
#88225=DIRECTION('',(-0.173648177666902,1.50111279695126E-18,-0.984807753012213));
#88226=DIRECTION('',(-0.173648177666902,1.50111279695126E-18,-0.984807753012213));
#88227=DIRECTION('center_axis',(0.529918793382048,0.000598506209364813,
0.848048179180187));
#88228=DIRECTION('ref_axis',(0.848046930758909,0.00148135485041045,-0.529919058742183));
#88229=DIRECTION('center_axis',(0.173648177666902,-1.50111279695127E-18,
0.984807753012213));
#88230=DIRECTION('ref_axis',(0.984806496090504,0.00159769267247521,-0.173647956037692));
#88231=DIRECTION('center_axis',(0.529918793382048,0.000598506209364813,
0.848048179180187));
#88232=DIRECTION('ref_axis',(0.848046930758909,0.00148135485041045,-0.529919058742183));
#88233=DIRECTION('center_axis',(0.999998762173495,0.00157342029648582,2.18262210013749E-7));
#88234=DIRECTION('ref_axis',(-2.18262210388419E-7,0.000277436450264717,
-0.999999961514483));
#88235=DIRECTION('',(0.999998760211623,0.00157466659798374,5.66973100805864E-7));
#88236=DIRECTION('',(0.999998761676006,0.00157373645740291,1.29989624092794E-7));
#88237=DIRECTION('center_axis',(0.173648177666902,-1.49186218934005E-18,
0.984807753012213));
#88238=DIRECTION('ref_axis',(0.984806496090504,0.00159769267247521,-0.173647956037692));
#88239=DIRECTION('center_axis',(0.173648177666902,-1.49186218934005E-18,
0.984807753012213));
#88240=DIRECTION('ref_axis',(0.984806496090504,0.00159769267247533,-0.173647956037692));
#88241=DIRECTION('center_axis',(0.529918793382083,0.000598506209369939,
0.848048179180166));
#88242=DIRECTION('ref_axis',(0.848046930758885,0.00148135485220636,-0.529919058742217));
#88243=DIRECTION('',(0.173648177666902,-1.49186218934005E-18,0.984807753012213));
#88244=DIRECTION('',(0.173648177666902,-1.49186218934005E-18,0.984807753012213));
#88245=DIRECTION('center_axis',(-0.173648177666902,1.49186218934005E-18,
-0.984807753012213));
#88246=DIRECTION('ref_axis',(-0.984806496090504,-0.00159769267247533,0.173647956037692));
#88247=DIRECTION('center_axis',(-0.173648177666902,1.49186218934005E-18,
-0.984807753012213));
#88248=DIRECTION('ref_axis',(-0.984806496090504,-0.00159769267247533,0.173647956037692));
#88249=DIRECTION('center_axis',(0.529918793382083,0.000598506209369939,
0.848048179180166));
#88250=DIRECTION('ref_axis',(0.848046930758885,0.00148135485220636,-0.529919058742217));
#88251=DIRECTION('center_axis',(0.984806496090504,0.00159769267247521,-0.173647956037692));
#88252=DIRECTION('ref_axis',(-0.173648177666902,-7.3602384881327E-19,-0.984807753012213));
#88253=DIRECTION('',(0.984806496090504,0.00159769267247521,-0.173647956037692));
#88254=DIRECTION('center_axis',(-0.173648177666903,4.70361612381465E-17,
-0.984807753012213));
#88255=DIRECTION('ref_axis',(0.984806496090504,0.00159769267247229,-0.173647956037693));
#88256=DIRECTION('center_axis',(-0.529918793382001,-0.000598506209405786,
-0.848048179180217));
#88257=DIRECTION('ref_axis',(0.848046930758947,0.00148135484529274,-0.529919058742137));
#88258=DIRECTION('center_axis',(0.173648177666903,1.59201841970382E-16,
0.984807753012213));
#88259=DIRECTION('ref_axis',(0.00157342013078983,-0.999998723688248,-0.000277436421047882));
#88260=DIRECTION('center_axis',(-0.529918793384811,-0.000598506215654095,
-0.848048179178457));
#88261=DIRECTION('ref_axis',(0.848046930757165,0.00148135485777394,-0.529919058744953));
#88262=DIRECTION('center_axis',(0.173648177666903,-6.48778977136688E-18,
0.984807753012213));
#88263=DIRECTION('ref_axis',(-0.984749768728927,-0.0108514562123488,0.173637953473302));
#88264=DIRECTION('center_axis',(0.0106865982093938,-0.99994112121568,-0.00188433559630659));
#88265=DIRECTION('ref_axis',(0.984749768728927,0.0108514562123489,-0.173637953473302));
#88266=DIRECTION('center_axis',(-0.173648177666903,-8.10973730173238E-20,
-0.984807753012213));
#88267=DIRECTION('ref_axis',(0.984806496090504,0.00159769267248121,-0.173647956037693));
#88268=DIRECTION('center_axis',(0.173648177666902,7.29480667023956E-16,
0.984807753012213));
#88269=DIRECTION('ref_axis',(-0.80947494239616,0.569541759667294,0.14273227255185));
#88270=DIRECTION('center_axis',(-0.173648177666909,-8.8187772501904E-18,
-0.984807753012212));
#88271=DIRECTION('ref_axis',(-0.984806496090238,-0.00159769284073281,0.173647956037652));
#88272=DIRECTION('center_axis',(-0.00157342029648582,0.999998723687979,
0.000277436450264715));
#88273=DIRECTION('ref_axis',(0.173648177666899,-3.61333496938023E-18,0.984807753012214));
#88274=DIRECTION('center_axis',(0.173648177666903,2.70178024823687E-16,
0.984807753012213));
#88275=DIRECTION('ref_axis',(-0.808728963551724,-0.570633414289505,0.142600736354538));
#88276=DIRECTION('center_axis',(-0.00157342029648582,0.999998723687979,
0.000277436450264715));
#88277=DIRECTION('ref_axis',(0.173648177666899,-3.61333496938023E-18,0.984807753012214));
#88278=DIRECTION('center_axis',(-0.173648177666904,-2.99281451101198E-15,
-0.984807753012213));
#88279=DIRECTION('ref_axis',(-0.343208372641265,-0.93730769666911,0.0605168961016933));
#88280=DIRECTION('center_axis',(0.984806496090504,0.00159769267247521,-0.173647956037693));
#88281=DIRECTION('ref_axis',(-0.173648177666903,-5.3530757125254E-20,-0.984807753012213));
#88282=DIRECTION('',(0.984806496090504,0.00159769267247521,-0.173647956037693));
#88283=DIRECTION('center_axis',(0.984806496090504,0.00159769267247521,-0.173647956037693));
#88284=DIRECTION('ref_axis',(-0.173648177666903,-3.73849559887003E-19,-0.984807753012213));
#88285=DIRECTION('center_axis',(0.89187284005045,0.424065723658381,-0.157261245061962));
#88286=DIRECTION('ref_axis',(7.57847339502874E-18,-0.347702922065335,-0.937604755740513));
#88287=DIRECTION('',(-0.417623212445505,0.905631416205343,0.0736382401242789));
#88288=DIRECTION('',(0.173648177666903,1.77379537806039E-19,0.984807753012213));
#88289=DIRECTION('',(-0.417623212445505,0.905631416205343,0.0736382401242789));
#88290=DIRECTION('',(0.173648177666806,-1.57202615380602E-16,0.98480775301223));
#88291=DIRECTION('center_axis',(-0.173648177666903,1.42314599624734E-16,
-0.984807753012213));
#88292=DIRECTION('ref_axis',(-0.00157342013078447,0.999998723688248,0.000277436421047244));
#88293=DIRECTION('center_axis',(-0.173648177666903,3.93652485185651E-17,
-0.984807753012213));
#88294=DIRECTION('ref_axis',(0.893202752211758,-0.421169721037697,-0.157495744457965));
#88295=DIRECTION('center_axis',(-0.173648177666903,-2.95239363889238E-17,
-0.984807753012213));
#88296=DIRECTION('ref_axis',(0.893202752211758,-0.421169721037697,-0.157495744457965));
#88297=DIRECTION('',(0.173648177666709,1.74490518016149E-14,0.984807753012247));
#88298=DIRECTION('center_axis',(-0.173648177666903,-1.77379537806039E-19,
-0.984807753012213));
#88299=DIRECTION('ref_axis',(-0.984807753012213,3.83929687396358E-37,0.173648177666903));
#88300=DIRECTION('center_axis',(0.173648177666903,0.,0.984807753012213));
#88301=DIRECTION('ref_axis',(0.417623212445507,-0.905631416205343,-0.0736382401242741));
#88302=DIRECTION('',(0.893202752211756,-0.421169721037697,-0.157495744457976));
#88303=DIRECTION('center_axis',(-0.173648177666903,7.16660291201912E-16,
-0.984807753012213));
#88304=DIRECTION('ref_axis',(-0.00157342013078448,0.999998723688248,0.000277436421047828));
#88305=DIRECTION('center_axis',(-0.173648177666903,-3.48020931800866E-17,
-0.984807753012213));
#88306=DIRECTION('ref_axis',(0.893202752211759,-0.421169721037697,-0.157495744457965));
#88307=DIRECTION('',(0.173648177666903,1.77379537806039E-19,0.984807753012213));
#88308=DIRECTION('center_axis',(-0.414771206611954,-0.906981844405385,0.0731353545466874));
#88309=DIRECTION('ref_axis',(-0.909417241788805,0.415884936415402,2.11769803727567E-18));
#88310=DIRECTION('',(0.893202752211756,-0.421169721037697,-0.157495744457976));
#88311=DIRECTION('center_axis',(0.173648177666903,1.77379537806039E-19,
0.984807753012213));
#88312=DIRECTION('ref_axis',(1.02148804663124E-18,-1.,1.45468743896681E-36));
#88313=DIRECTION('center_axis',(0.173648177666903,-6.88891849074889E-17,
0.984807753012213));
#88314=DIRECTION('ref_axis',(0.891872840050451,0.424065723658381,-0.157261245061954));
#88315=DIRECTION('',(-0.414771206611954,-0.906981844405386,0.0731353545466775));
#88316=DIRECTION('center_axis',(-0.173648177666903,-2.43614652260606E-16,
-0.984807753012213));
#88317=DIRECTION('ref_axis',(0.414771206611955,0.906981844405385,-0.0731353545466813));
#88318=DIRECTION('',(0.89187284005045,0.424065723658381,-0.157261245061962));
#88319=DIRECTION('center_axis',(0.173648177666903,-1.42314599624734E-16,
0.984807753012213));
#88320=DIRECTION('ref_axis',(0.00157342013078447,-0.999998723688248,-0.000277436421047244));
#88321=DIRECTION('',(0.173648177666806,-1.57202615380602E-16,0.98480775301223));
#88322=DIRECTION('',(0.173648177666902,5.32908145459909E-14,0.984807753012213));
#88323=DIRECTION('center_axis',(0.173648177666903,-6.88891849074889E-17,
0.984807753012213));
#88324=DIRECTION('ref_axis',(0.891872840050451,0.424065723658381,-0.157261245061954));
#88325=DIRECTION('center_axis',(-0.893202752211757,0.421169721037697,0.157495744457976));
#88326=DIRECTION('ref_axis',(0.173648177666915,8.8205638096327E-18,0.984807753012211));
#88327=DIRECTION('',(0.173648177666903,1.77379537806039E-19,0.984807753012213));
#88328=DIRECTION('',(-0.414771206611954,-0.906981844405384,0.0731353545466974));
#88329=DIRECTION('center_axis',(0.173648177666903,-7.16660291201912E-16,
0.984807753012213));
#88330=DIRECTION('ref_axis',(0.00157342013078448,-0.999998723688248,-0.000277436421047828));
#88331=DIRECTION('',(0.173648177667,1.57513029571763E-16,0.984807753012196));
#88332=DIRECTION('center_axis',(0.173648177666903,-8.12048840868686E-17,
0.984807753012213));
#88333=DIRECTION('ref_axis',(0.891872840050451,0.424065723658381,-0.157261245061954));
#88334=DIRECTION('center_axis',(0.417623212445504,-0.905631416205343,-0.0736382401242889));
#88335=DIRECTION('ref_axis',(4.02781508425194E-18,0.081044018053505,-0.996710523240195));
#88336=DIRECTION('',(0.89187284005045,0.424065723658381,-0.157261245061962));
#88337=DIRECTION('center_axis',(-0.00145739791678334,-0.999846419038759,
-0.0174646593635094));
#88338=DIRECTION('ref_axis',(-2.53744808518323E-21,0.0174646779110831,-0.99984748088169));
#88339=DIRECTION('',(0.173649190170913,-0.0174523841625769,0.984652920089119));
#88340=DIRECTION('',(0.984806496090239,0.00159769284073286,-0.173647956037646));
#88341=DIRECTION('',(0.173649190225314,-0.0174523841624888,0.984652920079526));
#88342=DIRECTION('',(-0.984806496090294,-0.00159769284073286,0.173647956037338));
#88343=DIRECTION('center_axis',(0.173648177666903,-9.44812840053846E-15,
0.984807753012213));
#88344=DIRECTION('ref_axis',(-0.00157342029648291,0.999998723687979,0.000277436450273798));
#88345=DIRECTION('center_axis',(0.173648177666903,6.91086727774848E-15,
0.984807753012213));
#88346=DIRECTION('ref_axis',(0.00157342029648635,-0.999998723687979,-0.000277436450257794));
#88347=DIRECTION('',(0.190808973440195,2.78835766832232E-5,0.981627187315635));
#88348=DIRECTION('center_axis',(-0.173648177666897,1.00951792985966E-17,
-0.984807753012214));
#88349=DIRECTION('ref_axis',(0.98480649609024,0.00159769284073303,-0.17364795603764));
#88350=DIRECTION('center_axis',(0.981625926717135,0.00159744950437461,-0.190808773780994));
#88351=DIRECTION('ref_axis',(-1.58138488522882E-19,-0.99996495671813,-0.00837169849608073));
#88352=DIRECTION('',(-0.00157342029648582,0.999998723687979,0.000277436450264717));
#88353=DIRECTION('',(0.190808973440108,2.7883631917396E-5,0.981627187315651));
#88354=DIRECTION('',(0.0015734202964251,-0.999998723687979,-0.000277436450577356));
#88355=DIRECTION('center_axis',(0.173648177666903,-6.57942269886179E-19,
0.984807753012213));
#88356=DIRECTION('ref_axis',(-0.984806496090239,-0.00159769284073276,0.173647956037646));
#88357=DIRECTION('center_axis',(0.173648177666894,-1.47993596544271E-17,
0.984807753012215));
#88358=DIRECTION('ref_axis',(0.984806496090241,0.00159769284073259,-0.173647956037637));
#88359=DIRECTION('',(0.173594270245887,0.0174523841625767,0.984662603953679));
#88360=DIRECTION('center_axis',(-0.173648177666903,-3.35757540913268E-15,
-0.984807753012213));
#88361=DIRECTION('ref_axis',(-0.00157342029648637,0.999998723687979,0.000277436450261404));
#88362=DIRECTION('center_axis',(-0.00460375923069061,0.999846419038759,
-0.0169098709728103));
#88363=DIRECTION('ref_axis',(-0.964879947320468,-1.01243743119455E-18,0.262691239402557));
#88364=DIRECTION('',(-0.984806496090239,-0.00159769284073286,0.173647956037646));
#88365=DIRECTION('',(0.173594270191486,0.0174523841624883,0.984662603963271));
#88366=DIRECTION('',(0.984806496090188,0.00159769284073286,-0.173647956037937));
#88367=DIRECTION('center_axis',(0.98480649609024,0.00159769284073286,-0.173647956037645));
#88368=DIRECTION('ref_axis',(-0.173648177666902,-4.25482427716051E-18,-0.984807753012213));
#88369=DIRECTION('center_axis',(0.98480649609024,0.00159769284073286,-0.173647956037645));
#88370=DIRECTION('ref_axis',(0.173648177666902,5.15300653782458E-19,0.984807753012213));
#88371=DIRECTION('center_axis',(0.98480649609024,0.00159769284073286,-0.173647956037645));
#88372=DIRECTION('ref_axis',(0.173648177666902,4.25482427716051E-18,0.984807753012213));
#88373=DIRECTION('',(0.984806496090163,0.00159769288929177,-0.173647956037633));
#88374=DIRECTION('center_axis',(0.173648177666903,-1.63457705018331E-15,
0.984807753012213));
#88375=DIRECTION('ref_axis',(0.224660098927353,-0.973631655051934,-0.039613636929517));
#88376=DIRECTION('center_axis',(0.00157342029648582,-0.999998723687979,
-0.000277436450264715));
#88377=DIRECTION('ref_axis',(0.173648177666901,7.61225010390707E-20,0.984807753012213));
#88378=DIRECTION('center_axis',(-0.173648177666903,4.34089614276706E-15,
-0.984807753012213));
#88379=DIRECTION('ref_axis',(-0.00157342029648684,0.999998723687979,0.000277436450269305));
#88380=DIRECTION('center_axis',(0.00157342029648582,-0.999998723687979,
-0.000277436450264715));
#88381=DIRECTION('ref_axis',(-0.173648177666901,4.11768476579406E-19,-0.984807753012213));
#88382=DIRECTION('center_axis',(0.00157342029648582,-0.999998723687979,
-0.000277436450264715));
#88383=DIRECTION('ref_axis',(0.173648177666901,7.61225010390707E-20,0.984807753012213));
#88384=DIRECTION('',(0.0015734203443027,-0.999998723687901,-0.000277436458698203));
#88385=DIRECTION('center_axis',(0.173648177666904,4.18775938476715E-16,
0.984807753012213));
#88386=DIRECTION('ref_axis',(-0.958840002473252,-0.228125843079737,0.169069362618583));
#88387=DIRECTION('center_axis',(-0.98480649609024,-0.00159769284073286,
0.173647956037645));
#88388=DIRECTION('ref_axis',(0.173648177666902,5.15300653782458E-19,0.984807753012213));
#88389=DIRECTION('center_axis',(-0.173648177666903,5.80467749850325E-19,
-0.984807753012213));
#88390=DIRECTION('ref_axis',(0.984806496090239,0.00159769284073277,-0.173647956037646));
#88391=DIRECTION('center_axis',(-0.98480649609024,-0.00159769284073286,
0.173647956037645));
#88392=DIRECTION('ref_axis',(-0.173648177666902,-4.25482427716051E-18,-0.984807753012213));
#88393=DIRECTION('center_axis',(-0.98480649609024,-0.00159769284073286,
0.173647956037645));
#88394=DIRECTION('ref_axis',(0.173648177666902,4.25482427716051E-18,0.984807753012213));
#88395=DIRECTION('',(-0.984806496090163,-0.00159769288928886,0.173647956037633));
#88396=DIRECTION('center_axis',(0.173648177666903,-1.63457705018331E-15,
0.984807753012213));
#88397=DIRECTION('ref_axis',(-0.224660098927352,0.973631655051934,0.039613636929517));
#88398=DIRECTION('center_axis',(-0.00157342029648582,0.999998723687979,
0.000277436450264715));
#88399=DIRECTION('ref_axis',(0.173648177666899,-3.61333496938023E-18,0.984807753012214));
#88400=DIRECTION('center_axis',(-0.173648177666903,-3.35757540913268E-15,
-0.984807753012213));
#88401=DIRECTION('ref_axis',(0.00157342029648637,-0.999998723687979,-0.000277436450261404));
#88402=DIRECTION('center_axis',(-0.173648177666903,4.55102546821287E-15,
-0.984807753012213));
#88403=DIRECTION('ref_axis',(0.00157342029648563,-0.999998723687979,-0.000277436450269305));
#88404=DIRECTION('center_axis',(0.173648177666899,-5.37964561848111E-18,
0.984807753012214));
#88405=DIRECTION('ref_axis',(0.98480649609024,0.00159769284073276,-0.173647956037643));
#88406=DIRECTION('',(0.156434486976668,-2.78836790155617E-5,0.987688336727152));
#88407=DIRECTION('center_axis',(0.173648177666894,-1.47993596544271E-17,
0.984807753012215));
#88408=DIRECTION('ref_axis',(-0.984806496090241,-0.00159769284073259,0.173647956037637));
#88409=DIRECTION('center_axis',(-0.987687083864603,-0.00159744950437461,
0.156434243444705));
#88410=DIRECTION('ref_axis',(-0.00161736185591408,0.999998692069458,-1.3098294468559E-20));
#88411=DIRECTION('',(-0.0015672529834684,0.999998721807879,0.000316386936718628));
#88412=DIRECTION('',(-0.156434487048126,2.79785493473008E-5,-0.987688336713151));
#88413=DIRECTION('',(0.00157343755135569,-0.999998723691179,-0.000277327037485099));
#88414=DIRECTION('center_axis',(-0.00157342029648582,0.999998723687979,
0.000277436450264715));
#88415=DIRECTION('ref_axis',(0.813978516242862,0.00111957060601937,0.580893898794544));
#88416=DIRECTION('center_axis',(-0.173648177666903,1.67985947297096E-15,
-0.984807753012213));
#88417=DIRECTION('ref_axis',(0.343208372641262,0.937307696669111,-0.0605168961016879));
#88418=DIRECTION('center_axis',(-0.173648177666903,7.07772878971226E-16,
-0.984807753012213));
#88419=DIRECTION('ref_axis',(-0.343208372641267,-0.937307696669109,0.0605168961016898));
#88420=DIRECTION('',(-0.167631936046611,0.016358281640073,-0.985713924340652));
#88421=DIRECTION('center_axis',(-0.819151155511157,-0.00112973932296881,
-0.573576593066522));
#88422=DIRECTION('ref_axis',(0.573575547587063,0.00112973047439091,-0.819151887575959));
#88423=DIRECTION('center_axis',(-0.00111431000077956,0.999999196217831,
0.000604877603267272));
#88424=DIRECTION('ref_axis',(-0.814897680756574,-0.0005574592593905,-0.579604571355964));
#88425=DIRECTION('center_axis',(0.0019082391455338,-0.999997900468177,-0.000746781495225125));
#88426=DIRECTION('ref_axis',(-0.581802269400352,-0.00171760010831627,0.81332845097812));
#88427=DIRECTION('center_axis',(0.173648177666903,-3.30780989858582E-15,
0.984807753012213));
#88428=DIRECTION('ref_axis',(0.0015734202964841,-0.999998723687979,-0.000277436450267774));
#88429=DIRECTION('',(0.156434486976398,-2.78835073328855E-5,0.987688336727199));
#88430=DIRECTION('',(-0.16758048981795,-0.0163387632005932,-0.985722995698817));
#88431=DIRECTION('center_axis',(0.819151155513041,0.00112973931574178,0.573576593063845));
#88432=DIRECTION('ref_axis',(0.573575547570477,0.00112973931585084,-0.819151887575378));
#88433=DIRECTION('center_axis',(-0.987687083864603,-0.00159744950437461,
0.156434243444705));
#88434=DIRECTION('ref_axis',(-0.00161736185591408,0.999998692069458,-1.3098294468559E-20));
#88435=DIRECTION('',(0.156434486976551,-2.78836043610342E-5,0.987688336727172));
#88436=DIRECTION('',(-0.00157342029645223,0.999998723687979,0.000277436450476588));
#88437=DIRECTION('',(0.00157342026969061,-0.999998723687974,-0.000277436619430731));
#88438=DIRECTION('center_axis',(0.1736481776669,-5.09813795295912E-18,0.984807753012213));
#88439=DIRECTION('ref_axis',(0.98480649609024,0.00159769284073301,-0.173647956037644));
#88440=DIRECTION('center_axis',(0.819151155513551,0.00112973933284856,0.573576593063084));
#88441=DIRECTION('ref_axis',(0.573575547569693,0.00112973932749382,-0.819151887575911));
#88442=DIRECTION('center_axis',(-0.00157342029648582,0.999998723687979,
0.000277436450264715));
#88443=DIRECTION('ref_axis',(-0.173648177666899,4.10122594699871E-18,-0.984807753012214));
#88444=DIRECTION('',(-0.00157342029692248,0.999998723687978,0.000277436450337063));
#88445=DIRECTION('center_axis',(-0.173648177666916,-2.23918124064188E-17,
-0.984807753012211));
#88446=DIRECTION('ref_axis',(0.984806496049417,0.00159771878360705,-0.173647956030462));
#88447=DIRECTION('center_axis',(-0.00157342029648582,0.999998723687979,
0.000277436450264715));
#88448=DIRECTION('ref_axis',(0.813978512696035,0.00111957059905984,0.580893903764556));
#88449=DIRECTION('center_axis',(-0.00157342029648582,0.999998723687979,
0.000277436450264715));
#88450=DIRECTION('ref_axis',(0.173648177666899,-3.61333496938023E-18,0.984807753012214));
#88451=DIRECTION('',(-0.00157958616680064,0.999998724013009,0.00023849506217036));
#88452=DIRECTION('center_axis',(0.173648177666904,4.18775938476715E-16,
0.984807753012213));
#88453=DIRECTION('ref_axis',(0.958840002473252,0.228125843079737,-0.169069362618583));
#88454=DIRECTION('center_axis',(-0.173648177666897,1.00951792985966E-17,
-0.984807753012214));
#88455=DIRECTION('ref_axis',(-0.98480649609024,-0.00159769284073303,0.17364795603764));
#88456=DIRECTION('center_axis',(-0.173648177666903,6.33237545291264E-19,
-0.984807753012213));
#88457=DIRECTION('ref_axis',(-0.984806496090239,-0.00159769284070554,0.173647956037646));
#88458=DIRECTION('center_axis',(0.173648177666903,-4.92055672404642E-15,
0.984807753012213));
#88459=DIRECTION('ref_axis',(0.00157342029648369,-0.999998723687979,-0.000277436450269339));
#88460=DIRECTION('center_axis',(0.173648177666903,6.91086727774848E-15,
0.984807753012213));
#88461=DIRECTION('ref_axis',(-0.00157342029648636,0.999998723687979,0.000277436450257794));
#88462=DIRECTION('',(0.156434486976507,-2.78835766825765E-5,0.98768833672718));
#88463=DIRECTION('center_axis',(-0.987687083864603,-0.00159744950437461,
0.156434243444705));
#88464=DIRECTION('ref_axis',(-0.00161736185591408,0.999998692069458,-1.3098294468559E-20));
#88465=DIRECTION('',(-0.156434486979456,2.79313446666122E-5,-0.987688336725363));
#88466=DIRECTION('',(0.00157342022766082,-0.999998723688078,-0.000277436481588655));
#88467=DIRECTION('center_axis',(-0.173648177666904,-2.48013246669082E-18,
-0.984807753012213));
#88468=DIRECTION('ref_axis',(0.809998687527633,-0.568773463940462,-0.142824622949545));
#88469=DIRECTION('center_axis',(-0.819151155512569,-0.0011297393161222,
-0.573576593064518));
#88470=DIRECTION('ref_axis',(0.573575547571143,0.00112973932052989,-0.819151887574906));
#88471=DIRECTION('center_axis',(0.819151155511153,0.00112973932295936,0.573576593066528));
#88472=DIRECTION('ref_axis',(4.42381266920449E-20,-0.999998060265046,0.0019696360437663));
#88473=DIRECTION('',(0.00157341843450662,-0.999998723688043,-0.000277446777199153));
#88474=DIRECTION('center_axis',(-0.173648177666903,-1.77379537806039E-19,
-0.984807753012213));
#88475=DIRECTION('ref_axis',(-0.984807753012213,3.83929687396358E-37,0.173648177666903));
#88476=DIRECTION('',(0.00157342029648582,-0.999998723687979,-0.000277436450264717));
#88477=DIRECTION('',(0.984806496090239,0.00159769284073286,-0.173647956037646));
#88478=DIRECTION('',(-0.00157342029648582,0.999998723687979,0.000277436450264717));
#88479=DIRECTION('',(0.984806496090239,0.00159769284073286,-0.173647956037646));
#88480=DIRECTION('',(-0.00157342029648582,0.999998723687979,0.000277436450264717));
#88481=DIRECTION('',(-0.984806496090239,-0.00159769284073286,0.173647956037646));
#88482=DIRECTION('',(-0.00157342029648582,0.999998723687979,0.000277436450264717));
#88483=DIRECTION('',(-0.984806496090239,-0.00159769284073286,0.173647956037646));
#88484=DIRECTION('center_axis',(-0.984806496090239,-0.00159769284073286,
0.173647956037646));
#88485=DIRECTION('ref_axis',(-0.0016223397637217,0.99999868400598,2.63557796693769E-20));
#88486=DIRECTION('',(0.173648177666903,1.77379537806039E-19,0.984807753012213));
#88487=DIRECTION('',(0.173648177666903,1.77379537806039E-19,0.984807753012213));
#88488=DIRECTION('',(-0.00157342029648582,0.999998723687979,0.000277436450264717));
#88489=DIRECTION('center_axis',(0.00157342029648582,-0.999998723687979,
-0.000277436450264717));
#88490=DIRECTION('ref_axis',(-2.2370400977484E-23,0.000277436793683327,
-0.999999961514412));
#88491=DIRECTION('',(0.173648177666903,1.77379537806039E-19,0.984807753012213));
#88492=DIRECTION('',(-0.984806496090239,-0.00159769284073286,0.173647956037646));
#88493=DIRECTION('center_axis',(0.984806496090239,0.00159769284073286,-0.173647956037646));
#88494=DIRECTION('ref_axis',(-1.16826950231067E-19,-0.999957675712221,-0.00920036869984769));
#88495=DIRECTION('',(0.173648177666903,1.77379537806039E-19,0.984807753012213));
#88496=DIRECTION('',(0.00157342029648582,-0.999998723687979,-0.00027743645028658));
#88497=DIRECTION('center_axis',(0.00157342029648582,-0.999998723687979,
-0.000277436450264717));
#88498=DIRECTION('ref_axis',(-2.2370400977484E-23,0.000277436793683327,
-0.999999961514412));
#88499=DIRECTION('',(0.173648177666903,1.77379537806039E-19,0.984807753012213));
#88500=DIRECTION('',(-0.984806496090222,-0.00159769284073286,0.173647956037743));
#88501=DIRECTION('center_axis',(0.984806496090239,0.00159769284073286,-0.173647956037646));
#88502=DIRECTION('ref_axis',(-1.16826950231067E-19,-0.999957675712221,-0.00920036869984769));
#88503=DIRECTION('',(0.173648177666903,1.77379537806039E-19,0.984807753012213));
#88504=DIRECTION('',(0.00157342029648582,-0.999998723687979,-0.000277436450264717));
#88505=DIRECTION('center_axis',(-0.00157342029648582,0.999998723687979,
0.000277436450264717));
#88506=DIRECTION('ref_axis',(0.173648177666903,-3.52094571672426E-20,0.984807753012213));
#88507=DIRECTION('',(0.173648177666903,1.77379537806039E-19,0.984807753012213));
#88508=DIRECTION('',(0.984806496090222,0.00159769284073286,-0.173647956037743));
#88509=DIRECTION('center_axis',(0.984806496090239,0.00159769284073286,-0.173647956037646));
#88510=DIRECTION('ref_axis',(-1.16826950231067E-19,-0.999957675712221,-0.00920036869984769));
#88511=DIRECTION('',(0.173648177666903,1.77379537806039E-19,0.984807753012213));
#88512=DIRECTION('',(0.00157342029648582,-0.999998723687979,-0.000277436450264717));
#88513=DIRECTION('center_axis',(-0.00157342029648582,0.999998723687979,
0.000277436450264717));
#88514=DIRECTION('ref_axis',(0.173648177666903,-3.52094571672426E-20,0.984807753012213));
#88515=DIRECTION('',(0.984806496090239,0.00159769284073286,-0.173647956037646));
#88516=DIRECTION('center_axis',(0.173648177666903,1.77379537806039E-19,
0.984807753012213));
#88517=DIRECTION('ref_axis',(1.02148804663124E-18,-1.,1.45468743896681E-36));
#88518=DIRECTION('center_axis',(0.173648177666903,1.77379537806039E-19,
0.984807753012213));
#88519=DIRECTION('ref_axis',(1.02148804663124E-18,-1.,1.45468743896681E-36));
#88520=DIRECTION('center_axis',(0.529918793382054,0.000598506209361558,
0.848048179180184));
#88521=DIRECTION('ref_axis',(0.0011294293297492,-0.999999362194491,-4.78634101357847E-20));
#88522=DIRECTION('',(0.00157342013088156,-0.999998723688247,-0.000277436420824379));
#88523=DIRECTION('',(0.00157342013076796,-0.999998723688248,-0.000277436421032639));
#88524=DIRECTION('center_axis',(0.173648177666903,1.77379537806039E-19,
0.984807753012213));
#88525=DIRECTION('ref_axis',(1.02148804663124E-18,-1.,1.45468743896681E-36));
#88526=DIRECTION('center_axis',(-0.314055242383514,-0.91431658158538,-0.255723470509566));
#88527=DIRECTION('ref_axis',(0.629237412598948,0.00124254729691768,-0.777212155503242));
#88528=DIRECTION('center_axis',(0.316965079769398,-0.913473350106414,0.255146187218511));
#88529=DIRECTION('ref_axis',(0.629162965906753,0.00120921019910097,-0.777272474838851));
#88530=DIRECTION('center_axis',(0.662632777829612,0.144272974524305,0.734917077341194));
#88531=DIRECTION('ref_axis',(0.742560405946752,0.00129143749156779,-0.669777855493447));
#88532=DIRECTION('center_axis',(0.146692737802188,0.952760334528529,-0.265949216252245));
#88533=DIRECTION('ref_axis',(-0.000412525464939198,0.268916590385109,0.963163380345406));
#88534=DIRECTION('center_axis',(-0.239999751079929,-0.186076176852954,-0.952772677971698));
#88535=DIRECTION('ref_axis',(-0.00155278376594829,0.9815301219139,-0.191301355557826));
#88536=DIRECTION('center_axis',(0.999998762173495,0.00157342029648582,2.18262210013629E-7));
#88537=DIRECTION('ref_axis',(-2.18262210388565E-7,0.000277436450264733,
-0.999999961514484));
#88538=DIRECTION('',(0.999998762247466,0.00157337326398415,3.28322100784373E-7));
#88539=DIRECTION('center_axis',(0.240601503772138,-0.185862702176551,0.95266257002268));
#88540=DIRECTION('ref_axis',(0.00153245606422671,-0.981421019486281,-0.191860454729264));
#88541=DIRECTION('center_axis',(-0.149644118021572,0.952159144810393,0.266457502982158));
#88542=DIRECTION('ref_axis',(0.000424375672975945,-0.269430126258093,0.963019847651042));
#88543=DIRECTION('center_axis',(0.999998762173495,0.00157342029648582,2.18262210013629E-7));
#88544=DIRECTION('ref_axis',(-2.18262210388565E-7,0.000277436450264733,
-0.999999961514484));
#88545=DIRECTION('',(0.999998762516763,0.00157320126714693,1.64818022882485E-6));
#88546=DIRECTION('center_axis',(-0.663074807330075,0.142596683678673,-0.734845552267978));
#88547=DIRECTION('ref_axis',(0.742562201227128,0.00135037093647457,-0.669775748894401));
#88548=DIRECTION('center_axis',(-0.252940505516454,0.721654216431443,-0.644388308844753));
#88549=DIRECTION('ref_axis',(0.931456534788202,0.00158377533602745,-0.363849165803687));
#88550=DIRECTION('center_axis',(0.250670969471596,0.722091646399503,0.644785017865819));
#88551=DIRECTION('ref_axis',(0.00105715928539588,-0.666254233378766,0.745723929426378));
#88552=DIRECTION('center_axis',(0.999998762173495,0.00157342029648582,2.1826221001363E-7));
#88553=DIRECTION('ref_axis',(-2.18262210388565E-7,0.000277436450264734,
-0.999999961514484));
#88554=DIRECTION('',(0.999998762173495,0.00157342029648582,2.18262209944475E-7));
#88555=DIRECTION('center_axis',(0.134465664742365,0.000413144039032103,
0.990918167316251));
#88556=DIRECTION('ref_axis',(0.990647603194621,-0.0234266874123494,-0.134419182416933));
#88557=DIRECTION('center_axis',(-0.275261853306783,-0.318164219754394,-0.907194819970988));
#88558=DIRECTION('ref_axis',(-0.927511143457601,0.336119090075094,0.16354521102455));
#88559=DIRECTION('center_axis',(-0.00157337729948021,0.999998723772464,
0.000277375768317332));
#88560=DIRECTION('ref_axis',(-0.98480671474633,-0.00159763995970335,0.173646716459311));
#88561=DIRECTION('center_axis',(0.276268688411157,-0.317806043628553,0.907014294505189));
#88562=DIRECTION('ref_axis',(-0.926448783505642,-0.33912381130528,0.163363680623008));
#88563=DIRECTION('center_axis',(0.999998762173495,0.00157342029648582,2.1826221001363E-7));
#88564=DIRECTION('ref_axis',(-2.18262210388565E-7,0.000277436450264734,
-0.999999961514484));
#88565=DIRECTION('center_axis',(0.134373628028009,0.000182201052963753,
0.990930721540798));
#88566=DIRECTION('ref_axis',(0.990818423918398,0.0150309177067826,-0.134361163796515));
#88567=DIRECTION('',(0.999998762173495,0.00157342029648582,2.18262209944475E-7));
#88568=DIRECTION('center_axis',(0.999998762173495,0.00157342029648582,2.18262210013657E-7));
#88569=DIRECTION('ref_axis',(2.18261402645051E-7,-0.000277435936897481,
0.999999961514626));
#88570=DIRECTION('center_axis',(0.966997552472099,-0.18932204760366,-0.170507758779852));
#88571=DIRECTION('ref_axis',(-0.17364740989288,4.04346645584571E-6,-0.984807888382879));
#88572=DIRECTION('center_axis',(-0.966395599704911,-0.192457245450031,0.170410544112656));
#88573=DIRECTION('ref_axis',(0.00103847482039741,-0.66584029656634,-0.74609357391583));
#88574=DIRECTION('center_axis',(0.975127266349125,-0.139841305698193,-0.171962855416822));
#88575=DIRECTION('ref_axis',(-0.00123501906440318,0.772405548492563,-0.635128446367987));
#88576=DIRECTION('center_axis',(0.173651504889683,2.11958655523597E-5,0.984807166099173));
#88577=DIRECTION('ref_axis',(0.984521190641717,-0.0241012604084658,-0.173600559976454));
#88578=DIRECTION('center_axis',(-0.974685226395651,-0.143017999760238,0.171856222437942));
#88579=DIRECTION('ref_axis',(0.00122150236050521,-0.772045967302346,-0.635565521645226));
#88580=DIRECTION('center_axis',(0.173652216761134,-2.53504643415288E-5,
0.984807040476102));
#88581=DIRECTION('ref_axis',(0.984520060172094,0.0241442914896521,-0.173600991665369));
#88582=DIRECTION('center_axis',(0.173648177666903,1.77379537806039E-19,
0.984807753012213));
#88583=DIRECTION('ref_axis',(1.02148804663124E-18,-1.,1.45468743896681E-36));
#158205=CARTESIAN_POINT('',(0.,0.,0.));
#158206=CARTESIAN_POINT('Origin',(26.6896610501315,-1.66681552173398E-14,
151.364589485454));
#158207=CARTESIAN_POINT('',(46.6311526176588,-7.22655593335579,147.848368540858));
#158208=CARTESIAN_POINT('',(5.51632265081665,-0.0343503924582198,155.098027723626));
#158209=CARTESIAN_POINT('Origin',(26.6896610501315,-1.66681552173398E-14,
151.364589485454));
#158210=CARTESIAN_POINT('',(46.5922727658143,-6.01049908472091,148.362935266823));
#158211=CARTESIAN_POINT('Ctrl Pts',(46.592272697957,-6.01049893749535,148.362935371323));
#158212=CARTESIAN_POINT('Ctrl Pts',(46.6144830676967,-5.9974822785011,148.359019105243));
#158213=CARTESIAN_POINT('Ctrl Pts',(46.6351119736002,-5.98996913036867,
148.354404235172));
#158214=CARTESIAN_POINT('Ctrl Pts',(46.6541344752789,-5.98752441441695,
148.349041555766));
#158215=CARTESIAN_POINT('Ctrl Pts',(46.6736823414854,-5.98501218016174,
148.343530769577));
#158216=CARTESIAN_POINT('Ctrl Pts',(46.6915328413437,-5.98785213129854,
148.337230105633));
#158217=CARTESIAN_POINT('Ctrl Pts',(46.7076331609104,-5.99555810475863,
148.330134203584));
#158218=CARTESIAN_POINT('Ctrl Pts',(46.7242892474038,-6.00353008071449,
148.322793358093));
#158219=CARTESIAN_POINT('Ctrl Pts',(46.739071016055,-6.0167097143341,148.314601354749));
#158220=CARTESIAN_POINT('Ctrl Pts',(46.7519101453899,-6.03454524601735,
148.305605204033));
#158221=CARTESIAN_POINT('Ctrl Pts',(46.7571747445889,-6.04185858661581,
148.301916392539));
#158222=CARTESIAN_POINT('Ctrl Pts',(46.7621127120552,-6.04995460487111,
148.298092981991));
#158223=CARTESIAN_POINT('Ctrl Pts',(46.7667196262217,-6.058794711895,148.294140644901));
#158224=CARTESIAN_POINT('Ctrl Pts',(46.7802991102161,-6.08485208728866,
148.282490612729));
#158225=CARTESIAN_POINT('Ctrl Pts',(46.7911285461141,-6.11693779180763,
148.269696104708));
#158226=CARTESIAN_POINT('Ctrl Pts',(46.7993490990491,-6.15360029378031,
148.255851527001));
#158227=CARTESIAN_POINT('Ctrl Pts',(46.8071143454513,-6.18823219309309,
148.242773750108));
#158228=CARTESIAN_POINT('Ctrl Pts',(46.8125506373435,-6.22694730095852,
148.228759733826));
#158229=CARTESIAN_POINT('Ctrl Pts',(46.8158102675014,-6.26850580218765,
148.21391438593));
#158230=CARTESIAN_POINT('Ctrl Pts',(46.8185709816293,-6.30370339698346,
148.201341253493));
#158231=CARTESIAN_POINT('Ctrl Pts',(46.8197706507559,-6.34094015738946,
148.188172356552));
#158232=CARTESIAN_POINT('Ctrl Pts',(46.8195289914499,-6.3794577430535,148.174481598226));
#158233=CARTESIAN_POINT('Ctrl Pts',(46.8192248796204,-6.42792950951748,
148.157252708387));
#158234=CARTESIAN_POINT('Ctrl Pts',(46.8166546262969,-6.47841958647206,
148.139178171846));
#158235=CARTESIAN_POINT('Ctrl Pts',(46.8119082091704,-6.53008108437151,
148.120433281528));
#158236=CARTESIAN_POINT('Ctrl Pts',(46.8072393702522,-6.58089819663437,
148.101994768624));
#158237=CARTESIAN_POINT('Ctrl Pts',(46.8004647856395,-6.63284840171413,
148.082907929366));
#158238=CARTESIAN_POINT('Ctrl Pts',(46.7917193796614,-6.68512593250974,
148.06334941683));
#158239=CARTESIAN_POINT('Ctrl Pts',(46.7851181003292,-6.72458648865097,
148.048586099392));
#158240=CARTESIAN_POINT('Ctrl Pts',(46.7773949212129,-6.76423351280253,
148.033554260372));
#158241=CARTESIAN_POINT('Ctrl Pts',(46.768627364254,-6.80372239658839,148.018332209879));
#158242=CARTESIAN_POINT('Ctrl Pts',(46.7573214772964,-6.85464386288281,
147.998703163504));
#158243=CARTESIAN_POINT('Ctrl Pts',(46.7442722310709,-6.90531476842511,
147.97876071212));
#158244=CARTESIAN_POINT('Ctrl Pts',(46.7295296446186,-6.9554691842044,147.958735860062));
#158245=CARTESIAN_POINT('Ctrl Pts',(46.7147691166906,-7.00568463705029,
147.938686638101));
#158246=CARTESIAN_POINT('Ctrl Pts',(46.6983111758215,-7.05538213512469,
147.91855543384));
#158247=CARTESIAN_POINT('Ctrl Pts',(46.6802562768064,-7.10430939864112,
147.898573855963));
#158248=CARTESIAN_POINT('Ctrl Pts',(46.664999047466,-7.1456552117551,147.88168849338));
#158249=CARTESIAN_POINT('Ctrl Pts',(46.64860236062,-7.18645120184107,147.864910163264));
#158250=CARTESIAN_POINT('Ctrl Pts',(46.6311537904856,-7.22655473104065,
147.848373621278));
#158251=CARTESIAN_POINT('',(46.5732575347653,6.074764193991,148.366288161248));
#158252=CARTESIAN_POINT('Origin',(26.7764851389615,-2.04263841746052E-14,
151.856993361954));
#158253=CARTESIAN_POINT('',(46.6083116808377,7.29121844351931,147.852402231042));
#158254=CARTESIAN_POINT('Ctrl Pts',(46.6083123648192,7.29121885610936,147.852402503935));
#158255=CARTESIAN_POINT('Ctrl Pts',(46.629098730082,7.24384081903475,147.871934753254));
#158256=CARTESIAN_POINT('Ctrl Pts',(46.6484155685107,7.19548878528177,147.891804947096));
#158257=CARTESIAN_POINT('Ctrl Pts',(46.6661206992522,7.14640049424429,147.911789154575));
#158258=CARTESIAN_POINT('Ctrl Pts',(46.6838077808551,7.09736224527508,147.931752989557));
#158259=CARTESIAN_POINT('Ctrl Pts',(46.699886262435,7.04758940618498,147.951830001543));
#158260=CARTESIAN_POINT('Ctrl Pts',(46.7142629109001,6.99733606536463,147.971788999166));
#158261=CARTESIAN_POINT('Ctrl Pts',(46.7264430853448,6.95476046374863,147.988698647711));
#158262=CARTESIAN_POINT('Ctrl Pts',(46.7374025380023,6.91184032817418,148.005523251997));
#158263=CARTESIAN_POINT('Ctrl Pts',(46.7471127455659,6.86873826094321,148.022122681677));
#158264=CARTESIAN_POINT('Ctrl Pts',(46.7588660208026,6.81656734120588,148.042214699744));
#158265=CARTESIAN_POINT('Ctrl Pts',(46.7687942102469,6.76411203487173,148.061974411536));
#158266=CARTESIAN_POINT('Ctrl Pts',(46.7767215184415,6.71216953488076,148.081221976832));
#158267=CARTESIAN_POINT('Ctrl Pts',(46.7847711291542,6.65942566595162,148.100766493583));
#158268=CARTESIAN_POINT('Ctrl Pts',(46.7907576638701,6.60721090429097,148.119782660209));
#158269=CARTESIAN_POINT('Ctrl Pts',(46.7945507233129,6.55636449864328,148.138089286346));
#158270=CARTESIAN_POINT('Ctrl Pts',(46.797397365301,6.51820492971532,148.151828172172));
#158271=CARTESIAN_POINT('Ctrl Pts',(46.7990097341067,6.48081618753838,148.165167541349));
#158272=CARTESIAN_POINT('Ctrl Pts',(46.7993515207053,6.44455284067278,148.178034849603));
#158273=CARTESIAN_POINT('Ctrl Pts',(46.7997762982508,6.39948420563544,148.194026534589));
#158274=CARTESIAN_POINT('Ctrl Pts',(46.798221872536,6.35616280553221,148.209304529387));
#158275=CARTESIAN_POINT('Ctrl Pts',(46.7944964971984,6.31580176935984,148.223752333791));
#158276=CARTESIAN_POINT('Ctrl Pts',(46.7905490980168,6.27303530780383,148.239061194272));
#158277=CARTESIAN_POINT('Ctrl Pts',(46.7841648875179,6.23359325766264,148.253437231881));
#158278=CARTESIAN_POINT('Ctrl Pts',(46.7751709819016,6.19890721773494,148.266764157202));
#158279=CARTESIAN_POINT('Ctrl Pts',(46.7677608266292,6.17032909465762,148.277744324233));
#158280=CARTESIAN_POINT('Ctrl Pts',(46.7585806685715,6.14497939587087,148.288012596913));
#158281=CARTESIAN_POINT('Ctrl Pts',(46.7475524713142,6.1236485023314,148.297519676975));
#158282=CARTESIAN_POINT('Ctrl Pts',(46.7364156891186,6.10210758228424,148.307120364876));
#158283=CARTESIAN_POINT('Ctrl Pts',(46.7233062761893,6.08496303983045,148.315957464712));
#158284=CARTESIAN_POINT('Ctrl Pts',(46.7082887242939,6.07276715603841,148.32396398118));
#158285=CARTESIAN_POINT('Ctrl Pts',(46.693623205093,6.0608571610426,148.331782813558));
#158286=CARTESIAN_POINT('Ctrl Pts',(46.6771391359373,6.05366667657209,148.338809443837));
#158287=CARTESIAN_POINT('Ctrl Pts',(46.6588949049778,6.05169860747618,148.345028922708));
#158288=CARTESIAN_POINT('Ctrl Pts',(46.6413878518859,6.0498100603389,148.350997096814));
#158289=CARTESIAN_POINT('Ctrl Pts',(46.6222609319471,6.05273047192043,148.356222244022));
#158290=CARTESIAN_POINT('Ctrl Pts',(46.6015490857105,6.06089226979178,148.360734230142));
#158291=CARTESIAN_POINT('Ctrl Pts',(46.5924259545905,6.06448736949,148.362721664798));
#158292=CARTESIAN_POINT('Ctrl Pts',(46.5829950097966,6.06909924750259,148.364571287597));
#158293=CARTESIAN_POINT('Ctrl Pts',(46.5732574663672,6.07476404354701,148.366288269697));
#158294=CARTESIAN_POINT('Origin',(26.6896610501315,-1.66681552173398E-14,
151.364589485454));
#158295=CARTESIAN_POINT('Origin',(20.7595757828115,-1.33056427483082E-16,
117.733404720054));
#158296=CARTESIAN_POINT('',(46.0417820332401,-4.21831552016986,139.708826847192));
#158297=CARTESIAN_POINT('',(46.3509510310709,0.0343503924439632,139.055898541647));
#158298=CARTESIAN_POINT('Ctrl Pts',(46.0417820332401,-4.21831552016986,
139.708826847192));
#158299=CARTESIAN_POINT('Ctrl Pts',(46.0798964649748,-3.96069965430408,
139.628141305823));
#158300=CARTESIAN_POINT('Ctrl Pts',(46.1145382929002,-3.7023636146849,139.555238670999));
#158301=CARTESIAN_POINT('Ctrl Pts',(46.145633349218,-3.44379565574912,139.489959447747));
#158302=CARTESIAN_POINT('Ctrl Pts',(46.176779243046,-3.18480496237181,139.424573499068));
#158303=CARTESIAN_POINT('Ctrl Pts',(46.204366746486,-2.92558188626453,139.366835911588));
#158304=CARTESIAN_POINT('Ctrl Pts',(46.2283726896026,-2.66662111980495,
139.316577350232));
#158305=CARTESIAN_POINT('Ctrl Pts',(46.2524801304473,-2.40656546074536,
139.266106294421));
#158306=CARTESIAN_POINT('Ctrl Pts',(46.2729756665083,-2.14677463153881,
139.223177640495));
#158307=CARTESIAN_POINT('Ctrl Pts',(46.2898876726048,-1.88774922729219,
139.187610755653));
#158308=CARTESIAN_POINT('Ctrl Pts',(46.3068526632686,-1.62791230790918,
139.151932441334));
#158309=CARTESIAN_POINT('Ctrl Pts',(46.3202116902603,-1.36884591102246,
139.123662086757));
#158310=CARTESIAN_POINT('Ctrl Pts',(46.3300449792115,-1.11105049051174,
139.102608260532));
#158311=CARTESIAN_POINT('Ctrl Pts',(46.3399398726735,-0.851640009074977,
139.081422534321));
#158312=CARTESIAN_POINT('Ctrl Pts',(46.3462647840154,-0.593516770546314,
139.06754402874));
#158313=CARTESIAN_POINT('Ctrl Pts',(46.3491526922906,-0.33718134924774,
139.060768657603));
#158314=CARTESIAN_POINT('Ctrl Pts',(46.3505528770535,-0.212898679269364,
139.057483660115));
#158315=CARTESIAN_POINT('Ctrl Pts',(46.3511458716836,-0.0890361107474958,
139.055868288421));
#158316=CARTESIAN_POINT('Ctrl Pts',(46.3509510310709,0.0343503924439631,
139.055898541647));
#158317=CARTESIAN_POINT('',(46.1497547374386,-7.65783120162291,146.034362956251));
#158318=CARTESIAN_POINT('Ctrl Pts',(46.1497339363911,-7.6578231488931,146.034366627848));
#158319=CARTESIAN_POINT('Ctrl Pts',(46.1042153651043,-7.68998708971556,
145.846479401818));
#158320=CARTESIAN_POINT('Ctrl Pts',(46.0629773097244,-7.71232938446267,
145.66225894746));
#158321=CARTESIAN_POINT('Ctrl Pts',(46.0072879996495,-7.73350808720076,
145.393632086788));
#158322=CARTESIAN_POINT('Ctrl Pts',(45.9897496172286,-7.7385121747197,145.305359799572));
#158323=CARTESIAN_POINT('Ctrl Pts',(45.9566301524631,-7.74481940759447,
145.131590450506));
#158324=CARTESIAN_POINT('Ctrl Pts',(45.941260819711,-7.74613449772924,145.047333435302));
#158325=CARTESIAN_POINT('Ctrl Pts',(45.8965248889764,-7.7453198499371,144.791744275131));
#158326=CARTESIAN_POINT('Ctrl Pts',(45.869145516159,-7.73806024054962,144.620256010497));
#158327=CARTESIAN_POINT('Ctrl Pts',(45.8321120275292,-7.71652195814888,
144.362521087448));
#158328=CARTESIAN_POINT('Ctrl Pts',(45.8204410308522,-7.7075650961645,144.276525090039));
#158329=CARTESIAN_POINT('Ctrl Pts',(45.8039994313618,-7.6913670319232,144.147544670468));
#158330=CARTESIAN_POINT('Ctrl Pts',(45.7960449821503,-7.68257696548179,
144.083057840277));
#158331=CARTESIAN_POINT('Ctrl Pts',(45.7885009205254,-7.67273025071386,
144.0186025713));
#158332=CARTESIAN_POINT('Ctrl Pts',(45.7835622888294,-7.66593221096656,
143.975643011381));
#158333=CARTESIAN_POINT('Ctrl Pts',(45.7813306285701,-7.66270987102601,
143.955903486097));
#158334=CARTESIAN_POINT('Ctrl Pts',(45.7684766770574,-7.64307962434864,
143.839891445313));
#158335=CARTESIAN_POINT('Ctrl Pts',(45.7596408825485,-7.6257233326379,143.7517794149));
#158336=CARTESIAN_POINT('Ctrl Pts',(45.7480663165466,-7.59844081559175,
143.62667668098));
#158337=CARTESIAN_POINT('Ctrl Pts',(45.7444886020521,-7.58913672710442,
143.586151562286));
#158338=CARTESIAN_POINT('Ctrl Pts',(45.737819455117,-7.57029207910011,143.507437894518));
#158339=CARTESIAN_POINT('Ctrl Pts',(45.7345929734825,-7.56030305028397,
143.467514656276));
#158340=CARTESIAN_POINT('Ctrl Pts',(45.7263484282852,-7.53292686773121,
143.361620720427));
#158341=CARTESIAN_POINT('Ctrl Pts',(45.7209182165448,-7.512317140153,143.286466775378));
#158342=CARTESIAN_POINT('Ctrl Pts',(45.7133201123482,-7.47677089169681,
143.167336673486));
#158343=CARTESIAN_POINT('Ctrl Pts',(45.7096587513103,-7.45783790075944,
143.106174761609));
#158344=CARTESIAN_POINT('Ctrl Pts',(45.7062958499248,-7.43694281070744,
143.042730367685));
#158345=CARTESIAN_POINT('Ctrl Pts',(45.7041309931867,-7.42255085999889,
142.999941895134));
#158346=CARTESIAN_POINT('Ctrl Pts',(45.7031826442293,-7.41585694488886,
142.980392066024));
#158347=CARTESIAN_POINT('Ctrl Pts',(45.6977051259425,-7.37383780134823,
142.86054559507));
#158348=CARTESIAN_POINT('Ctrl Pts',(45.6948246180137,-7.34029306004632,
142.773887831552));
#158349=CARTESIAN_POINT('Ctrl Pts',(45.691770042583,-7.29243658114092,142.656955627243));
#158350=CARTESIAN_POINT('Ctrl Pts',(45.690965722722,-7.27688780244582,142.620152809729));
#158351=CARTESIAN_POINT('Ctrl Pts',(45.6899804795069,-7.25440829956244,
142.568108874407));
#158352=CARTESIAN_POINT('Ctrl Pts',(45.6895433986862,-7.2433789219476,142.54287697546));
#158353=CARTESIAN_POINT('Ctrl Pts',(45.6891729752481,-7.23270513479341,
142.518811333593));
#158354=CARTESIAN_POINT('Ctrl Pts',(45.6889391217653,-7.22567243480026,
142.503024679245));
#158355=CARTESIAN_POINT('Ctrl Pts',(45.6888111605613,-7.22162158141484,
142.493977594143));
#158356=CARTESIAN_POINT('Ctrl Pts',(45.6880272138865,-7.19592616713251,
142.436783185656));
#158357=CARTESIAN_POINT('Ctrl Pts',(45.6872649054086,-7.16711518274869,
142.373531033505));
#158358=CARTESIAN_POINT('Ctrl Pts',(45.6869970866555,-7.1124947649413,142.261419388534));
#158359=CARTESIAN_POINT('Ctrl Pts',(45.6870571716022,-7.09237842868069,
142.221184305656));
#158360=CARTESIAN_POINT('Ctrl Pts',(45.6875194253624,-7.05896285169835,
142.156793104236));
#158361=CARTESIAN_POINT('Ctrl Pts',(45.687843822262,-7.04144413250784,142.123588874133));
#158362=CARTESIAN_POINT('Ctrl Pts',(45.6884201262682,-7.01949769659911,
142.08315377698));
#158363=CARTESIAN_POINT('Ctrl Pts',(45.6887133361663,-7.00975907998373,
142.065468995032));
#158364=CARTESIAN_POINT('Ctrl Pts',(45.6889195085684,-7.00319156414997,
142.053601082715));
#158365=CARTESIAN_POINT('Ctrl Pts',(45.6890630123584,-6.99883684277521,
142.045778847938));
#158366=CARTESIAN_POINT('Ctrl Pts',(45.6904048531293,-6.95929473657219,
141.975019900084));
#158367=CARTESIAN_POINT('Ctrl Pts',(45.6921845384018,-6.92005463882973,
141.908007387539));
#158368=CARTESIAN_POINT('Ctrl Pts',(45.6956863675944,-6.85796433617798,
141.807147597128));
#158369=CARTESIAN_POINT('Ctrl Pts',(45.696991894597,-6.83672982750858,141.77346926005));
#158370=CARTESIAN_POINT('Ctrl Pts',(45.6988007920649,-6.80949672370966,
141.731325674698));
#158371=CARTESIAN_POINT('Ctrl Pts',(45.699113663538,-6.80482761333938,141.724122677196));
#158372=CARTESIAN_POINT('Ctrl Pts',(45.7001636123571,-6.78963402102599,
141.70092561296));
#158373=CARTESIAN_POINT('Ctrl Pts',(45.7017539847202,-6.76725055741431,
141.667079480057));
#158374=CARTESIAN_POINT('Ctrl Pts',(45.7033639042665,-6.7461562007986,141.636033786375));
#158375=CARTESIAN_POINT('Ctrl Pts',(45.7065472854106,-6.70584735232583,
141.577556746701));
#158376=CARTESIAN_POINT('Ctrl Pts',(45.7086182735838,-6.6814878045978,141.54338751695));
#158377=CARTESIAN_POINT('Ctrl Pts',(45.7114500524151,-6.64923604612378,
141.498939073594));
#158378=CARTESIAN_POINT('Ctrl Pts',(45.7123488827038,-6.63919837515679,
141.485258043084));
#158379=CARTESIAN_POINT('Ctrl Pts',(45.7134002324388,-6.62758451559962,
141.469539272868));
#158380=CARTESIAN_POINT('Ctrl Pts',(45.7136497257773,-6.62484064018721,
141.465835629711));
#158381=CARTESIAN_POINT('Ctrl Pts',(45.7138335799324,-6.62281422693999,
141.463099121855));
#158382=CARTESIAN_POINT('Ctrl Pts',(45.7141373124748,-6.61945076661083,
141.458550380537));
#158383=CARTESIAN_POINT('Ctrl Pts',(45.7145264540736,-6.61511155314601,
141.452673412528));
#158384=CARTESIAN_POINT('Ctrl Pts',(45.7160229518845,-6.59845306229987,
141.430154955935));
#158385=CARTESIAN_POINT('Ctrl Pts',(45.7178479254177,-6.57813305522803,
141.402739126245));
#158386=CARTESIAN_POINT('Ctrl Pts',(45.7218380877348,-6.53630340439622,
141.348305743493));
#158387=CARTESIAN_POINT('Ctrl Pts',(45.7233789981059,-6.52046270551198,
141.327948884204));
#158388=CARTESIAN_POINT('Ctrl Pts',(45.7260617700661,-6.49369965360933,
141.294250513101));
#158389=CARTESIAN_POINT('Ctrl Pts',(45.7274961568459,-6.47956716151472,
141.276611176011));
#158390=CARTESIAN_POINT('Ctrl Pts',(45.7293458160154,-6.46172641248284,
141.254690011814));
#158391=CARTESIAN_POINT('Ctrl Pts',(45.7303164674517,-6.45246268687009,
141.243399581771));
#158392=CARTESIAN_POINT('Ctrl Pts',(45.7307424708742,-6.44841838679609,
141.238490762029));
#158393=CARTESIAN_POINT('Ctrl Pts',(45.7310287190181,-6.44570565034031,
141.235202715874));
#158394=CARTESIAN_POINT('Ctrl Pts',(45.7312503885032,-6.44360985675879,
141.232667182809));
#158395=CARTESIAN_POINT('Ctrl Pts',(45.7400169956866,-6.36082037669196,
141.132598362081));
#158396=CARTESIAN_POINT('Ctrl Pts',(45.7508279851103,-6.26573217913631,
141.024864807299));
#158397=CARTESIAN_POINT('Ctrl Pts',(45.7712367072148,-6.10013641485336,
140.855713182854));
#158398=CARTESIAN_POINT('Ctrl Pts',(45.7787367562556,-6.0411081552893,140.798076114454));
#158399=CARTESIAN_POINT('Ctrl Pts',(45.7911281773601,-5.94639684561445,
140.710486101705));
#158400=CARTESIAN_POINT('Ctrl Pts',(45.7976087465152,-5.8974994790897,140.666408991859));
#158401=CARTESIAN_POINT('Ctrl Pts',(45.8056828955101,-5.83766901096797,
140.614671644116));
#158402=CARTESIAN_POINT('Ctrl Pts',(45.8098496909852,-5.80704790930028,
140.588748214596));
#158403=CARTESIAN_POINT('Ctrl Pts',(45.8119656691689,-5.79155967192321,
140.575775820276));
#158404=CARTESIAN_POINT('Ctrl Pts',(45.8128795129233,-5.78488365189796,
140.570214260568));
#158405=CARTESIAN_POINT('Ctrl Pts',(45.8134902982546,-5.78042446799032,
140.566506154555));
#158406=CARTESIAN_POINT('Ctrl Pts',(45.8139419819895,-5.77712962556911,
140.563772785789));
#158407=CARTESIAN_POINT('Ctrl Pts',(45.8192693889668,-5.73828518183523,
140.531587282574));
#158408=CARTESIAN_POINT('Ctrl Pts',(45.825943633586,-5.68988489649699,140.492257824353));
#158409=CARTESIAN_POINT('Ctrl Pts',(45.8385455597466,-5.59991727629164,
140.423130510986));
#158410=CARTESIAN_POINT('Ctrl Pts',(45.8431787050888,-5.56702917127515,
140.398408932811));
#158411=CARTESIAN_POINT('Ctrl Pts',(45.8508194009384,-5.51316147609579,
140.35915507419));
#158412=CARTESIAN_POINT('Ctrl Pts',(45.8534813793313,-5.49444964359847,
140.345709308676));
#158413=CARTESIAN_POINT('Ctrl Pts',(45.8590425368407,-5.45548061424916,
140.318160471314));
#158414=CARTESIAN_POINT('Ctrl Pts',(45.8620980256864,-5.43413471853736,
140.303312692143));
#158415=CARTESIAN_POINT('Ctrl Pts',(45.8764235136232,-5.33434004698192,
140.235050331361));
#158416=CARTESIAN_POINT('Ctrl Pts',(45.8869093654876,-5.26225278333579,
140.189348452813));
#158417=CARTESIAN_POINT('Ctrl Pts',(45.9008095038559,-5.16718733759057,
140.131782210991));
#158418=CARTESIAN_POINT('Ctrl Pts',(45.9051402261405,-5.13767045970881,
140.11443064948));
#158419=CARTESIAN_POINT('Ctrl Pts',(45.9111524852506,-5.09678449221605,
140.090917922924));
#158420=CARTESIAN_POINT('Ctrl Pts',(45.9140378013058,-5.07718838456376,
140.079790802148));
#158421=CARTESIAN_POINT('Ctrl Pts',(45.9171874191562,-5.05583253773055,
140.067863841893));
#158422=CARTESIAN_POINT('Ctrl Pts',(45.9184903686662,-5.0470051275582,140.062973711995));
#158423=CARTESIAN_POINT('Ctrl Pts',(45.9193485312138,-5.04119268215965,
140.059762333137));
#158424=CARTESIAN_POINT('Ctrl Pts',(45.9196130476279,-5.03940128342387,
140.058773735075));
#158425=CARTESIAN_POINT('Ctrl Pts',(45.9571775476616,-4.78510952048925,
139.919026012772));
#158426=CARTESIAN_POINT('Ctrl Pts',(45.9983852910152,-4.51174191713301,
139.800717395929));
#158427=CARTESIAN_POINT('Ctrl Pts',(46.04178901647,-4.21831693899752,139.70882561586));
#158428=CARTESIAN_POINT('Ctrl Pts',(46.6311525941371,-7.22655631911563,
147.84836866603));
#158429=CARTESIAN_POINT('Ctrl Pts',(46.5749523425034,-7.28654605238906,
147.652930322284));
#158430=CARTESIAN_POINT('Ctrl Pts',(46.5201920540669,-7.34187891713897,
147.457811989727));
#158431=CARTESIAN_POINT('Ctrl Pts',(46.4669881862245,-7.39272369123276,
147.263294848322));
#158432=CARTESIAN_POINT('Ctrl Pts',(46.4117038947351,-7.44555664164975,
147.061171529451));
#158433=CARTESIAN_POINT('Ctrl Pts',(46.3580998832002,-7.49354395600487,
146.859697404632));
#158434=CARTESIAN_POINT('Ctrl Pts',(46.3062558753462,-7.53690360083462,
146.659141512676));
#158435=CARTESIAN_POINT('Ctrl Pts',(46.2906808817071,-7.54992971938474,
146.598890446625));
#158436=CARTESIAN_POINT('Ctrl Pts',(46.2752645598976,-7.56253823447593,
146.538721942065));
#158437=CARTESIAN_POINT('Ctrl Pts',(46.2600086377472,-7.57473518779224,
146.478642508045));
#158438=CARTESIAN_POINT('Ctrl Pts',(46.2222544574842,-7.60491926775972,
146.32996255545));
#158439=CARTESIAN_POINT('Ctrl Pts',(46.1854830765979,-7.63258269512805,
146.181829353134));
#158440=CARTESIAN_POINT('Ctrl Pts',(46.1497151458197,-7.65781587554136,
146.034369942548));
#158441=CARTESIAN_POINT('',(2.89423390144577,-0.0343503973693096,140.227423469835));
#158442=CARTESIAN_POINT('',(-0.413763883134335,-0.0343503924582198,121.466835774864));
#158443=CARTESIAN_POINT('',(1.71342629329879,-0.0343503924582184,133.530730749341));
#158444=CARTESIAN_POINT('Ctrl Pts',(2.89423390144145,-0.0343503973693145,
140.227423469823));
#158445=CARTESIAN_POINT('Ctrl Pts',(2.89490682052228,-0.462029070005339,
140.227304815406));
#158446=CARTESIAN_POINT('Ctrl Pts',(2.89460237971182,-0.917705420464532,
140.140419107162));
#158447=CARTESIAN_POINT('Ctrl Pts',(2.88567038560036,-1.75510442296394,
139.789430687949));
#158448=CARTESIAN_POINT('Ctrl Pts',(2.87635083480166,-2.13688745377311,
139.525490015263));
#158449=CARTESIAN_POINT('Ctrl Pts',(2.83941701094823,-2.73970894382591,
138.919770610805));
#158450=CARTESIAN_POINT('Ctrl Pts',(2.80921594987279,-3.00119474164409,
138.537367096412));
#158451=CARTESIAN_POINT('Ctrl Pts',(2.71482824727497,-3.34831581410866,
137.70361918511));
#158452=CARTESIAN_POINT('Ctrl Pts',(2.64987594375213,-3.43391381428035,
137.252346126911));
#158453=CARTESIAN_POINT('Ctrl Pts',(2.501341302863,-3.43391381428035,136.409964318453));
#158454=CARTESIAN_POINT('Ctrl Pts',(2.40803202714239,-3.34831581410866,
135.963691359544));
#158455=CARTESIAN_POINT('Ctrl Pts',(2.21156887464543,-3.00119474164409,
135.147942104127));
#158456=CARTESIAN_POINT('Ctrl Pts',(2.10915888407688,-2.73970894382592,
134.778270972251));
#158457=CARTESIAN_POINT('Ctrl Pts',(1.93669708828159,-2.13688745377311,
134.196448805887));
#158458=CARTESIAN_POINT('Ctrl Pts',(1.85518157469485,-1.75510442296394,
133.94523822934));
#158459=CARTESIAN_POINT('Ctrl Pts',(1.74352979420513,-0.917705420464523,
133.612362079917));
#158460=CARTESIAN_POINT('Ctrl Pts',(1.71409921239068,-0.4620290650944,133.530612095549));
#158461=CARTESIAN_POINT('Ctrl Pts',(1.71342629329879,-0.0343503924582188,
133.530730749341));
#158462=CARTESIAN_POINT('',(1.38116159371226,-0.0343503924582198,131.646363999275));
#158463=CARTESIAN_POINT('',(-0.413763883134335,-0.0343503924582198,121.466835774864));
#158464=CARTESIAN_POINT('',(21.0799238088015,-21.4999725592973,119.352372629494));
#158465=CARTESIAN_POINT('Origin',(21.0460952759711,4.44089209850063E-15,
119.358337512575));
#158466=CARTESIAN_POINT('',(21.0122667431774,21.4999725592974,119.364302395616));
#158467=CARTESIAN_POINT('Origin',(21.0460952759615,-9.02974887056722E-15,
119.358337512554));
#158468=CARTESIAN_POINT('Origin',(21.0460952759711,4.44089209850063E-15,
119.358337512575));
#158469=CARTESIAN_POINT('Ctrl Pts',(1.71342629329879,-0.0343503924582162,
133.530730749341));
#158470=CARTESIAN_POINT('Ctrl Pts',(1.7127533742069,0.393328280177966,133.530849403133));
#158471=CARTESIAN_POINT('Ctrl Pts',(1.74074994280215,0.849049561642535,
133.612852242722));
#158472=CARTESIAN_POINT('Ctrl Pts',(1.84976630355433,1.68661093518625,133.94619308775));
#158473=CARTESIAN_POINT('Ctrl Pts',(1.93008022417292,2.06850914312402,134.197615537557));
#158474=CARTESIAN_POINT('Ctrl Pts',(2.10064469350225,2.6715474277491,134.779772253768));
#158475=CARTESIAN_POINT('Ctrl Pts',(2.20223164676253,2.93314903787896,135.149588509328));
#158476=CARTESIAN_POINT('Ctrl Pts',(2.39760220552714,3.28043393904487,135.965530418499));
#158477=CARTESIAN_POINT('Ctrl Pts',(2.49064204597367,3.36607750679975,136.411850886116));
#158478=CARTESIAN_POINT('Ctrl Pts',(2.56490936641823,3.36607750679975,136.833041790345));
#158479=CARTESIAN_POINT('Ctrl Pts',(2.63917668686279,3.36607750679975,137.254232694574));
#158480=CARTESIAN_POINT('Ctrl Pts',(2.70439842565971,3.28043393904489,137.705458244064));
#158481=CARTESIAN_POINT('Ctrl Pts',(2.79987872198988,2.93314903787895,138.539013501613));
#158482=CARTESIAN_POINT('Ctrl Pts',(2.83090282037359,2.6715474277491,138.921271892322));
#158483=CARTESIAN_POINT('Ctrl Pts',(2.86973397069298,2.06850914312402,139.526656746933));
#158484=CARTESIAN_POINT('Ctrl Pts',(2.88025511445985,1.68661093518626,139.790385546358));
#158485=CARTESIAN_POINT('Ctrl Pts',(2.89182252830886,0.849049561642544,
140.140909269967));
#158486=CARTESIAN_POINT('Ctrl Pts',(2.89356098234184,0.393328280177964,
140.227542123616));
#158487=CARTESIAN_POINT('Ctrl Pts',(2.89423390143373,-0.0343503924582163,
140.227423469824));
#158488=CARTESIAN_POINT('',(46.1255152751644,7.72197159682826,146.038637027215));
#158489=CARTESIAN_POINT('Ctrl Pts',(46.1255152751644,7.72197159682826,146.038637027215));
#158490=CARTESIAN_POINT('Ctrl Pts',(46.183994384387,7.68085770665526,146.279171780814));
#158491=CARTESIAN_POINT('Ctrl Pts',(46.2451773117493,7.6332659101491,146.52149373214));
#158492=CARTESIAN_POINT('Ctrl Pts',(46.3089515198577,7.57882968383795,146.765090549348));
#158493=CARTESIAN_POINT('Ctrl Pts',(46.3705589150633,7.52624300017179,147.000410843142));
#158494=CARTESIAN_POINT('Ctrl Pts',(46.4345846392306,7.46726902673398,147.236920819104));
#158495=CARTESIAN_POINT('Ctrl Pts',(46.5008817904809,7.40156269285372,147.4741666267));
#158496=CARTESIAN_POINT('Ctrl Pts',(46.5360620153873,7.36669598199073,147.600059831942));
#158497=CARTESIAN_POINT('Ctrl Pts',(46.571881048459,7.32993330205662,147.726160374427));
#158498=CARTESIAN_POINT('Ctrl Pts',(46.6083112377426,7.29122142518356,147.852401444788));
#158499=CARTESIAN_POINT('',(46.0284016907478,4.28565939879059,139.711186162701));
#158500=CARTESIAN_POINT('Ctrl Pts',(46.0284016907478,4.28565939879059,139.711186162701));
#158501=CARTESIAN_POINT('Ctrl Pts',(46.009451892876,4.41100978518104,139.750554627543));
#158502=CARTESIAN_POINT('Ctrl Pts',(45.9896428349026,4.54135926216652,139.797642870725));
#158503=CARTESIAN_POINT('Ctrl Pts',(45.9692247694648,4.67560735556524,139.854095719192));
#158504=CARTESIAN_POINT('Ctrl Pts',(45.9590157367459,4.7427314022646,139.882322143426));
#158505=CARTESIAN_POINT('Ctrl Pts',(45.9486567169092,4.81082554163191,139.912892067642));
#158506=CARTESIAN_POINT('Ctrl Pts',(45.9381949514543,4.87972100603375,139.946021991183));
#158507=CARTESIAN_POINT('Ctrl Pts',(45.9329640687268,4.91416873823467,139.962586952953));
#158508=CARTESIAN_POINT('Ctrl Pts',(45.9277077024198,4.94881617101466,139.979791741817));
#158509=CARTESIAN_POINT('Ctrl Pts',(45.922433052648,4.98363888587044,139.99766286594));
#158510=CARTESIAN_POINT('Ctrl Pts',(45.9177959001256,5.01425290708772,140.013374075573));
#158511=CARTESIAN_POINT('Ctrl Pts',(45.9129814428359,5.04609222585267,140.030196196397));
#158512=CARTESIAN_POINT('Ctrl Pts',(45.908425332391,5.07626481501438,140.04657579581));
#158513=CARTESIAN_POINT('Ctrl Pts',(45.9077989764833,5.08041282233302,140.048827597864));
#158514=CARTESIAN_POINT('Ctrl Pts',(45.9071775807259,5.08452934809361,140.051071022753));
#158515=CARTESIAN_POINT('Ctrl Pts',(45.9065623496373,5.08860689606862,140.053302021474));
#158516=CARTESIAN_POINT('Ctrl Pts',(45.8862006710659,5.22355736064531,140.127139120553));
#158517=CARTESIAN_POINT('Ctrl Pts',(45.8666105311921,5.35404529556136,140.20707833822));
#158518=CARTESIAN_POINT('Ctrl Pts',(45.8480731697131,5.47967188638401,140.292630687702));
#158519=CARTESIAN_POINT('Ctrl Pts',(45.8388044889737,5.54248518179534,140.335406862442));
#158520=CARTESIAN_POINT('Ctrl Pts',(45.8297989417253,5.60408474185784,140.379586566384));
#158521=CARTESIAN_POINT('Ctrl Pts',(45.821090801588,5.66442993465207,140.425110148166));
#158522=CARTESIAN_POINT('Ctrl Pts',(45.8167367315194,5.69460253104918,140.447871939057));
#158523=CARTESIAN_POINT('Ctrl Pts',(45.8124569345293,5.72446213510723,140.470970159996));
#158524=CARTESIAN_POINT('Ctrl Pts',(45.8082558796439,5.75400203758663,140.494395532349));
#158525=CARTESIAN_POINT('Ctrl Pts',(45.8061553522012,5.76877198882632,140.506108218525));
#158526=CARTESIAN_POINT('Ctrl Pts',(45.8040745109114,5.78346201486672,140.517902692444));
#158527=CARTESIAN_POINT('Ctrl Pts',(45.8020139522343,5.7980709928589,140.529777516931));
#158528=CARTESIAN_POINT('Ctrl Pts',(45.8009836728958,5.805375481855,140.535714929175));
#158529=CARTESIAN_POINT('Ctrl Pts',(45.7999584643093,5.81265970884927,140.541672429043));
#158530=CARTESIAN_POINT('Ctrl Pts',(45.7989383976504,5.81992356232579,140.54764986147));
#158531=CARTESIAN_POINT('Ctrl Pts',(45.798428364321,5.82355548906404,140.550638577684));
#158532=CARTESIAN_POINT('Ctrl Pts',(45.7979196164765,5.82718232242351,140.553632277037));
#158533=CARTESIAN_POINT('Ctrl Pts',(45.7974121631645,5.83080404735202,140.55663093907));
#158534=CARTESIAN_POINT('Ctrl Pts',(45.7969047098525,5.83442577228053,140.559629601103));
#158535=CARTESIAN_POINT('Ctrl Pts',(45.7965205363705,5.83716976420411,140.561906282869));
#158536=CARTESIAN_POINT('Ctrl Pts',(45.7958936958764,5.84165388185056,140.565641792772));
#158537=CARTESIAN_POINT('Ctrl Pts',(45.7806100795712,5.95098557663157,140.656720943858));
#158538=CARTESIAN_POINT('Ctrl Pts',(45.7666915407109,6.05363275282939,140.750035584638));
#158539=CARTESIAN_POINT('Ctrl Pts',(45.7541788910299,6.14992992876353,140.844616000562));
#158540=CARTESIAN_POINT('Ctrl Pts',(45.7412877000483,6.2491403532217,140.942057728403));
#158541=CARTESIAN_POINT('Ctrl Pts',(45.7298886223451,6.3416109033887,141.040842998358));
#158542=CARTESIAN_POINT('Ctrl Pts',(45.7199718226298,6.42769967331016,141.139921000597));
#158543=CARTESIAN_POINT('Ctrl Pts',(45.7142480946429,6.47738795137442,141.197106337661));
#158544=CARTESIAN_POINT('Ctrl Pts',(45.7090171683938,6.52495010581967,141.254389367596));
#158545=CARTESIAN_POINT('Ctrl Pts',(45.7042695604774,6.57045361793451,141.311569384902));
#158546=CARTESIAN_POINT('Ctrl Pts',(45.6959999643079,6.64971367396863,141.411168100804));
#158547=CARTESIAN_POINT('Ctrl Pts',(45.6891813300088,6.72277528512748,141.510435605595));
#158548=CARTESIAN_POINT('Ctrl Pts',(45.6836775820624,6.79018167418363,141.608430686704));
#158549=CARTESIAN_POINT('Ctrl Pts',(45.6822073808803,6.80818775909815,141.634607845522));
#158550=CARTESIAN_POINT('Ctrl Pts',(45.6808307273227,6.82579023568006,141.66069425717));
#158551=CARTESIAN_POINT('Ctrl Pts',(45.6795444407347,6.84299930990636,141.686672084303));
#158552=CARTESIAN_POINT('Ctrl Pts',(45.6764936687251,6.88381522328763,141.748285435967));
#158553=CARTESIAN_POINT('Ctrl Pts',(45.6739516782181,6.92242270120041,141.809296108042));
#158554=CARTESIAN_POINT('Ctrl Pts',(45.67187119573,6.95897798206324,141.869511322291));
#158555=CARTESIAN_POINT('Ctrl Pts',(45.6708309544859,6.97725562249465,141.899618929415));
#158556=CARTESIAN_POINT('Ctrl Pts',(45.6699059875799,6.99502036582419,141.92952811241));
#158557=CARTESIAN_POINT('Ctrl Pts',(45.6690898210906,7.01229252155032,141.959217281051));
#158558=CARTESIAN_POINT('Ctrl Pts',(45.668681737846,7.02092859941338,141.974061865372));
#158559=CARTESIAN_POINT('Ctrl Pts',(45.6683008482816,7.02944152814726,141.988851447237));
#158560=CARTESIAN_POINT('Ctrl Pts',(45.6679463130868,7.03783389502715,142.003583500307));
#158561=CARTESIAN_POINT('Ctrl Pts',(45.6677690454893,7.0420300784671,142.010949526842));
#158562=CARTESIAN_POINT('Ctrl Pts',(45.6675983660977,7.04619612131013,142.018301171247));
#158563=CARTESIAN_POINT('Ctrl Pts',(45.6674341680494,7.05033234744749,142.025638122581));
#158564=CARTESIAN_POINT('Ctrl Pts',(45.6672699700011,7.05446857358485,142.032975073916));
#158565=CARTESIAN_POINT('Ctrl Pts',(45.667138694479,7.05786270423485,142.039020679768));
#158566=CARTESIAN_POINT('Ctrl Pts',(45.6669609097315,7.06265190001152,142.047604589381));
#158567=CARTESIAN_POINT('Ctrl Pts',(45.6643797133639,7.13218460690298,142.17223145763));
#158568=CARTESIAN_POINT('Ctrl Pts',(45.6632752867041,7.19971530774337,142.303556493107));
#158569=CARTESIAN_POINT('Ctrl Pts',(45.6642598432247,7.26386732472425,142.441753873634));
#158570=CARTESIAN_POINT('Ctrl Pts',(45.6643602975754,7.27041275820106,142.455854159229));
#158571=CARTESIAN_POINT('Ctrl Pts',(45.664482539201,7.27692303529989,142.470025979662));
#158572=CARTESIAN_POINT('Ctrl Pts',(45.6646272451483,7.28339670455111,142.484269515212));
#158573=CARTESIAN_POINT('Ctrl Pts',(45.6658824739582,7.33955152264681,142.6078228073));
#158574=CARTESIAN_POINT('Ctrl Pts',(45.6688648672261,7.39326350094975,142.737656382104));
#158575=CARTESIAN_POINT('Ctrl Pts',(45.6739949548805,7.4426081922518,142.871601936082));
#158576=CARTESIAN_POINT('Ctrl Pts',(45.6752527010066,7.45470605461057,142.904441433763));
#158577=CARTESIAN_POINT('Ctrl Pts',(45.6766397732845,7.46654149812806,142.937528055851));
#158578=CARTESIAN_POINT('Ctrl Pts',(45.678162778316,7.47808632877853,142.970829776213));
#158579=CARTESIAN_POINT('Ctrl Pts',(45.6842271030676,7.52405571221501,143.103431076202));
#158580=CARTESIAN_POINT('Ctrl Pts',(45.6921579897756,7.56376098479096,143.234237122771));
#158581=CARTESIAN_POINT('Ctrl Pts',(45.7015834264608,7.59812982795002,143.362462267337));
#158582=CARTESIAN_POINT('Ctrl Pts',(45.7041801077836,7.60759834766917,143.397787934372));
#158583=CARTESIAN_POINT('Ctrl Pts',(45.7068899336171,7.61666173680026,143.432917765412));
#158584=CARTESIAN_POINT('Ctrl Pts',(45.7097045081294,7.62533917254263,143.467835441451));
#158585=CARTESIAN_POINT('Ctrl Pts',(45.716219968196,7.64542657325434,143.548666388674));
#158586=CARTESIAN_POINT('Ctrl Pts',(45.7232940489111,7.66345579613631,143.628364479795));
#158587=CARTESIAN_POINT('Ctrl Pts',(45.730825190822,7.67966776014608,143.706779012972));
#158588=CARTESIAN_POINT('Ctrl Pts',(45.7345907617774,7.68777374215096,143.745986279561));
#158589=CARTESIAN_POINT('Ctrl Pts',(45.7384706822679,7.69542519551929,143.784873283985));
#158590=CARTESIAN_POINT('Ctrl Pts',(45.7424527782053,7.70265099123863,143.82342473189));
#158591=CARTESIAN_POINT('Ctrl Pts',(45.744443826174,7.7062638890983,143.842700455843));
#158592=CARTESIAN_POINT('Ctrl Pts',(45.7464604132963,7.70977037069837,143.861892291497));
#158593=CARTESIAN_POINT('Ctrl Pts',(45.7485010660626,7.713173954904,143.880998580289));
#158594=CARTESIAN_POINT('Ctrl Pts',(45.750541718829,7.71657753910963,143.900104869082));
#158595=CARTESIAN_POINT('Ctrl Pts',(45.7523875871807,7.71954259370185,143.91714049923));
#158596=CARTESIAN_POINT('Ctrl Pts',(45.754693733771,7.72307952403362,143.938059155794));
#158597=CARTESIAN_POINT('Ctrl Pts',(45.7740222053368,7.7527235447722,144.113384375925));
#158598=CARTESIAN_POINT('Ctrl Pts',(45.7967147306483,7.77509870425236,144.29208668924));
#158599=CARTESIAN_POINT('Ctrl Pts',(45.8228388932108,7.78980599766508,144.473167914215));
#158600=CARTESIAN_POINT('Ctrl Pts',(45.8480458992102,7.80399695335224,144.647891812575));
#158601=CARTESIAN_POINT('Ctrl Pts',(45.8764481162649,7.81104914922233,144.824830466553));
#158602=CARTESIAN_POINT('Ctrl Pts',(45.9080636557945,7.81058759439462,145.003094689877));
#158603=CARTESIAN_POINT('Ctrl Pts',(45.9384234946378,7.810144371524,145.174278644735));
#158604=CARTESIAN_POINT('Ctrl Pts',(45.971746665868,7.8027724802356,145.346684928471));
#158605=CARTESIAN_POINT('Ctrl Pts',(46.0080057877663,7.78812270517353,145.519533808147));
#158606=CARTESIAN_POINT('Ctrl Pts',(46.0442649096645,7.77347293011147,145.692382687822));
#158607=CARTESIAN_POINT('Ctrl Pts',(46.0834604821633,7.75154542668907,145.865674075287));
#158608=CARTESIAN_POINT('Ctrl Pts',(46.1255152751644,7.72197159682826,146.038637027215));
#158609=CARTESIAN_POINT('Ctrl Pts',(46.3509510310085,0.0343504322637197,
139.055898541659));
#158610=CARTESIAN_POINT('Ctrl Pts',(46.3505517348952,0.289138438632088,
139.055978266158));
#158611=CARTESIAN_POINT('Ctrl Pts',(46.346783451412,0.54593555688485,139.063076026948));
#158612=CARTESIAN_POINT('Ctrl Pts',(46.3394906583825,0.804246151701623,
139.077400049602));
#158613=CARTESIAN_POINT('Ctrl Pts',(46.3322349286742,1.06124396436419,139.091651274927));
#158614=CARTESIAN_POINT('Ctrl Pts',(46.3214903244831,1.31973962955468,139.113055515702));
#158615=CARTESIAN_POINT('Ctrl Pts',(46.3071533183797,1.57923398323097,139.141809086788));
#158616=CARTESIAN_POINT('Ctrl Pts',(46.2928958374792,1.83728896100349,139.170403166166));
#158617=CARTESIAN_POINT('Ctrl Pts',(46.2750856444827,2.09633129025598,139.206265280019));
#158618=CARTESIAN_POINT('Ctrl Pts',(46.2536712542073,2.35586335520789,139.249579620141));
#158619=CARTESIAN_POINT('Ctrl Pts',(46.2323093671487,2.61475910653701,139.292787763347));
#158620=CARTESIAN_POINT('Ctrl Pts',(46.2073608959045,2.87414190315989,139.343411642094));
#158621=CARTESIAN_POINT('Ctrl Pts',(46.1788256748232,3.13351541783259,139.401625114299));
#158622=CARTESIAN_POINT('Ctrl Pts',(46.1503563543616,3.39228992276671,139.459704145495));
#158623=CARTESIAN_POINT('Ctrl Pts',(46.1183168315074,3.65105489450121,139.525337755125));
#158624=CARTESIAN_POINT('Ctrl Pts',(46.0827580021033,3.90931946967923,139.598689596019));
#158625=CARTESIAN_POINT('Ctrl Pts',(46.0654671907504,4.03490302018918,139.634357610533));
#158626=CARTESIAN_POINT('Ctrl Pts',(46.047345015463,4.16036831109744,139.671850450518));
#158627=CARTESIAN_POINT('Ctrl Pts',(46.0284016907478,4.28565939879059,139.711186162701));
#158628=CARTESIAN_POINT('Origin',(10.4384266411762,-0.0270045052801676,
156.534945497534));
#158629=CARTESIAN_POINT('',(48.9375087269424,-4.00018398478067,142.087510868902));
#158630=CARTESIAN_POINT('',(49.3053711741162,0.0383111611405328,141.534954558003));
#158631=CARTESIAN_POINT('Ctrl Pts',(48.9375087304962,-4.00018624765936,
142.087502763741));
#158632=CARTESIAN_POINT('Ctrl Pts',(48.9949833354212,-3.68955343570011,
142.000798941664));
#158633=CARTESIAN_POINT('Ctrl Pts',(49.0457220209274,-3.37742578915628,
141.924471192877));
#158634=CARTESIAN_POINT('Ctrl Pts',(49.0897258950434,-3.06450751067134,
141.858426739305));
#158635=CARTESIAN_POINT('Ctrl Pts',(49.1341269388833,-2.74876489753937,
141.791786182368));
#158636=CARTESIAN_POINT('Ctrl Pts',(49.1716710490429,-2.43221753600664,
141.735615251058));
#158637=CARTESIAN_POINT('Ctrl Pts',(49.2023593250218,-2.11556420125793,
141.689771614418));
#158638=CARTESIAN_POINT('Ctrl Pts',(49.233208589264,-1.7972497282135,141.643687485694));
#158639=CARTESIAN_POINT('Ctrl Pts',(49.2571299006305,-1.47882835832807,
141.60803910677));
#158640=CARTESIAN_POINT('Ctrl Pts',(49.2741243321198,-1.16098201742068,
141.582637047908));
#158641=CARTESIAN_POINT('Ctrl Pts',(49.2912478117602,-0.840722092827111,
141.557042097114));
#158642=CARTESIAN_POINT('Ctrl Pts',(49.3013388131149,-0.521046152281689,
141.541849489902));
#158643=CARTESIAN_POINT('Ctrl Pts',(49.3043983848133,-0.20262062689389,
141.536822739548));
#158644=CARTESIAN_POINT('Ctrl Pts',(49.3051708417072,-0.122227023957362,
141.535553624669));
#158645=CARTESIAN_POINT('Ctrl Pts',(49.305495099357,-0.0419129635884498,
141.534932300882));
#158646=CARTESIAN_POINT('Ctrl Pts',(49.3053711741162,0.0383111611405328,
141.534954558003));
#158647=CARTESIAN_POINT('',(48.9248217570406,4.07524464379169,142.089728903236));
#158648=CARTESIAN_POINT('Ctrl Pts',(49.3053711741162,0.0383111611405328,
141.534954558003));
#158649=CARTESIAN_POINT('Ctrl Pts',(49.3048343231318,0.372806541263403,
141.535047359322));
#158650=CARTESIAN_POINT('Ctrl Pts',(49.296501913863,0.708834768942396,141.546333420866));
#158651=CARTESIAN_POINT('Ctrl Pts',(49.2803751560891,1.0456269205789,141.569098282739));
#158652=CARTESIAN_POINT('Ctrl Pts',(49.2651845064688,1.36286933483779,141.590541715151));
#158653=CARTESIAN_POINT('Ctrl Pts',(49.2430781218927,1.68078908219588,141.62216982411));
#158654=CARTESIAN_POINT('Ctrl Pts',(49.2140570630999,1.99871197485721,141.664179276538));
#158655=CARTESIAN_POINT('Ctrl Pts',(49.1851901179431,2.31494656753981,141.705965641673));
#158656=CARTESIAN_POINT('Ctrl Pts',(49.1494817433335,2.63118408738318,141.758023563724));
#158657=CARTESIAN_POINT('Ctrl Pts',(49.1069330268926,2.9467332676804,141.820503266713));
#158658=CARTESIAN_POINT('Ctrl Pts',(49.0646947262146,3.25998034705143,141.882527146677));
#158659=CARTESIAN_POINT('Ctrl Pts',(49.0157155278959,3.57254888781943,141.954821446331));
#158660=CARTESIAN_POINT('Ctrl Pts',(48.9599965345,3.88373813372928,142.037487896656));
#158661=CARTESIAN_POINT('Ctrl Pts',(48.9485557565992,3.94763460476313,142.054461794431));
#158662=CARTESIAN_POINT('Ctrl Pts',(48.9368308264528,4.01147284724558,142.071872828551));
#158663=CARTESIAN_POINT('Ctrl Pts',(48.924821753789,4.07524667829838,142.089721632632));
#158664=CARTESIAN_POINT('',(94.5819839425882,4.14714157564843,142.089747519112));
#158665=CARTESIAN_POINT('',(48.924821753789,4.07524667829838,142.089721632632));
#158666=CARTESIAN_POINT('',(93.9162870067071,0.108481919349057,141.534966741905));
#158667=CARTESIAN_POINT('Ctrl Pts',(94.5819839479975,4.14713813598916,142.089759812562));
#158668=CARTESIAN_POINT('Ctrl Pts',(94.3592538320324,3.45222469974125,141.895409168734));
#158669=CARTESIAN_POINT('Ctrl Pts',(94.1924301510237,2.7627644869811,141.756622462181));
#158670=CARTESIAN_POINT('Ctrl Pts',(94.0260343534174,1.74942114702695,141.621535163829));
#158671=CARTESIAN_POINT('Ctrl Pts',(93.9845424294768,1.4150798243908,141.588672491858));
#158672=CARTESIAN_POINT('Ctrl Pts',(93.943262545855,0.920005572230557,141.556241959662));
#158673=CARTESIAN_POINT('Ctrl Pts',(93.9278621095087,0.674074769870453,
141.544241726843));
#158674=CARTESIAN_POINT('Ctrl Pts',(93.9190636792179,0.390213915861264,
141.537307403827));
#158675=CARTESIAN_POINT('Ctrl Pts',(93.9169566054853,0.249076665690299,
141.53556754835));
#158676=CARTESIAN_POINT('Ctrl Pts',(93.9164760984515,0.178709844243637,
141.535124545383));
#158677=CARTESIAN_POINT('Ctrl Pts',(93.9163929583916,0.148596247998712,
141.53502564476));
#158678=CARTESIAN_POINT('Ctrl Pts',(93.9163648186267,0.128530249581641,
141.534979865354));
#158679=CARTESIAN_POINT('Ctrl Pts',(93.916366176505,0.117150856258414,141.534966682013));
#158680=CARTESIAN_POINT('Ctrl Pts',(93.9162870067071,0.108481919349057,
141.534966741905));
#158681=CARTESIAN_POINT('',(94.5946916752436,-3.92833378532365,142.087508698775));
#158682=CARTESIAN_POINT('Ctrl Pts',(93.9162870071781,0.108481918637627,
141.53496917311));
#158683=CARTESIAN_POINT('Ctrl Pts',(93.9164305461748,0.00514822670153565,
141.534938907382));
#158684=CARTESIAN_POINT('Ctrl Pts',(93.9179253256695,-0.0987368552810903,
141.535974789762));
#158685=CARTESIAN_POINT('Ctrl Pts',(93.9208317148094,-0.203146342090515,
141.53811584605));
#158686=CARTESIAN_POINT('Ctrl Pts',(93.925388846452,-0.366857308942038,
141.541472958566));
#158687=CARTESIAN_POINT('Ctrl Pts',(93.933415834867,-0.531859595231141,
141.547546324156));
#158688=CARTESIAN_POINT('Ctrl Pts',(93.9450163344638,-0.698040796407542,
141.556450216679));
#158689=CARTESIAN_POINT('Ctrl Pts',(93.9566168340607,-0.864221997583943,
141.565354109202));
#158690=CARTESIAN_POINT('Ctrl Pts',(93.9717910021007,-1.03158290547825,
141.577088579239));
#158691=CARTESIAN_POINT('Ctrl Pts',(93.9906654644376,-1.19996598454483,
141.591788795191));
#158692=CARTESIAN_POINT('Ctrl Pts',(94.0097354656431,-1.37009350730349,
141.606641304944));
#158693=CARTESIAN_POINT('Ctrl Pts',(94.032584612726,-1.54126418678172,141.624521917453));
#158694=CARTESIAN_POINT('Ctrl Pts',(94.0592177093987,-1.71336391385054,
141.64554051154));
#158695=CARTESIAN_POINT('Ctrl Pts',(94.0858508060713,-1.88546364091937,
141.666559105628));
#158696=CARTESIAN_POINT('Ctrl Pts',(94.1162683856671,-2.05849314321545,
141.690715870679));
#158697=CARTESIAN_POINT('Ctrl Pts',(94.1504711301126,-2.23228203059035,
141.718132816551));
#158698=CARTESIAN_POINT('Ctrl Pts',(94.1837144857192,-2.4011961302375,141.744780715603));
#158699=CARTESIAN_POINT('Ctrl Pts',(94.2205347524744,-2.57082605769036,
141.774508809456));
#158700=CARTESIAN_POINT('Ctrl Pts',(94.2608643460002,-2.74110246525793,
141.807426377993));
#158701=CARTESIAN_POINT('Ctrl Pts',(94.2987854901771,-2.90121010921786,
141.838378137068));
#158702=CARTESIAN_POINT('Ctrl Pts',(94.339809638591,-3.06188925156412,141.872150017002));
#158703=CARTESIAN_POINT('Ctrl Pts',(94.3838582501225,-3.22304667840359,
141.908835852476));
#158704=CARTESIAN_POINT('Ctrl Pts',(94.4299695860226,-3.39175084372076,
141.947239625569));
#158705=CARTESIAN_POINT('Ctrl Pts',(94.4793959638611,-3.56097846054621,
141.988836666638));
#158706=CARTESIAN_POINT('Ctrl Pts',(94.5320209407876,-3.73066988997311,
142.033746929427));
#158707=CARTESIAN_POINT('Ctrl Pts',(94.5524331818669,-3.79649001130812,
142.051166777653));
#158708=CARTESIAN_POINT('Ctrl Pts',(94.5733262516347,-3.86237956533525,
142.069085116504));
#158709=CARTESIAN_POINT('Ctrl Pts',(94.5946916751395,-3.92833371710833,
142.0875089431));
#158710=CARTESIAN_POINT('',(48.9375087304962,-4.00018624765936,142.087502763741));
#158711=CARTESIAN_POINT('Origin',(20.7769406005715,-3.80534757440804E-14,
117.831885495454));
#158712=CARTESIAN_POINT('',(11.4514113671306,-17.0269155958486,125.365772183904));
#158713=CARTESIAN_POINT('',(11.3978832029447,16.9933024121131,125.375210643478));
#158714=CARTESIAN_POINT('Origin',(21.7841119891515,-1.2034114792157E-14,
123.543838280654));
#158715=CARTESIAN_POINT('',(2.75313371105733,-0.0319538534495447,130.789059825797));
#158716=CARTESIAN_POINT('Origin',(21.0460952759475,5.19193629061609E-12,
119.358337512588));
#158717=CARTESIAN_POINT('',(3.19063603741116,-0.0319538534495439,133.270258815289));
#158718=CARTESIAN_POINT('',(1.08081067876142,-0.0319538534495447,121.304844616208));
#158719=CARTESIAN_POINT('',(4.37144364554608,-0.0319538534495668,139.966951535772));
#158720=CARTESIAN_POINT('Ctrl Pts',(3.19063603741116,-0.031953853449541,
133.270258815289));
#158721=CARTESIAN_POINT('Ctrl Pts',(3.19130914580987,-0.4597528414267,133.270140128117));
#158722=CARTESIAN_POINT('Ctrl Pts',(3.22179255511482,-0.915479709149352,
133.351752291131));
#158723=CARTESIAN_POINT('Ctrl Pts',(3.33722344804325,-1.75284033660896,
133.683998128254));
#158724=CARTESIAN_POINT('Ctrl Pts',(3.42141457794632,-2.13454361927574,
133.93471892068));
#158725=CARTESIAN_POINT('Ctrl Pts',(3.59892084762791,-2.73722937084846,
134.515522124483));
#158726=CARTESIAN_POINT('Ctrl Pts',(3.7040443169968,-2.9986912819894,134.884637277465));
#158727=CARTESIAN_POINT('Ctrl Pts',(3.90438475055902,-3.34584029838365,
135.699666792464));
#158728=CARTESIAN_POINT('Ctrl Pts',(3.99879634971067,-3.43148439569077,
136.145797224032));
#158729=CARTESIAN_POINT('Ctrl Pts',(4.14737386872942,-3.43148439569077,
136.988422206447));
#158730=CARTESIAN_POINT('Ctrl Pts',(4.21124157983659,-3.34584029838365,
137.439938349572));
#158731=CARTESIAN_POINT('Ctrl Pts',(4.30173966430781,-2.99869128198941,
138.27433603434));
#158732=CARTESIAN_POINT('Ctrl Pts',(4.32920073339708,-2.73722937084846,
138.657145163879));
#158733=CARTESIAN_POINT('Ctrl Pts',(4.36104579664255,-2.13454361927575,
139.263632368418));
#158734=CARTESIAN_POINT('Ctrl Pts',(4.36768357449715,-1.75284033660896,
139.528027909254));
#158735=CARTESIAN_POINT('Ctrl Pts',(4.372848785034,-0.915479709149344,139.87971656123));
#158736=CARTESIAN_POINT('Ctrl Pts',(4.37211675394481,-0.459752841426703,
139.9668328486));
#158737=CARTESIAN_POINT('Ctrl Pts',(4.3714436455461,-0.0319538534495412,
139.966951535772));
#158738=CARTESIAN_POINT('',(6.47258659531382,-0.0319538534495448,151.883125347209));
#158739=CARTESIAN_POINT('',(1.08081067876142,-0.0319538534495447,121.304844616208));
#158740=CARTESIAN_POINT('',(45.86371189171,0.217029124246953,144.937407156988));
#158741=CARTESIAN_POINT('Origin',(26.1687165171315,-2.57311409771171E-14,
148.410166226454));
#158742=CARTESIAN_POINT('Origin',(26.1687165171315,-2.57311409771171E-14,
148.410166226454));
#158743=CARTESIAN_POINT('Ctrl Pts',(4.3714436455461,-0.0319538534495414,
139.966951535772));
#158744=CARTESIAN_POINT('Ctrl Pts',(4.37077053714739,0.39584513452762,139.967070222943));
#158745=CARTESIAN_POINT('Ctrl Pts',(4.37006839073011,0.851620317635747,
139.880206819763));
#158746=CARTESIAN_POINT('Ctrl Pts',(4.36226786195385,1.68915555832631,139.528982845496));
#158747=CARTESIAN_POINT('Ctrl Pts',(4.35442872841004,2.0709827100228,139.264799136081));
#158748=CARTESIAN_POINT('Ctrl Pts',(4.32068673997907,2.67390169638796,138.658646410632));
#158749=CARTESIAN_POINT('Ctrl Pts',(4.29240269482834,2.93548826733316,138.275982393978));
#158750=CARTESIAN_POINT('Ctrl Pts',(4.20081190886385,3.2828137128186,137.441777381964));
#158751=CARTESIAN_POINT('Ctrl Pts',(4.13667461184008,3.36850692538934,136.99030877411));
#158752=CARTESIAN_POINT('Ctrl Pts',(4.06238585233071,3.36850692538934,136.568996282902));
#158753=CARTESIAN_POINT('Ctrl Pts',(3.98809709282133,3.36850692538933,136.147683791695));
#158754=CARTESIAN_POINT('Ctrl Pts',(3.89395507958628,3.28281371281859,135.701505824857));
#158755=CARTESIAN_POINT('Ctrl Pts',(3.69470734751732,2.93548826733316,134.886283637102));
#158756=CARTESIAN_POINT('Ctrl Pts',(3.5904068542099,2.67390169638796,134.517023371236));
#158757=CARTESIAN_POINT('Ctrl Pts',(3.41479750971382,2.0709827100228,133.935885688343));
#158758=CARTESIAN_POINT('Ctrl Pts',(3.33180773549995,1.68915555832632,133.684953064496));
#158759=CARTESIAN_POINT('Ctrl Pts',(3.21901216081092,0.851620317635762,
133.352242549663));
#158760=CARTESIAN_POINT('Ctrl Pts',(3.18996292901245,0.395845134527619,
133.27037750246));
#158761=CARTESIAN_POINT('Ctrl Pts',(3.19063603741116,-0.0319538534495416,
133.270258815289));
#158762=CARTESIAN_POINT('Origin',(21.0460952759475,5.19193629061609E-12,
119.358337512588));
#158763=CARTESIAN_POINT('Origin',(-3.46221193726519,-0.0437048830555943,
137.895785892187));
#158764=CARTESIAN_POINT('',(-2.87180813319772,-0.0437048830555947,141.244132252429));
#158765=CARTESIAN_POINT('Origin',(21.4151041909515,-3.07084035820744E-14,
121.451091063454));
#158766=CARTESIAN_POINT('',(21.0134477487628,20.7493757828742,119.364094152467));
#158767=CARTESIAN_POINT('Origin',(22.4050280472972,0.00237376213208851,
118.509181234833));
#158768=CARTESIAN_POINT('',(21.078742803216,-20.7493757828747,119.352580872643));
#158769=CARTESIAN_POINT('Origin',(21.0460952759615,-1.96166393586405E-14,
119.358337512554));
#158770=CARTESIAN_POINT('Origin',(22.4050280472236,0.00237376205382667,
118.5091812347));
#158771=CARTESIAN_POINT('Origin',(26.1687165171315,-2.57311409771171E-14,
148.410166226454));
#158772=CARTESIAN_POINT('',(44.6470594068091,0.200751938845159,146.675075734032));
#158773=CARTESIAN_POINT('Origin',(44.3865872386167,0.200751939928429,145.197864087198));
#158774=CARTESIAN_POINT('Origin',(26.4291887836315,-2.1219048984176E-14,
149.887377855954));
#158775=CARTESIAN_POINT('Origin',(19.0737828394622,2.73849310306822,149.661194460162));
#158776=CARTESIAN_POINT('',(16.5110267574855,2.73391286221553,151.636217420201));
#158777=CARTESIAN_POINT('',(17.0138492275693,4.37111689096414,151.547556247505));
#158778=CARTESIAN_POINT('Ctrl Pts',(16.5110267574884,2.73391286260886,151.636217420217));
#158779=CARTESIAN_POINT('Ctrl Pts',(16.5109213014316,2.80093627975376,151.636236014965));
#158780=CARTESIAN_POINT('Ctrl Pts',(16.5131087246683,2.86733052016455,151.635850313274));
#158781=CARTESIAN_POINT('Ctrl Pts',(16.5174994497767,2.93316110936568,151.635076109366));
#158782=CARTESIAN_POINT('Ctrl Pts',(16.5219269490194,2.99954305691286,151.634295421181));
#158783=CARTESIAN_POINT('Ctrl Pts',(16.528594872203,3.06535254744676,151.633119685007));
#158784=CARTESIAN_POINT('Ctrl Pts',(16.5374637983434,3.13066082684022,151.63155585318));
#158785=CARTESIAN_POINT('Ctrl Pts',(16.5463769426455,3.1962947163476,151.629984224493));
#158786=CARTESIAN_POINT('Ctrl Pts',(16.5575132097492,3.26142305811755,151.6280206004));
#158787=CARTESIAN_POINT('Ctrl Pts',(16.5708839249923,3.32611207446319,151.625662984223));
#158788=CARTESIAN_POINT('Ctrl Pts',(16.5786271707001,3.36357476356017,151.624297642055));
#158789=CARTESIAN_POINT('Ctrl Pts',(16.587120749502,3.40088994557632,151.622799996355));
#158790=CARTESIAN_POINT('Ctrl Pts',(16.5963744098056,3.43806820585387,151.621168326374));
#158791=CARTESIAN_POINT('Ctrl Pts',(16.6155372509694,3.5150583992551,151.617789400449));
#158792=CARTESIAN_POINT('Ctrl Pts',(16.6378503686473,3.59147349031497,151.613854992147));
#158793=CARTESIAN_POINT('Ctrl Pts',(16.6632921003587,3.6669574847227,151.609368928814));
#158794=CARTESIAN_POINT('Ctrl Pts',(16.6886237454174,3.742114859057,151.604902276727));
#158795=CARTESIAN_POINT('Ctrl Pts',(16.7170570072394,3.81634864986932,151.599888727443));
#158796=CARTESIAN_POINT('Ctrl Pts',(16.7485197474872,3.88930711941047,151.594340998023));
#158797=CARTESIAN_POINT('Ctrl Pts',(16.7792847645072,3.96064764917713,151.588916296021));
#158798=CARTESIAN_POINT('Ctrl Pts',(16.8129461791987,4.03076832487788,151.58298088017));
#158799=CARTESIAN_POINT('Ctrl Pts',(16.8493895442315,4.09934729821385,151.576554931647));
#158800=CARTESIAN_POINT('Ctrl Pts',(16.8864091997694,4.16901073263477,151.570027367559));
#158801=CARTESIAN_POINT('Ctrl Pts',(16.9263312196188,4.23708316156678,151.562988036505));
#158802=CARTESIAN_POINT('Ctrl Pts',(16.9689085232936,4.30331911518685,151.555480501453));
#158803=CARTESIAN_POINT('Ctrl Pts',(16.9835773374774,4.32613885274841,151.552893991102));
#158804=CARTESIAN_POINT('Ctrl Pts',(16.9985611252097,4.34874102035924,151.550251942044));
#158805=CARTESIAN_POINT('Ctrl Pts',(17.0138492253656,4.37111689096524,151.547556235016));
#158806=CARTESIAN_POINT('',(17.7868045912878,5.1371366674824,151.411263364416));
#158807=CARTESIAN_POINT('Ctrl Pts',(17.013849229773,4.37111689096304,151.547556259993));
#158808=CARTESIAN_POINT('Ctrl Pts',(17.0874139946951,4.47878727439227,151.534584809587));
#158809=CARTESIAN_POINT('Ctrl Pts',(17.3140356434103,4.76667060199688,151.494625297278));
#158810=CARTESIAN_POINT('Ctrl Pts',(17.5873714274621,5.00446152832237,151.446428745532));
#158811=CARTESIAN_POINT('Ctrl Pts',(17.7868045798642,5.13713666751144,151.411263299869));
#158812=CARTESIAN_POINT('',(18.605129224176,4.01827646758674,149.770415815628));
#158813=CARTESIAN_POINT('Ctrl Pts',(17.7868045622877,5.13713666742147,151.411263199672));
#158814=CARTESIAN_POINT('Ctrl Pts',(17.8333695830196,5.10000197274449,151.40308003586));
#158815=CARTESIAN_POINT('Ctrl Pts',(17.8786263509401,5.06215449207173,151.39182828418));
#158816=CARTESIAN_POINT('Ctrl Pts',(17.9223569681114,5.02392012874832,151.377571697894));
#158817=CARTESIAN_POINT('Ctrl Pts',(17.9660416539441,4.98572592391336,151.363330085649));
#158818=CARTESIAN_POINT('Ctrl Pts',(18.0082031654458,4.94714599031353,151.346090043535));
#158819=CARTESIAN_POINT('Ctrl Pts',(18.0486598288029,4.90851753398444,151.325950997884));
#158820=CARTESIAN_POINT('Ctrl Pts',(18.089076324385,4.86992743027787,151.305831947471));
#158821=CARTESIAN_POINT('Ctrl Pts',(18.1277911741071,4.83128925917755,151.282819769792));
#158822=CARTESIAN_POINT('Ctrl Pts',(18.1646617998986,4.79294628030214,151.257047778563));
#158823=CARTESIAN_POINT('Ctrl Pts',(18.1819336501171,4.7749847140457,151.244975025177));
#158824=CARTESIAN_POINT('Ctrl Pts',(18.1988013706392,4.75708799228111,151.232297133882));
#158825=CARTESIAN_POINT('Ctrl Pts',(18.2152533744101,4.73929158706959,151.219030266785));
#158826=CARTESIAN_POINT('Ctrl Pts',(18.2457334285694,4.70632080720359,151.194451204364));
#158827=CARTESIAN_POINT('Ctrl Pts',(18.2748346125101,4.67364117953585,151.167807523998));
#158828=CARTESIAN_POINT('Ctrl Pts',(18.302455989941,4.64152037095539,151.139236557104));
#158829=CARTESIAN_POINT('Ctrl Pts',(18.3298880217829,4.60961975173487,151.110861445272));
#158830=CARTESIAN_POINT('Ctrl Pts',(18.3558604017593,4.578270864997,151.080585687432));
#158831=CARTESIAN_POINT('Ctrl Pts',(18.3803128993181,4.5477287180692,151.048578755568));
#158832=CARTESIAN_POINT('Ctrl Pts',(18.4050185665606,4.51687035208604,151.016240438953));
#158833=CARTESIAN_POINT('Ctrl Pts',(18.4281726447028,4.48683609445531,150.982135203747));
#158834=CARTESIAN_POINT('Ctrl Pts',(18.4497537930202,4.45787304836873,150.946469282319));
#158835=CARTESIAN_POINT('Ctrl Pts',(18.4713349413375,4.42891000228215,150.910803360891));
#158836=CARTESIAN_POINT('Ctrl Pts',(18.4913432679761,4.40101867870896,150.873577155597));
#158837=CARTESIAN_POINT('Ctrl Pts',(18.5097976222555,4.37442217458881,150.835022880457));
#158838=CARTESIAN_POINT('Ctrl Pts',(18.5292444217898,4.34639535359538,150.794395218905));
#158839=CARTESIAN_POINT('Ctrl Pts',(18.5462486579485,4.31943573437702,150.752388020248));
#158840=CARTESIAN_POINT('Ctrl Pts',(18.5609892954202,4.29383785418226,150.709206820558));
#158841=CARTESIAN_POINT('Ctrl Pts',(18.5757609439036,4.26818612176019,150.66593477726));
#158842=CARTESIAN_POINT('Ctrl Pts',(18.5882600126999,4.24390184679293,150.621483899194));
#158843=CARTESIAN_POINT('Ctrl Pts',(18.5986661429026,4.22123002260434,150.576071609115));
#158844=CARTESIAN_POINT('Ctrl Pts',(18.6090913275091,4.19851668460743,150.530576165732));
#158845=CARTESIAN_POINT('Ctrl Pts',(18.617416379132,4.17742164365807,150.484115911147));
#158846=CARTESIAN_POINT('Ctrl Pts',(18.6238137156254,4.1581403294452,150.436918302939));
#158847=CARTESIAN_POINT('Ctrl Pts',(18.6287640278216,4.14322028811149,150.400396401084));
#158848=CARTESIAN_POINT('Ctrl Pts',(18.6325599423428,4.12938523005701,150.36343318447));
#158849=CARTESIAN_POINT('Ctrl Pts',(18.6352754623615,4.11670530563327,150.326136917576));
#158850=CARTESIAN_POINT('Ctrl Pts',(18.6387914804342,4.10028751341469,150.277846222779));
#158851=CARTESIAN_POINT('Ctrl Pts',(18.6404971161023,4.08580781121885,150.228997108719));
#158852=CARTESIAN_POINT('Ctrl Pts',(18.6405359001165,4.07337555758929,150.179829108576));
#158853=CARTESIAN_POINT('Ctrl Pts',(18.6405747401186,4.06092535698763,150.130590130415));
#158854=CARTESIAN_POINT('Ctrl Pts',(18.638942151287,4.05052839958962,150.081031497016));
#158855=CARTESIAN_POINT('Ctrl Pts',(18.6357590644381,4.04224765948019,150.031396813581));
#158856=CARTESIAN_POINT('Ctrl Pts',(18.6325620265088,4.03393062589957,149.981544587398));
#158857=CARTESIAN_POINT('Ctrl Pts',(18.6278010355476,4.02774830027686,149.931615802684));
#158858=CARTESIAN_POINT('Ctrl Pts',(18.6215721414155,4.02371889111107,149.881857991779));
#158859=CARTESIAN_POINT('Ctrl Pts',(18.6169055376704,4.02070011193378,149.844580108773));
#158860=CARTESIAN_POINT('Ctrl Pts',(18.6114144783443,4.01888877449659,149.807398219849));
#158861=CARTESIAN_POINT('Ctrl Pts',(18.6051290423695,4.0182763981666,149.770415847677));
#158862=CARTESIAN_POINT('',(17.7320851166166,2.73630903683038,149.924354425571));
#158863=CARTESIAN_POINT('Origin',(19.0783287073222,2.73849310306824,149.686975357862));
#158864=CARTESIAN_POINT('Origin',(16.2505544908171,2.73391286142859,150.159005790699));
#158865=CARTESIAN_POINT('Origin',(19.0824366510928,-2.76149987721566,149.659668559686));
#158866=CARTESIAN_POINT('',(17.8030144592149,-5.16515196693523,151.408405127377));
#158867=CARTESIAN_POINT('',(17.0246388076071,-4.39725480535896,151.545653753608));
#158868=CARTESIAN_POINT('Ctrl Pts',(17.8030144477807,-5.16515196697007,
151.408405062833));
#158869=CARTESIAN_POINT('Ctrl Pts',(17.6031647754424,-5.03312458159598,
151.443643952118));
#158870=CARTESIAN_POINT('Ctrl Pts',(17.3277548264866,-4.79507474988715,
151.492206235477));
#158871=CARTESIAN_POINT('Ctrl Pts',(17.0993533621461,-4.50629347348466,
151.532479576936));
#158872=CARTESIAN_POINT('Ctrl Pts',(17.0246388097555,-4.3972548053579,151.545653765783));
#158873=CARTESIAN_POINT('',(16.5196805691194,-2.76608011964102,151.634691519724));
#158874=CARTESIAN_POINT('Ctrl Pts',(17.0246388054587,-4.39725480536002,
151.545653741432));
#158875=CARTESIAN_POINT('Ctrl Pts',(16.980179831894,-4.33237122813037,151.553493065376));
#158876=CARTESIAN_POINT('Ctrl Pts',(16.9382853629388,-4.26557476157888,
151.560880198771));
#158877=CARTESIAN_POINT('Ctrl Pts',(16.8992102235566,-4.19709416983573,
151.567770201294));
#158878=CARTESIAN_POINT('Ctrl Pts',(16.8866244911932,-4.17503721972902,
151.56998940586));
#158879=CARTESIAN_POINT('Ctrl Pts',(16.8743310868166,-4.15280592507466,
151.572157064749));
#158880=CARTESIAN_POINT('Ctrl Pts',(16.8623380347648,-4.1304089735751,151.574271763407));
#158881=CARTESIAN_POINT('Ctrl Pts',(16.8248877436378,-4.06047078349699,
151.580875260168));
#158882=CARTESIAN_POINT('Ctrl Pts',(16.7903359033042,-3.98891417475552,
151.586967682095));
#158883=CARTESIAN_POINT('Ctrl Pts',(16.7588050789201,-3.9160820073487,151.592527416549));
#158884=CARTESIAN_POINT('Ctrl Pts',(16.727125626097,-3.84290652727713,151.598113358203));
#158885=CARTESIAN_POINT('Ctrl Pts',(16.6984958086485,-3.76844397059384,
151.603161565509));
#158886=CARTESIAN_POINT('Ctrl Pts',(16.672988491886,-3.69304977473514,151.607659193346));
#158887=CARTESIAN_POINT('Ctrl Pts',(16.6480921897446,-3.61946160796379,
151.612049082827));
#158888=CARTESIAN_POINT('Ctrl Pts',(16.6261703394414,-3.54498638983783,
151.615914500064));
#158889=CARTESIAN_POINT('Ctrl Pts',(16.6072434948582,-3.46995433517785,
151.619251813424));
#158890=CARTESIAN_POINT('Ctrl Pts',(16.5910626489886,-3.40580829612739,
151.622104933121));
#158891=CARTESIAN_POINT('Ctrl Pts',(16.5771441731587,-3.34124760024139,
151.624559132651));
#158892=CARTESIAN_POINT('Ctrl Pts',(16.5654479168803,-3.27621426711835,
151.626621497644));
#158893=CARTESIAN_POINT('Ctrl Pts',(16.5537840579261,-3.21136106906744,
151.628678150116));
#158894=CARTESIAN_POINT('Ctrl Pts',(16.5443299721102,-3.14603718468865,
151.630345161695));
#158895=CARTESIAN_POINT('Ctrl Pts',(16.5370953273655,-3.08017315174642,
151.631620825864));
#158896=CARTESIAN_POINT('Ctrl Pts',(16.5299478482173,-3.01510267231301,
151.632881120374));
#158897=CARTESIAN_POINT('Ctrl Pts',(16.5249666064023,-2.94950433109478,
151.633759448475));
#158898=CARTESIAN_POINT('Ctrl Pts',(16.5222106325192,-2.88330921082613,
151.634245401212));
#158899=CARTESIAN_POINT('Ctrl Pts',(16.5205924674715,-2.84444286648317,
151.634530727476));
#158900=CARTESIAN_POINT('Ctrl Pts',(16.5197423899986,-2.80537079682772,
151.634680619052));
#158901=CARTESIAN_POINT('Ctrl Pts',(16.5196805691229,-2.76608012003402,
151.634691519741));
#158902=CARTESIAN_POINT('',(17.7407389282419,-2.76368394459876,149.922828525116));
#158903=CARTESIAN_POINT('Origin',(16.2592083024477,-2.7660801188553,150.157479890222));
#158904=CARTESIAN_POINT('',(18.6178127187803,-4.0428120877243,149.768179371269));
#158905=CARTESIAN_POINT('Origin',(19.0869825189528,-2.76149987721565,149.685449457386));
#158906=CARTESIAN_POINT('Ctrl Pts',(18.617812536877,-4.04281201894015,149.768179403335));
#158907=CARTESIAN_POINT('Ctrl Pts',(18.6247401961886,-4.0434875741113,149.808927579398));
#158908=CARTESIAN_POINT('Ctrl Pts',(18.6307224387778,-4.04558831789134,
149.850751083093));
#158909=CARTESIAN_POINT('Ctrl Pts',(18.6356396503344,-4.0493168664848,149.893503877485));
#158910=CARTESIAN_POINT('Ctrl Pts',(18.6404443940295,-4.05296013465421,
149.935278817803));
#158911=CARTESIAN_POINT('Ctrl Pts',(18.6442323371476,-4.05815801892354,
149.977941025346));
#158912=CARTESIAN_POINT('Ctrl Pts',(18.646863348556,-4.06507915814563,150.021321280173));
#158913=CARTESIAN_POINT('Ctrl Pts',(18.6495033041142,-4.07202382585026,
150.064849006613));
#158914=CARTESIAN_POINT('Ctrl Pts',(18.6509785664528,-4.08070406885189,
150.109099781635));
#158915=CARTESIAN_POINT('Ctrl Pts',(18.6511169129511,-4.09126184905199,
150.153868015298));
#158916=CARTESIAN_POINT('Ctrl Pts',(18.6512552594495,-4.10181962925208,
150.19863624896));
#158917=CARTESIAN_POINT('Ctrl Pts',(18.6500566898563,-4.11425558887344,
150.243921988825));
#158918=CARTESIAN_POINT('Ctrl Pts',(18.6473174902442,-4.12867414193584,
150.289483893473));
#158919=CARTESIAN_POINT('Ctrl Pts',(18.6447913376859,-4.14197126148257,
150.331502124447));
#158920=CARTESIAN_POINT('Ctrl Pts',(18.6409544671681,-4.15695459366357,
150.373754845816));
#158921=CARTESIAN_POINT('Ctrl Pts',(18.6356240268674,-4.1736703057728,150.416025570632));
#158922=CARTESIAN_POINT('Ctrl Pts',(18.6303765276118,-4.19012592330175,
150.457638567775));
#158923=CARTESIAN_POINT('Ctrl Pts',(18.6236813521633,-4.20826079186167,
150.499268906268));
#158924=CARTESIAN_POINT('Ctrl Pts',(18.6153450232028,-4.2280795345367,150.54068568822));
#158925=CARTESIAN_POINT('Ctrl Pts',(18.6071814355015,-4.24748760309108,
150.581244252233));
#158926=CARTESIAN_POINT('Ctrl Pts',(18.5974436983681,-4.26851076455874,
150.621597865278));
#158927=CARTESIAN_POINT('Ctrl Pts',(18.5859356427768,-4.29111059082044,
150.661508081389));
#158928=CARTESIAN_POINT('Ctrl Pts',(18.582139493849,-4.29856556925292,150.674673218011));
#158929=CARTESIAN_POINT('Ctrl Pts',(18.5781506118915,-4.30619174058161,
150.687789939588));
#158930=CARTESIAN_POINT('Ctrl Pts',(18.5739616953087,-4.3139865953369,150.700849202694));
#158931=CARTESIAN_POINT('Ctrl Pts',(18.5667904471748,-4.32733105720735,
150.723206109146));
#158932=CARTESIAN_POINT('Ctrl Pts',(18.559032968913,-4.34117019340261,150.745394719647));
#158933=CARTESIAN_POINT('Ctrl Pts',(18.5506519942545,-4.355487266246,150.767368082748));
#158934=CARTESIAN_POINT('Ctrl Pts',(18.5464615069252,-4.3626458026677,150.778354764298));
#158935=CARTESIAN_POINT('Ctrl Pts',(18.5421151592065,-4.36992380104806,
150.789287654068));
#158936=CARTESIAN_POINT('Ctrl Pts',(18.5376082142567,-4.3773185881527,150.800160647524));
#158937=CARTESIAN_POINT('Ctrl Pts',(18.5353547417818,-4.38101598170501,
150.805597144252));
#158938=CARTESIAN_POINT('Ctrl Pts',(18.5330611210657,-4.38474257067892,
150.81101866842));
#158939=CARTESIAN_POINT('Ctrl Pts',(18.5307267628424,-4.38849799834734,
150.816424455196));
#158940=CARTESIAN_POINT('Ctrl Pts',(18.5295595837308,-4.39037571218156,
150.819127348584));
#158941=CARTESIAN_POINT('Ctrl Pts',(18.5283822203052,-4.39226063559047,
150.82182630772));
#158942=CARTESIAN_POINT('Ctrl Pts',(18.5271945987749,-4.39415272176831,
150.824521236267));
#158943=CARTESIAN_POINT('Ctrl Pts',(18.526221894561,-4.39570240754895,150.826728478461));
#158944=CARTESIAN_POINT('Ctrl Pts',(18.5248709135798,-4.39784386759893,
150.829763064945));
#158945=CARTESIAN_POINT('Ctrl Pts',(18.5240538436865,-4.39913510367867,
150.831585101082));
#158946=CARTESIAN_POINT('Ctrl Pts',(18.5238733135046,-4.39942040006074,
150.83198767682));
#158947=CARTESIAN_POINT('Ctrl Pts',(18.5237189903995,-4.39966407142166,
150.832331198531));
#158948=CARTESIAN_POINT('Ctrl Pts',(18.5236008861957,-4.39985042090695,
150.832593833795));
#158949=CARTESIAN_POINT('Ctrl Pts',(18.5169837837748,-4.41029114689819,
150.847308673622));
#158950=CARTESIAN_POINT('Ctrl Pts',(18.5094035732404,-4.42195192080497,
150.863333569431));
#158951=CARTESIAN_POINT('Ctrl Pts',(18.5007046991651,-4.43493162585227,
150.880507535861));
#158952=CARTESIAN_POINT('Ctrl Pts',(18.492178102557,-4.44765427341244,150.897341379258));
#158953=CARTESIAN_POINT('Ctrl Pts',(18.4825765824297,-4.46164474473058,
150.915279447519));
#158954=CARTESIAN_POINT('Ctrl Pts',(18.4717247631423,-4.47699417422253,
150.934129532891));
#158955=CARTESIAN_POINT('Ctrl Pts',(18.4612660869295,-4.49178751982269,
150.952296711524));
#158956=CARTESIAN_POINT('Ctrl Pts',(18.4496458069598,-4.50784372002333,
150.971311078383));
#158957=CARTESIAN_POINT('Ctrl Pts',(18.4366827522023,-4.52523385814105,
150.990960683196));
#158958=CARTESIAN_POINT('Ctrl Pts',(18.4240133975992,-4.54222999296668,
151.010165092638));
#158959=CARTESIAN_POINT('Ctrl Pts',(18.4100611626767,-4.56050088978042,
151.029976374868));
#158960=CARTESIAN_POINT('Ctrl Pts',(18.394637062584,-4.58009421356124,151.050156624144));
#158961=CARTESIAN_POINT('Ctrl Pts',(18.3797843883863,-4.59896165171437,
151.069589243611));
#158962=CARTESIAN_POINT('Ctrl Pts',(18.36356653662,-4.61905581378937,151.089363930518));
#158963=CARTESIAN_POINT('Ctrl Pts',(18.3458006418009,-4.64039421716833,
151.109230676935));
#158964=CARTESIAN_POINT('Ctrl Pts',(18.3300948332558,-4.65925827560971,
151.126793727872));
#158965=CARTESIAN_POINT('Ctrl Pts',(18.3131788106762,-4.67909469083498,
151.144428244391));
#158966=CARTESIAN_POINT('Ctrl Pts',(18.2949200820071,-4.69989366150591,
151.161936176571));
#158967=CARTESIAN_POINT('Ctrl Pts',(18.2857552887525,-4.71033350480281,
151.170724114749));
#158968=CARTESIAN_POINT('Ctrl Pts',(18.276252137315,-4.72101549961146,151.179479781068));
#158969=CARTESIAN_POINT('Ctrl Pts',(18.2663936047421,-4.73193600197506,
151.188175816906));
#158970=CARTESIAN_POINT('Ctrl Pts',(18.2611983184977,-4.73769092901845,
151.192758486287));
#158971=CARTESIAN_POINT('Ctrl Pts',(18.25562747465,-4.74381594765354,151.197562783229));
#158972=CARTESIAN_POINT('Ctrl Pts',(18.2501128722837,-4.74983064582462,
151.202203432408));
#158973=CARTESIAN_POINT('Ctrl Pts',(18.2451630104228,-4.75522938957876,
151.206368841055));
#158974=CARTESIAN_POINT('Ctrl Pts',(18.2402590238559,-4.76053903323933,
151.210403073422));
#158975=CARTESIAN_POINT('Ctrl Pts',(18.2357348032586,-4.76540758764143,
151.214056119989));
#158976=CARTESIAN_POINT('Ctrl Pts',(18.2104452633172,-4.79262188861566,
151.234475961391));
#158977=CARTESIAN_POINT('Ctrl Pts',(18.1849808019506,-4.81917655659402,
151.252858774329));
#158978=CARTESIAN_POINT('Ctrl Pts',(18.159568537672,-4.84492883335936,151.269416046978));
#158979=CARTESIAN_POINT('Ctrl Pts',(18.1334500898831,-4.87139674227017,
151.286433431044));
#158980=CARTESIAN_POINT('Ctrl Pts',(18.1073871349694,-4.89701735989194,
151.301522906798));
#158981=CARTESIAN_POINT('Ctrl Pts',(18.0816053781645,-4.92168676407901,
151.314920793821));
#158982=CARTESIAN_POINT('Ctrl Pts',(18.0546865634699,-4.94744416784942,
151.328909570489));
#158983=CARTESIAN_POINT('Ctrl Pts',(18.0280746598158,-4.97216491409709,
151.341054792255));
#158984=CARTESIAN_POINT('Ctrl Pts',(18.0019983724429,-4.99578093615701,
151.351624537475));
#158985=CARTESIAN_POINT('Ctrl Pts',(17.9753055934216,-5.01995528464432,
151.362444171016));
#158986=CARTESIAN_POINT('Ctrl Pts',(17.9491742270689,-5.04297261980922,
151.371613467534));
#158987=CARTESIAN_POINT('Ctrl Pts',(17.9238166183558,-5.06480438672461,
151.379410864763));
#158988=CARTESIAN_POINT('Ctrl Pts',(17.8975602901792,-5.08740991090049,
151.387484615837));
#158989=CARTESIAN_POINT('Ctrl Pts',(17.8721336705373,-5.10874491376694,
151.394088022405));
#158990=CARTESIAN_POINT('Ctrl Pts',(17.8477350782245,-5.12881605336842,
151.399512408282));
#158991=CARTESIAN_POINT('Ctrl Pts',(17.8324094016906,-5.14142349355419,
151.402919669745));
#158992=CARTESIAN_POINT('Ctrl Pts',(17.8174885798052,-5.15353299626255,
151.405861348784));
#158993=CARTESIAN_POINT('Ctrl Pts',(17.8030144302228,-5.16515196687232,
151.408404962689));
#158994=CARTESIAN_POINT('Origin',(-3.46221193726519,-0.0437048830555943,
137.895785892187));
#158995=CARTESIAN_POINT('',(16.1274832823092,-0.0125284566453824,136.624761290332));
#158996=CARTESIAN_POINT('',(15.4719024191847,-0.0123825748629563,132.374023471094));
#158997=CARTESIAN_POINT('Ctrl Pts',(16.1278796078287,-0.012527862009953,
136.624691413793));
#158998=CARTESIAN_POINT('Ctrl Pts',(16.1280756600303,-0.147252630708614,
136.624656901064));
#158999=CARTESIAN_POINT('Ctrl Pts',(16.1260140219066,-0.281703535965217,
136.612160674053));
#159000=CARTESIAN_POINT('Ctrl Pts',(16.1184237857483,-0.550546425183159,
136.561598615638));
#159001=CARTESIAN_POINT('Ctrl Pts',(16.1127815881379,-0.684158670131424,
136.522886157832));
#159002=CARTESIAN_POINT('Ctrl Pts',(16.0999699315943,-0.900695439409687,
136.436931228838));
#159003=CARTESIAN_POINT('Ctrl Pts',(16.0938142045473,-0.985927359311978,
136.396487701947));
#159004=CARTESIAN_POINT('Ctrl Pts',(16.0774730187525,-1.179187317559,136.288758970976));
#159005=CARTESIAN_POINT('Ctrl Pts',(16.0667146508231,-1.28439591328589,
136.217237967408));
#159006=CARTESIAN_POINT('Ctrl Pts',(16.0477442990125,-1.43633696818377,
136.093006015257));
#159007=CARTESIAN_POINT('Ctrl Pts',(16.0406072535459,-1.48790350507802,
136.046492779664));
#159008=CARTESIAN_POINT('Ctrl Pts',(16.0180809062315,-1.63604495799591,
135.899176828029));
#159009=CARTESIAN_POINT('Ctrl Pts',(16.0017341497931,-1.72501087141097,
135.791412214741));
#159010=CARTESIAN_POINT('Ctrl Pts',(15.9484822225129,-1.95897592507266,
135.443568696062));
#159011=CARTESIAN_POINT('Ctrl Pts',(15.9084293170325,-2.06745293008694,
135.183131963649));
#159012=CARTESIAN_POINT('Ctrl Pts',(15.8454622575998,-2.14896862539609,
134.773809102494));
#159013=CARTESIAN_POINT('Ctrl Pts',(15.8242126961341,-2.16253104213606,
134.635901479587));
#159014=CARTESIAN_POINT('Ctrl Pts',(15.7600738513876,-2.16229456842722,
134.220112412375));
#159015=CARTESIAN_POINT('Ctrl Pts',(15.7176216288766,-2.10713461966444,
133.945253864148));
#159016=CARTESIAN_POINT('Ctrl Pts',(15.658003533512,-1.94659995619521,133.560448072899));
#159017=CARTESIAN_POINT('Ctrl Pts',(15.6389302244503,-1.88053411433489,
133.437714497772));
#159018=CARTESIAN_POINT('Ctrl Pts',(15.5849918526666,-1.64667906149591,
133.090062319416));
#159019=CARTESIAN_POINT('Ctrl Pts',(15.5541314319578,-1.44578832059754,
132.890481229408));
#159020=CARTESIAN_POINT('Ctrl Pts',(15.5104027469076,-1.03166236295503,
132.615596514834));
#159021=CARTESIAN_POINT('Ctrl Pts',(15.4963699054271,-0.834355542246234,
132.523574025011));
#159022=CARTESIAN_POINT('Ctrl Pts',(15.4775279834229,-0.427200653112934,
132.403665195811));
#159023=CARTESIAN_POINT('Ctrl Pts',(15.4719964486658,-0.220326112747798,
132.374007009116));
#159024=CARTESIAN_POINT('Ctrl Pts',(15.4715027782058,-0.0123835530891811,
132.374093927259));
#159025=CARTESIAN_POINT('',(18.4340776165402,-0.00878730969903237,136.218046482001));
#159026=CARTESIAN_POINT('',(-3.08886835528135,-0.0437048830555946,140.013122561163));
#159027=CARTESIAN_POINT('Origin',(18.0607340345509,-0.0087873096990321,
134.100709812994));
#159028=CARTESIAN_POINT('Ctrl Pts',(15.4723019669606,-0.0123818775344335,
132.373953008719));
#159029=CARTESIAN_POINT('Ctrl Pts',(15.4720739225224,0.122337644049303,
132.373993159465));
#159030=CARTESIAN_POINT('Ctrl Pts',(15.4734478511091,0.25678132131525,132.386609333691));
#159031=CARTESIAN_POINT('Ctrl Pts',(15.4805945056066,0.525616774422636,
132.437246534484));
#159032=CARTESIAN_POINT('Ctrl Pts',(15.4864564770072,0.659236057971183,
132.475920825168));
#159033=CARTESIAN_POINT('Ctrl Pts',(15.4994543432378,0.875785798846138,
132.561846679565));
#159034=CARTESIAN_POINT('Ctrl Pts',(15.5055005624332,0.961013695629594,
132.602308731372));
#159035=CARTESIAN_POINT('Ctrl Pts',(15.5217640239017,1.15425338252864,132.710038136568));
#159036=CARTESIAN_POINT('Ctrl Pts',(15.5327218200456,1.25946737867874,132.781523829943));
#159037=CARTESIAN_POINT('Ctrl Pts',(15.5515854786746,1.41143029625106,132.905791858573));
#159038=CARTESIAN_POINT('Ctrl Pts',(15.5586329892119,1.46300914551536,132.952333036519));
#159039=CARTESIAN_POINT('Ctrl Pts',(15.5810696143101,1.61114009658696,133.09965967983));
#159040=CARTESIAN_POINT('Ctrl Pts',(15.5976677826201,1.70009826756318,133.207367676168));
#159041=CARTESIAN_POINT('Ctrl Pts',(15.6509515974162,1.9340590641442,133.555197445029));
#159042=CARTESIAN_POINT('Ctrl Pts',(15.6908841576945,2.04253968408142,133.815655476476));
#159043=CARTESIAN_POINT('Ctrl Pts',(15.7539112731536,2.12405772760858,134.224977826637));
#159044=CARTESIAN_POINT('Ctrl Pts',(15.7751563397812,2.13762000308831,134.362886607084));
#159045=CARTESIAN_POINT('Ctrl Pts',(15.8392705263805,2.13738358102934,134.778675904911));
#159046=CARTESIAN_POINT('Ctrl Pts',(15.8817767412965,2.08222503727033,135.05352591926));
#159047=CARTESIAN_POINT('Ctrl Pts',(15.9413746662881,1.92168664483466,135.438343380605));
#159048=CARTESIAN_POINT('Ctrl Pts',(15.960375686495,1.85561760089108,135.561095264048));
#159049=CARTESIAN_POINT('Ctrl Pts',(16.0144310397426,1.62173151582931,135.90876638651));
#159050=CARTESIAN_POINT('Ctrl Pts',(16.0457627258355,1.42084183019191,136.108235901066));
#159051=CARTESIAN_POINT('Ctrl Pts',(16.0882048047342,1.00669224073221,136.383367061237));
#159052=CARTESIAN_POINT('Ctrl Pts',(16.1031585177866,0.809464228630117,
136.475177773857));
#159053=CARTESIAN_POINT('Ctrl Pts',(16.1226011363339,0.402306803369797,
136.594985487103));
#159054=CARTESIAN_POINT('Ctrl Pts',(16.1269248006866,0.195420549416648,
136.624859648122));
#159055=CARTESIAN_POINT('Ctrl Pts',(16.1270868790944,-0.0125287751724091,
136.624831193257));
#159056=CARTESIAN_POINT('Origin',(34.7113261754309,-17.2069969078973,150.45786679959));
#159057=CARTESIAN_POINT('',(34.7286909932009,-17.2069969078973,150.55634757489));
#159058=CARTESIAN_POINT('',(34.1022561745275,-15.848549783591,150.666804935116));
#159059=CARTESIAN_POINT('',(34.7286909932009,-17.2069969078973,150.55634757489));
#159060=CARTESIAN_POINT('',(34.0848913567676,-15.848549783591,150.568324159816));
#159061=CARTESIAN_POINT('',(34.0848913567676,-15.848549783591,150.568324159816));
#159062=CARTESIAN_POINT('',(34.7113261754309,-17.2069969078973,150.45786679959));
#159063=CARTESIAN_POINT('',(34.7113261754309,-17.2069969078973,150.45786679959));
#159064=CARTESIAN_POINT('',(34.7113261754309,-17.2069969078973,150.45786679959));
#159065=CARTESIAN_POINT('Origin',(26.7764851389615,-2.04263841746052E-14,
151.856993361954));
#159066=CARTESIAN_POINT('',(43.7647022487539,-8.00222469971588,148.963054992579));
#159067=CARTESIAN_POINT('Origin',(26.7938499567315,-1.48611011759408E-14,
151.955474137254));
#159068=CARTESIAN_POINT('',(43.7473374309938,-8.00222469971587,148.864574217279));
#159069=CARTESIAN_POINT('Origin',(26.7764851389615,-2.04263841746052E-14,
151.856993361954));
#159070=CARTESIAN_POINT('',(43.7473374309938,-8.00222469971587,148.864574217279));
#159071=CARTESIAN_POINT('Origin',(26.7938499567315,-1.48611011759408E-14,
151.955474137254));
#159072=CARTESIAN_POINT('',(42.4248981204347,-7.37047011815913,149.199298609248));
#159073=CARTESIAN_POINT('Origin',(26.7938499567315,-1.48611011759408E-14,
151.955474137254));
#159074=CARTESIAN_POINT('',(42.4248981204347,-7.37047011815913,149.199298609248));
#159075=CARTESIAN_POINT('Origin',(26.7764851389615,-2.04263841746052E-14,
151.856993361954));
#159076=CARTESIAN_POINT('',(42.4075333026747,-7.37047011815912,149.100817833948));
#159077=CARTESIAN_POINT('Origin',(26.7764851389615,-2.04263841746052E-14,
151.856993361954));
#159078=CARTESIAN_POINT('',(42.4075333026747,-7.37047011815912,149.100817833948));
#159079=CARTESIAN_POINT('Origin',(42.4075333026747,-7.37047011815912,149.100817833948));
#159080=CARTESIAN_POINT('',(42.4075333026747,-7.37047011815912,149.100817833948));
#159081=CARTESIAN_POINT('Origin',(26.7938499567315,-1.48611011759408E-14,
151.955474137254));
#159082=CARTESIAN_POINT('',(43.7394339176877,8.05724874950928,148.967510481072));
#159083=CARTESIAN_POINT('',(34.6745028823554,17.232655043704,150.565902400871));
#159084=CARTESIAN_POINT('Origin',(26.7938499567315,-1.48611011759408E-14,
151.955474137254));
#159085=CARTESIAN_POINT('',(34.052346072443,15.8721822770942,150.675605432751));
#159086=CARTESIAN_POINT('',(34.6745028823554,17.232655043704,150.565902400871));
#159087=CARTESIAN_POINT('',(42.4016246576106,7.42115016402197,149.20340234871));
#159088=CARTESIAN_POINT('Origin',(26.7938499567315,-1.48611011759408E-14,
151.955474137254));
#159089=CARTESIAN_POINT('',(42.4016246576106,7.42115016402197,149.20340234871));
#159090=CARTESIAN_POINT('Origin',(26.7764851389615,-2.04263841746052E-14,
151.856993361954));
#159091=CARTESIAN_POINT('',(34.6571380645954,17.232655043704,150.467421625571));
#159092=CARTESIAN_POINT('',(34.6571380645954,17.232655043704,150.467421625571));
#159093=CARTESIAN_POINT('',(43.7220690999277,8.05724874950929,148.869029705772));
#159094=CARTESIAN_POINT('',(43.7220690999277,8.05724874950929,148.869029705772));
#159095=CARTESIAN_POINT('Origin',(26.7764851389615,-2.04263841746052E-14,
151.856993361954));
#159096=CARTESIAN_POINT('Origin',(34.6571380645954,17.232655043704,150.467421625571));
#159097=CARTESIAN_POINT('',(34.034981254673,15.8721822770942,150.577124657451));
#159098=CARTESIAN_POINT('',(34.034981254673,15.8721822770942,150.577124657451));
#159099=CARTESIAN_POINT('',(34.6571380645954,17.232655043704,150.467421625571));
#159100=CARTESIAN_POINT('Origin',(26.7764851389615,-2.04263841746052E-14,
151.856993361954));
#159101=CARTESIAN_POINT('',(42.3842598398506,7.42115016402198,149.10492157341));
#159102=CARTESIAN_POINT('',(42.3842598398506,7.42115016402198,149.10492157341));
#159103=CARTESIAN_POINT('Origin',(26.7764851389615,-2.04263841746052E-14,
151.856993361954));
#159104=CARTESIAN_POINT('Origin',(42.3842598398506,7.42115016402198,149.10492157341));
#159105=CARTESIAN_POINT('',(42.3842598398506,7.42115016402198,149.10492157341));
#159106=CARTESIAN_POINT('Origin',(16.7219736911164,-6.50941809057164,128.751923016915));
#159107=CARTESIAN_POINT('',(16.7219736911164,-6.50941809057164,128.751923016915));
#159108=CARTESIAN_POINT('',(20.3737087297297,-6.87643093232191,149.458564755529));
#159109=CARTESIAN_POINT('',(16.7219736911164,-6.50941809057164,128.751923016915));
#159110=CARTESIAN_POINT('',(27.5548451481147,-6.49184346932355,126.841795500437));
#159111=CARTESIAN_POINT('',(16.7219736911164,-6.50941809057164,128.751923016915));
#159112=CARTESIAN_POINT('',(31.2065801874991,-6.8588563110934,147.548437240149));
#159113=CARTESIAN_POINT('',(27.5548451481147,-6.49184346932355,126.841795500437));
#159114=CARTESIAN_POINT('',(31.2065802141502,-6.85885631372248,147.548437388466));
#159115=CARTESIAN_POINT('Origin',(29.3788505316782,-5.49184474563557,137.195444817487));
#159116=CARTESIAN_POINT('',(28.5380782239063,-5.49024705279486,126.668424980917));
#159117=CARTESIAN_POINT('Origin',(27.5532717278182,-5.49184474563557,126.842072936887));
#159118=CARTESIAN_POINT('',(32.5506728884128,-5.48966067834193,147.311437431176));
#159119=CARTESIAN_POINT('',(28.5380782239063,-5.49024705279486,126.668424980917));
#159120=CARTESIAN_POINT('Origin',(31.2044292741582,-5.49184474563556,147.548816349987));
#159121=CARTESIAN_POINT('Origin',(28.5380782239063,-5.49024705279486,126.668424980917));
#159122=CARTESIAN_POINT('',(28.5207706006449,5.50973890777291,126.671476781869));
#159123=CARTESIAN_POINT('',(28.5380782239063,-5.49024705279486,126.668424980917));
#159124=CARTESIAN_POINT('',(32.5333652653764,5.51032528280824,147.314489233291));
#159125=CARTESIAN_POINT('',(28.5207706006449,5.50973890777291,126.671476781869));
#159126=CARTESIAN_POINT('',(32.5333652941263,5.51032528330627,147.314489381211));
#159127=CARTESIAN_POINT('Origin',(29.3615429084169,5.5081412149322,137.19849661844));
#159128=CARTESIAN_POINT('',(27.5343906842604,6.50813993862018,126.84540217429));
#159129=CARTESIAN_POINT('Origin',(27.5359641045569,5.5081412149322,126.84512473784));
#159130=CARTESIAN_POINT('',(31.1849707906507,6.87515278037055,147.552247558648));
#159131=CARTESIAN_POINT('',(27.5343906842604,6.50813993862018,126.84540217429));
#159132=CARTESIAN_POINT('Origin',(31.1871216508969,5.5081412149322,147.55186815094));
#159133=CARTESIAN_POINT('Origin',(27.5343906842604,6.50813993862018,126.84540217429));
#159134=CARTESIAN_POINT('',(16.7015192294221,6.4905653173756,128.755529690369));
#159135=CARTESIAN_POINT('',(27.5343906842604,6.50813993862018,126.84540217429));
#159136=CARTESIAN_POINT('',(20.3520993354489,6.85757815914594,149.46237507597));
#159137=CARTESIAN_POINT('',(16.7015192294221,6.4905653173756,128.755529690369));
#159138=CARTESIAN_POINT('',(20.3520993611167,6.85757816177451,149.462375224439));
#159139=CARTESIAN_POINT('Origin',(20.0759123749787,8.35691092392083,149.484491984831));
#159140=CARTESIAN_POINT('',(31.4385374584628,8.37491358353456,149.00409452878));
#159141=CARTESIAN_POINT('Origin',(31.1780651780795,8.3749224115792,147.526882901754));
#159142=CARTESIAN_POINT('',(20.6056660035708,8.3573389629198,150.914222044819));
#159143=CARTESIAN_POINT('Origin',(20.3451937232412,8.35734779033466,149.437010417732));
#159144=CARTESIAN_POINT('',(20.6056659874021,8.35734778978584,150.914222047732));
#159145=CARTESIAN_POINT('Origin',(31.1825758355569,5.50814121493218,147.52608755114));
#159146=CARTESIAN_POINT('',(34.2662677573925,5.51272144253028,148.505489382891));
#159147=CARTESIAN_POINT('Origin',(34.005804184202,5.51272145657184,147.028276220504));
#159148=CARTESIAN_POINT('Origin',(31.4430481020469,5.50814121493219,149.00329918054));
#159149=CARTESIAN_POINT('Origin',(34.0053739547706,5.78615690368945,147.02835208156));
#159150=CARTESIAN_POINT('',(34.2835753800336,-5.48726451810046,148.502437582047));
#159151=CARTESIAN_POINT('Origin',(34.0231118074634,-5.48726450399593,147.025224419551));
#159152=CARTESIAN_POINT('',(34.2662764501683,5.51272145895295,148.505487850204));
#159153=CARTESIAN_POINT('Origin',(31.1998834588183,-5.49184474563559,147.523035750187));
#159154=CARTESIAN_POINT('',(31.4648663689593,-8.35861711486726,148.999452031481));
#159155=CARTESIAN_POINT('Origin',(31.2043941162956,-8.35862594228162,147.522240399573));
#159156=CARTESIAN_POINT('Origin',(31.4603557253082,-5.49184474563557,149.000247379587));
#159157=CARTESIAN_POINT('Origin',(31.4736754645682,-8.35818907586777,147.474758832475));
#159158=CARTESIAN_POINT('',(20.6319949119108,-8.3761917354855,150.909579547881));
#159159=CARTESIAN_POINT('Origin',(20.3715226593074,-8.37620056352966,149.432367915951));
#159160=CARTESIAN_POINT('',(31.4648663851448,-8.35862594173281,148.999452028673));
#159161=CARTESIAN_POINT('Origin',(20.36701200183,-5.50941936688363,149.433163266565));
#159162=CARTESIAN_POINT('',(17.8042733066227,-5.51399958031571,151.408183160806));
#159163=CARTESIAN_POINT('',(19.0253142554132,-5.51160343525972,149.696323083178));
#159164=CARTESIAN_POINT('Origin',(17.5437836531848,-5.51399960852327,149.930974597102));
#159165=CARTESIAN_POINT('Origin',(20.37155781716,-5.50941936688365,149.458943866465));
#159166=CARTESIAN_POINT('Origin',(20.62748426831,-5.50941936688363,150.910374895965));
#159167=CARTESIAN_POINT('Origin',(18.54597907469,-5.50941936688364,139.105572333965));
#159168=CARTESIAN_POINT('',(15.7355937747319,-5.51101705972437,128.925848409336));
#159169=CARTESIAN_POINT('',(15.7355937747319,-5.51101705972437,128.925848409336));
#159170=CARTESIAN_POINT('Origin',(16.72040027082,-5.50941936688366,128.752200453365));
#159171=CARTESIAN_POINT('Origin',(15.7342146708969,-4.63451757771262,128.926091582552));
#159172=CARTESIAN_POINT('',(19.0239390506279,-4.63510509600238,149.696590864325));
#159173=CARTESIAN_POINT('',(19.0253142789822,-5.51160343624773,149.696323231995));
#159174=CARTESIAN_POINT('',(15.7342146642767,-4.63451676584635,128.926091509742));
#159175=CARTESIAN_POINT('',(19.023940582593,-4.63510509608687,149.696600544993));
#159176=CARTESIAN_POINT('',(15.7342146544329,-4.6345167235289,128.926091486888));
#159177=CARTESIAN_POINT('Origin',(17.5670013172358,-20.2701550170947,149.926880696501));
#159178=CARTESIAN_POINT('Ctrl Pts',(17.8042733066227,-5.51399958031571,
151.408183160806));
#159179=CARTESIAN_POINT('Ctrl Pts',(17.8040727766663,-5.39760138028505,
151.408218519755));
#159180=CARTESIAN_POINT('Ctrl Pts',(17.803197591333,-5.28155019758945,151.40837276968));
#159181=CARTESIAN_POINT('Ctrl Pts',(17.8030144477807,-5.16515196697007,
151.408405062833));
#159182=CARTESIAN_POINT('Ctrl Pts',(17.8030145110624,-5.16515196693421,
151.408405421157));
#159183=CARTESIAN_POINT('Ctrl Pts',(17.8032686440368,-5.16506456763226,
151.408360570365));
#159184=CARTESIAN_POINT('Ctrl Pts',(17.8035227301876,-5.16497718304309,
151.40831566124));
#159185=CARTESIAN_POINT('Ctrl Pts',(17.8037767695064,-5.16488981316054,
151.408270693831));
#159186=CARTESIAN_POINT('Ctrl Pts',(17.862944075151,-5.14454083502309,151.397797510206));
#159187=CARTESIAN_POINT('Ctrl Pts',(17.9195683479851,-5.12498821356407,
151.384163610296));
#159188=CARTESIAN_POINT('Ctrl Pts',(17.9735593295081,-5.10616350562641,
151.367997328169));
#159189=CARTESIAN_POINT('Ctrl Pts',(18.0141603152175,-5.09200740628533,
151.355840353596));
#159190=CARTESIAN_POINT('Ctrl Pts',(18.0532723727275,-5.07826346323026,
151.342251170234));
#159191=CARTESIAN_POINT('Ctrl Pts',(18.0908765654888,-5.06490598702596,
151.327492702657));
#159192=CARTESIAN_POINT('Ctrl Pts',(18.1306829185968,-5.05076627612203,
151.311869956134));
#159193=CARTESIAN_POINT('Ctrl Pts',(18.1687985096706,-5.03706161899898,
151.294938929714));
#159194=CARTESIAN_POINT('Ctrl Pts',(18.2051782310708,-5.02382494627252,
151.277032580921));
#159195=CARTESIAN_POINT('Ctrl Pts',(18.2421925228161,-5.01035738667676,
151.258813892245));
#159196=CARTESIAN_POINT('Ctrl Pts',(18.2774097802937,-4.99737420617687,
151.23958542498));
#159197=CARTESIAN_POINT('Ctrl Pts',(18.3108227210156,-4.98488683732149,
151.219669746269));
#159198=CARTESIAN_POINT('Ctrl Pts',(18.3257831989105,-4.97929568007251,
151.210752600257));
#159199=CARTESIAN_POINT('Ctrl Pts',(18.3403824934267,-4.97380362102034,
151.201697325601));
#159200=CARTESIAN_POINT('Ctrl Pts',(18.3546224893735,-4.96841030642996,
151.192531168065));
#159201=CARTESIAN_POINT('Ctrl Pts',(18.3847289059392,-4.95700767848437,
151.173151938035));
#159202=CARTESIAN_POINT('Ctrl Pts',(18.4132283127862,-4.94604727726768,
151.153278696366));
#159203=CARTESIAN_POINT('Ctrl Pts',(18.4401695613823,-4.93552410333679,
151.133157868164));
#159204=CARTESIAN_POINT('Ctrl Pts',(18.4715173128486,-4.923279762105,151.109746083091));
#159205=CARTESIAN_POINT('Ctrl Pts',(18.5007912709236,-4.91161856435262,
151.085973610496));
#159206=CARTESIAN_POINT('Ctrl Pts',(18.5281149683316,-4.90054938866558,
151.062158444953));
#159207=CARTESIAN_POINT('Ctrl Pts',(18.5480297397248,-4.89248166269037,
151.044800853468));
#159208=CARTESIAN_POINT('Ctrl Pts',(18.5669090859487,-4.88472795998422,
151.027419554606));
#159209=CARTESIAN_POINT('Ctrl Pts',(18.5848077147215,-4.87728530986754,
151.01012314597));
#159210=CARTESIAN_POINT('Ctrl Pts',(18.6041734638248,-4.86923259830776,
150.991408979969));
#159211=CARTESIAN_POINT('Ctrl Pts',(18.6223913498396,-4.86154427010307,
150.972794478652));
#159212=CARTESIAN_POINT('Ctrl Pts',(18.6395346836216,-4.85422093190089,
150.95440742827));
#159213=CARTESIAN_POINT('Ctrl Pts',(18.6625785148652,-4.8443770023702,150.92969181044));
#159214=CARTESIAN_POINT('Ctrl Pts',(18.6836843450984,-4.83519218394656,
150.90538522494));
#159215=CARTESIAN_POINT('Ctrl Pts',(18.703043268029,-4.82666826822253,150.881742670367));
#159216=CARTESIAN_POINT('Ctrl Pts',(18.7066722600945,-4.8250703889066,150.877310675712));
#159217=CARTESIAN_POINT('Ctrl Pts',(18.7102398675248,-4.82349567172762,
150.872901881842));
#159218=CARTESIAN_POINT('Ctrl Pts',(18.7137473492472,-4.8219440464152,150.86851778913));
#159219=CARTESIAN_POINT('Ctrl Pts',(18.7248564520267,-4.81702964730051,
150.854632232375));
#159220=CARTESIAN_POINT('Ctrl Pts',(18.7353624974549,-4.81234775577349,
150.840994780032));
#159221=CARTESIAN_POINT('Ctrl Pts',(18.7453055442633,-4.8078983210624,150.827649249466));
#159222=CARTESIAN_POINT('Ctrl Pts',(18.7502770676675,-4.80567360370686,
150.820976484183));
#159223=CARTESIAN_POINT('Ctrl Pts',(18.7551077977608,-4.80350700062168,
150.814376668407));
#159224=CARTESIAN_POINT('Ctrl Pts',(18.7598027413949,-4.80139850535284,
150.807854732614));
#159225=CARTESIAN_POINT('Ctrl Pts',(18.7621502132119,-4.80034425771842,
150.804593764717));
#159226=CARTESIAN_POINT('Ctrl Pts',(18.7644637355996,-4.79930453704117,
150.801352264728));
#159227=CARTESIAN_POINT('Ctrl Pts',(18.7667439227061,-4.79827934252448,
150.798130829766));
#159228=CARTESIAN_POINT('Ctrl Pts',(18.7678840162594,-4.79776674526614,
150.796520112284));
#159229=CARTESIAN_POINT('Ctrl Pts',(18.7690157758177,-4.79725777954814,
150.79491441094));
#159230=CARTESIAN_POINT('Ctrl Pts',(18.7701392779379,-4.79675244527051,
150.793313798456));
#159231=CARTESIAN_POINT('Ctrl Pts',(18.7711622488311,-4.7962923284198,150.791856409145));
#159232=CARTESIAN_POINT('Ctrl Pts',(18.7715594121143,-4.79611369840959,
150.791290836496));
#159233=CARTESIAN_POINT('Ctrl Pts',(18.7730216399206,-4.79545584278048,
150.789192685758));
#159234=CARTESIAN_POINT('Ctrl Pts',(18.7731653385895,-4.7953911928143,150.788986492532));
#159235=CARTESIAN_POINT('Ctrl Pts',(18.7733192946451,-4.79532192767035,
150.788765471694));
#159236=CARTESIAN_POINT('Ctrl Pts',(18.7734850880704,-4.79524733665902,
150.788527299497));
#159237=CARTESIAN_POINT('Ctrl Pts',(18.7735686544069,-4.79520973988732,
150.788407251444));
#159238=CARTESIAN_POINT('Ctrl Pts',(18.7736522009151,-4.79517214962227,
150.788287194308));
#159239=CARTESIAN_POINT('Ctrl Pts',(18.7737357275941,-4.79513456586254,
150.788167128097));
#159240=CARTESIAN_POINT('Ctrl Pts',(18.7994173117021,-4.78357885099189,
150.751250893089));
#159241=CARTESIAN_POINT('Ctrl Pts',(18.8232225180652,-4.77263971823976,
150.713480061588));
#159242=CARTESIAN_POINT('Ctrl Pts',(18.8451390713033,-4.76233225449921,
150.675080910954));
#159243=CARTESIAN_POINT('Ctrl Pts',(18.8660880089645,-4.75247986516592,
150.638377082384));
#159244=CARTESIAN_POINT('Ctrl Pts',(18.8853114789135,-4.74320466491597,
150.601099478334));
#159245=CARTESIAN_POINT('Ctrl Pts',(18.902818577608,-4.7345010424511,150.563405237081));
#159246=CARTESIAN_POINT('Ctrl Pts',(18.9072890851304,-4.73227853771856,
150.553779862139));
#159247=CARTESIAN_POINT('Ctrl Pts',(18.9116477734959,-4.73009320328575,
150.544127096179));
#159248=CARTESIAN_POINT('Ctrl Pts',(18.9158949898502,-4.72794474002493,
150.534449081862));
#159249=CARTESIAN_POINT('Ctrl Pts',(18.9321731474239,-4.71971040002829,
150.497356494878));
#159250=CARTESIAN_POINT('Ctrl Pts',(18.9468132378253,-4.71201873441901,
150.459896796704));
#159251=CARTESIAN_POINT('Ctrl Pts',(18.9598456409741,-4.70487992765189,
150.422248501799));
#159252=CARTESIAN_POINT('Ctrl Pts',(18.9726834715103,-4.69784770263092,
150.385162292567));
#159253=CARTESIAN_POINT('Ctrl Pts',(18.9839615301877,-4.69135194893011,
150.347893225263));
#159254=CARTESIAN_POINT('Ctrl Pts',(18.9937149473093,-4.68538848733506,
150.310563172745));
#159255=CARTESIAN_POINT('Ctrl Pts',(18.9980741755566,-4.68272315579916,
150.293878741291));
#159256=CARTESIAN_POINT('Ctrl Pts',(19.0021289006343,-4.68016396806322,
150.277181459132));
#159257=CARTESIAN_POINT('Ctrl Pts',(19.0058824151226,-4.67770968246238,
150.260478952394));
#159258=CARTESIAN_POINT('Ctrl Pts',(19.0071873230318,-4.67685645099038,
150.254672332169));
#159259=CARTESIAN_POINT('Ctrl Pts',(19.0084558267926,-4.67601589330426,
150.24886506311));
#159260=CARTESIAN_POINT('Ctrl Pts',(19.0096881718686,-4.67518789459185,
150.243057804819));
#159261=CARTESIAN_POINT('Ctrl Pts',(19.0177907306694,-4.66974387701547,
150.204875600259));
#159262=CARTESIAN_POINT('Ctrl Pts',(19.0243258691249,-4.66479586263019,
150.166725395175));
#159263=CARTESIAN_POINT('Ctrl Pts',(19.0293672876622,-4.66039573729584,
150.128732829071));
#159264=CARTESIAN_POINT('Ctrl Pts',(19.0346499413677,-4.65578506309171,
150.088922293875));
#159265=CARTESIAN_POINT('Ctrl Pts',(19.0382926601038,-4.6517758526121,150.049284581529));
#159266=CARTESIAN_POINT('Ctrl Pts',(19.0403583521838,-4.64842129637797,
150.009911502095));
#159267=CARTESIAN_POINT('Ctrl Pts',(19.0409159290519,-4.64751582601433,
149.999283820201));
#159268=CARTESIAN_POINT('Ctrl Pts',(19.0413584816065,-4.64665802362371,
149.988675149452));
#159269=CARTESIAN_POINT('Ctrl Pts',(19.0416869720438,-4.64584887936723,
149.978086731175));
#159270=CARTESIAN_POINT('Ctrl Pts',(19.0428991363296,-4.64286305190253,
149.939014353356));
#159271=CARTESIAN_POINT('Ctrl Pts',(19.0425602936179,-4.64053893606678,
149.900221237493));
#159272=CARTESIAN_POINT('Ctrl Pts',(19.0407796597806,-4.63882574119599,
149.861866673758));
#159273=CARTESIAN_POINT('Ctrl Pts',(19.0389238726557,-4.63704023936122,
149.821893320412));
#159274=CARTESIAN_POINT('Ctrl Pts',(19.0355022508431,-4.63591816343537,
149.782395926731));
#159275=CARTESIAN_POINT('Ctrl Pts',(19.0306062369459,-4.63541455822507,
149.743509320325));
#159276=CARTESIAN_POINT('Ctrl Pts',(19.0286247156489,-4.63521073845036,
149.727771080937));
#159277=CARTESIAN_POINT('Ctrl Pts',(19.0264013147576,-4.63510837488812,
149.712132419708));
#159278=CARTESIAN_POINT('Ctrl Pts',(19.0239405861026,-4.6351050960812,149.696600544437));
#159279=CARTESIAN_POINT('Ctrl Pts',(17.6621982343867,-5.08983843849182,
151.41501950764));
#159280=CARTESIAN_POINT('Ctrl Pts',(17.6847306497354,-5.07160503979059,
151.411230178286));
#159281=CARTESIAN_POINT('Ctrl Pts',(17.7859585568119,-4.98827094266869,
151.390595823914));
#159282=CARTESIAN_POINT('Ctrl Pts',(17.9528371002266,-4.8392053876882,151.327196400169));
#159283=CARTESIAN_POINT('Ctrl Pts',(18.1412192519315,-4.64592260348376,
151.191964020737));
#159284=CARTESIAN_POINT('Ctrl Pts',(18.290663302471,-4.46611281318578,151.013567428543));
#159285=CARTESIAN_POINT('Ctrl Pts',(18.3989836624423,-4.30756139525972,
150.800619385748));
#159286=CARTESIAN_POINT('Ctrl Pts',(18.4664123754855,-4.17761345587552,
150.562907468878));
#159287=CARTESIAN_POINT('Ctrl Pts',(18.4959930732887,-4.08166751220023,
150.310538928411));
#159288=CARTESIAN_POINT('Ctrl Pts',(18.4927145236842,-4.02235496188064,
150.052984722078));
#159289=CARTESIAN_POINT('Ctrl Pts',(18.4685252055117,-4.00488505051922,
149.854449636007));
#159290=CARTESIAN_POINT('Ctrl Pts',(18.4477123504894,-4.00541093234517,
149.744136010205));
#159291=CARTESIAN_POINT('Ctrl Pts',(18.4423888805384,-4.0061290882458,149.718123679723));
#159292=CARTESIAN_POINT('Ctrl Pts',(17.8515417284861,-5.40956555909364,
151.471675872937));
#159293=CARTESIAN_POINT('Ctrl Pts',(17.8765946229952,-5.39089090765192,
151.470972088971));
#159294=CARTESIAN_POINT('Ctrl Pts',(17.9897535980413,-5.3046331251463,151.464325699469));
#159295=CARTESIAN_POINT('Ctrl Pts',(18.1813513235114,-5.14333102257086,
151.424477159));
#159296=CARTESIAN_POINT('Ctrl Pts',(18.4073681596413,-4.92052595862295,
151.31364703635));
#159297=CARTESIAN_POINT('Ctrl Pts',(18.5972951085453,-4.69933599657195,
151.14777762627));
#159298=CARTESIAN_POINT('Ctrl Pts',(18.7454331128204,-4.49100697775858,
150.931283323269));
#159299=CARTESIAN_POINT('Ctrl Pts',(18.8481060957408,-4.30814243871773,
150.670238207001));
#159300=CARTESIAN_POINT('Ctrl Pts',(18.9039096879475,-4.16387944968833,
150.37340949851));
#159301=CARTESIAN_POINT('Ctrl Pts',(18.9136043748492,-4.06987311790436,
150.052640225632));
#159302=CARTESIAN_POINT('Ctrl Pts',(18.8872116191077,-4.04226503063461,
149.797795335174));
#159303=CARTESIAN_POINT('Ctrl Pts',(18.8606390219642,-4.04409959522934,
149.65595859604));
#159304=CARTESIAN_POINT('Ctrl Pts',(18.8537000884272,-4.04552153588302,
149.622549665771));
#159305=CARTESIAN_POINT('Ctrl Pts',(17.9453265591402,-5.68136644548878,
151.229565777176));
#159306=CARTESIAN_POINT('Ctrl Pts',(17.9699637161583,-5.66659577633329,
151.230975467175));
#159307=CARTESIAN_POINT('Ctrl Pts',(18.0816307292424,-5.59777282493662,
151.234694595341));
#159308=CARTESIAN_POINT('Ctrl Pts',(18.274376104946,-5.46432194190647,151.218538751389));
#159309=CARTESIAN_POINT('Ctrl Pts',(18.5118820460989,-5.26934063561602,
151.145798229773));
#159310=CARTESIAN_POINT('Ctrl Pts',(18.7224658531959,-5.06521421683433,
151.01979784497));
#159311=CARTESIAN_POINT('Ctrl Pts',(18.8983183234987,-4.86277986153453,
150.839733266627));
#159312=CARTESIAN_POINT('Ctrl Pts',(19.0316797298042,-4.67617937190132,
150.606963224139));
#159313=CARTESIAN_POINT('Ctrl Pts',(19.1158310094995,-4.52247914657655,
150.326911047139));
#159314=CARTESIAN_POINT('Ctrl Pts',(19.1458603127157,-4.4192415037174,150.011520850732));
#159315=CARTESIAN_POINT('Ctrl Pts',(19.1258473951864,-4.38916359743563,
149.755721082763));
#159316=CARTESIAN_POINT('Ctrl Pts',(19.0992158962855,-4.39200367109623,
149.613897663077));
#159317=CARTESIAN_POINT('Ctrl Pts',(19.0920562581333,-4.39379506526226,
149.580569593459));
#159318=CARTESIAN_POINT('Ctrl Pts',(17.8767193898592,-5.71154921833711,
150.861222724773));
#159319=CARTESIAN_POINT('Ctrl Pts',(17.8983008572918,-5.70224569438056,
150.86226770474));
#159320=CARTESIAN_POINT('Ctrl Pts',(17.9961160866383,-5.65879160865082,
150.865343185256));
#159321=CARTESIAN_POINT('Ctrl Pts',(18.1656197374524,-5.57343226026813,
150.8561378627));
#159322=CARTESIAN_POINT('Ctrl Pts',(18.3802817903841,-5.44379286700894,
150.808030716389));
#159323=CARTESIAN_POINT('Ctrl Pts',(18.5769758391995,-5.30301381326858,
150.720829569143));
#159324=CARTESIAN_POINT('Ctrl Pts',(18.7486895990784,-5.15794570622578,
150.591209998157));
#159325=CARTESIAN_POINT('Ctrl Pts',(18.8863142702363,-5.01945224373198,
150.418173801994));
#159326=CARTESIAN_POINT('Ctrl Pts',(18.9807367833996,-4.90191979379112,
150.204179494235));
#159327=CARTESIAN_POINT('Ctrl Pts',(19.0239711438131,-4.82149176558256,
149.958929257427));
#159328=CARTESIAN_POINT('Ctrl Pts',(19.0143749134135,-4.79837244989064,
149.758210007737));
#159329=CARTESIAN_POINT('Ctrl Pts',(18.9934273279386,-4.80119830885926,
149.647926848569));
#159330=CARTESIAN_POINT('Ctrl Pts',(18.9875990235869,-4.80276154379444,
149.622099476749));
#159331=CARTESIAN_POINT('Origin',(18.4005666698389,-4.63611527055336,149.806488332022));
#159332=CARTESIAN_POINT('Origin',(16.5749874807289,-4.63611527055335,139.453114266522));
#159333=CARTESIAN_POINT('',(15.202263756867,-3.70950744065599,129.683973252045));
#159334=CARTESIAN_POINT('',(18.6178095147825,-4.04281182632481,149.768159429233));
#159335=CARTESIAN_POINT('Origin',(14.9369722812793,-4.63608791228591,130.064673259349));
#159336=CARTESIAN_POINT('Ctrl Pts',(15.6326354081712,0.0908296618712509,
137.316474337295));
#159337=CARTESIAN_POINT('Ctrl Pts',(15.8266313658842,0.0821951493031128,
137.044680273464));
#159338=CARTESIAN_POINT('Ctrl Pts',(16.0206273235873,0.0735606367349667,
136.772886209534));
#159339=CARTESIAN_POINT('Ctrl Pts',(16.2146232813003,0.0649261241668086,
136.501092145703));
#159340=CARTESIAN_POINT('Ctrl Pts',(15.6339880746382,-0.0834675886911582,
137.323205056148));
#159341=CARTESIAN_POINT('Ctrl Pts',(15.8278573503132,-0.0770410283918743,
137.050831116014));
#159342=CARTESIAN_POINT('Ctrl Pts',(16.0217266259883,-0.0706144680925627,
136.778457175779));
#159343=CARTESIAN_POINT('Ctrl Pts',(16.2155959016633,-0.0641879077932888,
136.506083235644));
#159344=CARTESIAN_POINT('Ctrl Pts',(15.6309087180474,-0.490284867328187,
137.299711347775));
#159345=CARTESIAN_POINT('Ctrl Pts',(15.8250778738318,-0.448705023318383,
137.029361549055));
#159346=CARTESIAN_POINT('Ctrl Pts',(16.0192470296262,-0.407125179308591,
136.759011750435));
#159347=CARTESIAN_POINT('Ctrl Pts',(16.2134161854106,-0.365545335298786,
136.488661951715));
#159348=CARTESIAN_POINT('Ctrl Pts',(15.6033825426741,-1.12583594967189,
137.120216729638));
#159349=CARTESIAN_POINT('Ctrl Pts',(15.8001894098461,-1.02933748521726,
136.865331428465));
#159350=CARTESIAN_POINT('Ctrl Pts',(15.9969962770082,-0.932839020763151,
136.610446127291));
#159351=CARTESIAN_POINT('Ctrl Pts',(16.1938031441802,-0.836340556308595,
136.355560826018));
#159352=CARTESIAN_POINT('Ctrl Pts',(15.5449483970485,-1.75570002821504,
136.746489385655));
#159353=CARTESIAN_POINT('Ctrl Pts',(15.7473444668466,-1.60477390395317,
136.523802803418));
#159354=CARTESIAN_POINT('Ctrl Pts',(15.9497405366547,-1.45384777969131,
136.30111622128));
#159355=CARTESIAN_POINT('Ctrl Pts',(16.1521366064528,-1.30292165543043,
136.078429639043));
#159356=CARTESIAN_POINT('Ctrl Pts',(15.4617593776569,-2.26668159677003,
136.218359273874));
#159357=CARTESIAN_POINT('Ctrl Pts',(15.6721069301266,-2.07160013148221,
136.041174053354));
#159358=CARTESIAN_POINT('Ctrl Pts',(15.8824544825962,-1.8765186661934,135.863988832833));
#159359=CARTESIAN_POINT('Ctrl Pts',(16.0928020350659,-1.68143720090556,
135.686803612212));
#159360=CARTESIAN_POINT('Ctrl Pts',(15.3618046767863,-2.6146082031803,135.58649639665));
#159361=CARTESIAN_POINT('Ctrl Pts',(15.5817024284862,-2.38946079206905,
135.46374967683));
#159362=CARTESIAN_POINT('Ctrl Pts',(15.8016001801861,-2.16431338095777,
135.341002956909));
#159363=CARTESIAN_POINT('Ctrl Pts',(16.021497931886,-1.93916596984552,135.218256237088));
#159364=CARTESIAN_POINT('Ctrl Pts',(15.2522266269535,-2.78470879606595,
134.895948354886));
#159365=CARTESIAN_POINT('Ctrl Pts',(15.4825910225606,-2.54486131186758,
134.832696174107));
#159366=CARTESIAN_POINT('Ctrl Pts',(15.7129554181676,-2.30501382766823,
134.769443993427));
#159367=CARTESIAN_POINT('Ctrl Pts',(15.9433198137746,-2.06516634346886,
134.706191812648));
#159368=CARTESIAN_POINT('Ctrl Pts',(15.1396605412371,-2.77118141126198,
134.188484376818));
#159369=CARTESIAN_POINT('Ctrl Pts',(15.3807742998572,-2.53250117447683,
134.186184123501));
#159370=CARTESIAN_POINT('Ctrl Pts',(15.6218880584774,-2.29382093769172,
134.183883870284));
#159371=CARTESIAN_POINT('Ctrl Pts',(15.8630018170975,-2.05514070090757,
134.181583616967));
#159372=CARTESIAN_POINT('Ctrl Pts',(15.0305921321479,-2.57491612832342,
133.504865240957));
#159373=CARTESIAN_POINT('Ctrl Pts',(15.2821186291523,-2.35319364293089,
133.561462537436));
#159374=CARTESIAN_POINT('Ctrl Pts',(15.5336451261467,-2.13147115753737,
133.618059833915));
#159375=CARTESIAN_POINT('Ctrl Pts',(15.7851716231411,-1.90974867214482,
133.674657130294));
#159376=CARTESIAN_POINT('Ctrl Pts',(14.9316301076284,-2.20286413122342,
132.886563257347));
#159377=CARTESIAN_POINT('Ctrl Pts',(15.1926017157584,-2.01328934411237,
132.996430657771));
#159378=CARTESIAN_POINT('Ctrl Pts',(15.4535733238983,-1.82371455700229,
133.106298058095));
#159379=CARTESIAN_POINT('Ctrl Pts',(15.7145449320382,-1.63413976989123,
133.216165458519));
#159380=CARTESIAN_POINT('Ctrl Pts',(14.849904498969,-1.67305154249018,132.378215214644));
#159381=CARTESIAN_POINT('Ctrl Pts',(15.1186729626689,-1.52925686142635,
132.531879568582));
#159382=CARTESIAN_POINT('Ctrl Pts',(15.3874414263788,-1.38546218036253,
132.68554392262));
#159383=CARTESIAN_POINT('Ctrl Pts',(15.6562098900787,-1.2416674992987,132.839208276557));
#159384=CARTESIAN_POINT('Ctrl Pts',(14.793162055357,-1.02580630728256,132.028107883375));
#159385=CARTESIAN_POINT('Ctrl Pts',(15.0673399157224,-0.937939500879029,
132.211935871462));
#159386=CARTESIAN_POINT('Ctrl Pts',(15.3415177760977,-0.85007269447598,
132.395763859549));
#159387=CARTESIAN_POINT('Ctrl Pts',(15.6156956364631,-0.762205888072875,
132.579591847736));
#159388=CARTESIAN_POINT('Ctrl Pts',(14.7690193246188,-0.429827561211837,
131.882404280965));
#159389=CARTESIAN_POINT('Ctrl Pts',(15.0454941881122,-0.393459152817816,
132.078785396901));
#159390=CARTESIAN_POINT('Ctrl Pts',(15.3219690516056,-0.357090744423894,
132.275166512837));
#159391=CARTESIAN_POINT('Ctrl Pts',(15.5984439150991,-0.320722336029973,
132.471547628773));
#159392=CARTESIAN_POINT('Ctrl Pts',(14.7661244244312,-0.0562448076138019,
131.868005288716));
#159393=CARTESIAN_POINT('Ctrl Pts',(15.0428703976198,-0.0521577867173374,
132.065626930907));
#159394=CARTESIAN_POINT('Ctrl Pts',(15.3196163708083,-0.0480707658208829,
132.263248573098));
#159395=CARTESIAN_POINT('Ctrl Pts',(15.5963623440068,-0.0439837449244126,
132.460870215289));
#159396=CARTESIAN_POINT('Ctrl Pts',(14.7667334772298,0.0886098244785636,
131.873306754642));
#159397=CARTESIAN_POINT('Ctrl Pts',(15.0434192179426,0.0801798916379546,
132.070471636069));
#159398=CARTESIAN_POINT('Ctrl Pts',(15.3201049586553,0.0717499587973433,
132.267636517396));
#159399=CARTESIAN_POINT('Ctrl Pts',(15.596790699368,0.0633200259567142,
132.464801398824));
#159400=CARTESIAN_POINT('',(15.7204620888588,-0.013326943698867,137.195385296531));
#159401=CARTESIAN_POINT('Origin',(227.634194189643,0.131638934550563,287.921260411963));
#159402=CARTESIAN_POINT('',(14.8912321715194,-0.0131815370763207,131.959834448354));
#159403=CARTESIAN_POINT('Origin',(168.294554533299,0.439697821287936,-82.4898013238501));
#159404=CARTESIAN_POINT('Ctrl Pts',(15.7205398917825,-0.0133270177734878,
137.195877603114));
#159405=CARTESIAN_POINT('Ctrl Pts',(15.7210832648335,-0.362848575696153,
137.195739139215));
#159406=CARTESIAN_POINT('Ctrl Pts',(15.7105102208732,-0.714886006099241,
137.125388679336));
#159407=CARTESIAN_POINT('Ctrl Pts',(15.6729215390833,-1.30198405806983,
136.882067817117));
#159408=CARTESIAN_POINT('Ctrl Pts',(15.6454643677425,-1.60729537011807,
136.705592307119));
#159409=CARTESIAN_POINT('Ctrl Pts',(15.5631895994256,-2.13639793975214,
136.180726786475));
#159410=CARTESIAN_POINT('Ctrl Pts',(15.5178003232202,-2.33085785365462,
135.892164379888));
#159411=CARTESIAN_POINT('Ctrl Pts',(15.4177062562099,-2.59550999840174,
135.25749269031));
#159412=CARTESIAN_POINT('Ctrl Pts',(15.3641108455972,-2.66344085160448,
134.918410851475));
#159413=CARTESIAN_POINT('Ctrl Pts',(15.2555256364223,-2.66303508426177,
134.232834867303));
#159414=CARTESIAN_POINT('Ctrl Pts',(15.2017550777324,-2.59480606967409,
133.894037601806));
#159415=CARTESIAN_POINT('Ctrl Pts',(15.1011070518146,-2.33030164433699,
133.261271906951));
#159416=CARTESIAN_POINT('Ctrl Pts',(15.055158835653,-2.13624050986265,132.973147927333));
#159417=CARTESIAN_POINT('Ctrl Pts',(14.9700712795838,-1.5999752670426,132.44140230918));
#159418=CARTESIAN_POINT('Ctrl Pts',(14.9422731326707,-1.29173136487026,
132.269039366159));
#159419=CARTESIAN_POINT('Ctrl Pts',(14.9140989162941,-0.874949693559167,
132.095410361788));
#159420=CARTESIAN_POINT('Ctrl Pts',(14.9056757258523,-0.705283371614432,
132.043960993393));
#159421=CARTESIAN_POINT('Ctrl Pts',(14.8944282106145,-0.360086125972263,
131.976471995303));
#159422=CARTESIAN_POINT('Ctrl Pts',(14.8915614467703,-0.187041438110135,
131.960139027468));
#159423=CARTESIAN_POINT('Ctrl Pts',(14.8913098915074,-0.0131819538729922,
131.960326159532));
#159424=CARTESIAN_POINT('Ctrl Pts',(14.766880881743,-0.117682776752729,
131.872322017485));
#159425=CARTESIAN_POINT('Ctrl Pts',(15.0435746463364,-0.108286228136295,
132.06958563023));
#159426=CARTESIAN_POINT('Ctrl Pts',(15.3202684109298,-0.0988896795198714,
132.266849242975));
#159427=CARTESIAN_POINT('Ctrl Pts',(15.5969621755232,-0.0894931309034575,
132.46411285572));
#159428=CARTESIAN_POINT('Ctrl Pts',(14.7655281944518,0.0566164276715459,
131.865591195374));
#159429=CARTESIAN_POINT('Ctrl Pts',(15.0423486518352,0.0509506755153907,
132.063434734082));
#159430=CARTESIAN_POINT('Ctrl Pts',(15.3191691092286,0.0452849233592512,
132.261278272791));
#159431=CARTESIAN_POINT('Ctrl Pts',(15.5959895666119,0.0396191712030961,
132.459121811499));
#159432=CARTESIAN_POINT('Ctrl Pts',(14.7686075831621,0.463438098286559,
131.889085123866));
#159433=CARTESIAN_POINT('Ctrl Pts',(15.0451281366027,0.422616210984097,
132.084904359668));
#159434=CARTESIAN_POINT('Ctrl Pts',(15.3216486900533,0.381794323681724,
132.280723595571));
#159435=CARTESIAN_POINT('Ctrl Pts',(15.5981692434938,0.340972436379235,
132.476542831474));
#159436=CARTESIAN_POINT('Ctrl Pts',(14.7961340834777,1.09899596056801,132.068581651183));
#159437=CARTESIAN_POINT('Ctrl Pts',(15.0700167119187,1.00325100517306,132.248935137205));
#159438=CARTESIAN_POINT('Ctrl Pts',(15.3438993403696,0.907506049779131,
132.429288623227));
#159439=CARTESIAN_POINT('Ctrl Pts',(15.6177819688205,0.811761094384798,
132.60964210925));
#159440=CARTESIAN_POINT('Ctrl Pts',(14.8545689042686,1.72886661379578,132.44231288469));
#159441=CARTESIAN_POINT('Ctrl Pts',(15.1228618787092,1.57868960320719,132.590465051457));
#159442=CARTESIAN_POINT('Ctrl Pts',(15.3911548531599,1.42851259261963,132.738617218224));
#159443=CARTESIAN_POINT('Ctrl Pts',(15.6594478276006,1.27833558203105,132.886769384991));
#159444=CARTESIAN_POINT('Ctrl Pts',(14.9377588841678,2.23985351617292,132.970448492951));
#159445=CARTESIAN_POINT('Ctrl Pts',(15.1980997338175,2.04551759872797,133.073095623512));
#159446=CARTESIAN_POINT('Ctrl Pts',(15.4584405834572,1.851181681283,133.175742754073));
#159447=CARTESIAN_POINT('Ctrl Pts',(15.7187814331068,1.65684576383804,133.278389884633));
#159448=CARTESIAN_POINT('Ctrl Pts',(15.037714738664,2.58778375445155,133.602317946183));
#159449=CARTESIAN_POINT('Ctrl Pts',(15.2885046178437,2.36337946316326,133.65052217977));
#159450=CARTESIAN_POINT('Ctrl Pts',(15.5392944970234,2.13897517187496,133.698726413357));
#159451=CARTESIAN_POINT('Ctrl Pts',(15.7900843762032,1.91457088058667,133.746930646944));
#159452=CARTESIAN_POINT('Ctrl Pts',(15.1472940528428,2.75788612305896,134.292873174639));
#159453=CARTESIAN_POINT('Ctrl Pts',(15.3876164428632,2.51878057155707,134.281578064556));
#159454=CARTESIAN_POINT('Ctrl Pts',(15.6279388328837,2.27967502005419,134.270282954472));
#159455=CARTESIAN_POINT('Ctrl Pts',(15.8682612228942,2.04056946855229,134.258987844389));
#159456=CARTESIAN_POINT('Ctrl Pts',(15.2598614370511,2.74435859725416,135.000344515569));
#159457=CARTESIAN_POINT('Ctrl Pts',(15.4894335959701,2.50642038742937,134.928092555749));
#159458=CARTESIAN_POINT('Ctrl Pts',(15.7190057548991,2.2684821776046,134.855840595929));
#159459=CARTESIAN_POINT('Ctrl Pts',(15.9485779138282,2.03054396777882,134.783588636109));
#159460=CARTESIAN_POINT('Ctrl Pts',(15.3689311039534,2.54809126587522,135.683970765961));
#159461=CARTESIAN_POINT('Ctrl Pts',(15.5880896836034,2.32711217689028,135.552816500125));
#159462=CARTESIAN_POINT('Ctrl Pts',(15.8072482632634,2.10613308790537,135.42166223419));
#159463=CARTESIAN_POINT('Ctrl Pts',(16.0264068429134,1.88515399892043,135.290507968354));
#159464=CARTESIAN_POINT('Ctrl Pts',(15.4678942694229,2.17603538543718,136.302279184494));
#159465=CARTESIAN_POINT('Ctrl Pts',(15.6776069751826,1.98720659087041,136.117850512733));
#159466=CARTESIAN_POINT('Ctrl Pts',(15.8873196809323,1.79837779630263,135.933421840973));
#159467=CARTESIAN_POINT('Ctrl Pts',(16.097032386692,1.60954900173483,135.748993169312));
#159468=CARTESIAN_POINT('Ctrl Pts',(15.5496208199135,1.64621726661601,136.810632517662));
#159469=CARTESIAN_POINT('Ctrl Pts',(15.7515360404562,1.50317227513574,136.582403355514));
#159470=CARTESIAN_POINT('Ctrl Pts',(15.9534512609989,1.36012728365549,136.354174193265));
#159471=CARTESIAN_POINT('Ctrl Pts',(16.1553664815517,1.21708229217522,136.125945031116));
#159472=CARTESIAN_POINT('Ctrl Pts',(15.6063639169654,0.998965275500975,
137.160743492757));
#159473=CARTESIAN_POINT('Ctrl Pts',(15.8028693039962,0.911852675220866,
136.902348260412));
#159474=CARTESIAN_POINT('Ctrl Pts',(15.9993746910371,0.824740074940445,
136.643953028167));
#159475=CARTESIAN_POINT('Ctrl Pts',(16.1958800780679,0.737627474659937,
136.385557795822));
#159476=CARTESIAN_POINT('Ctrl Pts',(15.6305069308838,0.40298016741526,137.306448645902));
#159477=CARTESIAN_POINT('Ctrl Pts',(15.8247151287538,0.367370136173505,
137.035499269165));
#159478=CARTESIAN_POINT('Ctrl Pts',(16.0189233266237,0.331760104931878,
136.764549892329));
#159479=CARTESIAN_POINT('Ctrl Pts',(16.2131315244937,0.29615007369015,136.493600515492));
#159480=CARTESIAN_POINT('Ctrl Pts',(15.6334018603134,0.0293933703536851,
137.320847764629));
#159481=CARTESIAN_POINT('Ctrl Pts',(15.8273389269369,0.026067345982975,
137.048657763365));
#159482=CARTESIAN_POINT('Ctrl Pts',(16.0212759935504,0.0227413216122492,
136.7764677621));
#159483=CARTESIAN_POINT('Ctrl Pts',(16.2152130601639,0.0194152972415234,
136.504277760835));
#159484=CARTESIAN_POINT('Ctrl Pts',(15.6327927962462,-0.11546291508241,
137.315546216845));
#159485=CARTESIAN_POINT('Ctrl Pts',(15.8267901005858,-0.106270962677035,
137.043813015627));
#159486=CARTESIAN_POINT('Ctrl Pts',(16.0207874049254,-0.0970790102716011,
136.77207981431));
#159487=CARTESIAN_POINT('Ctrl Pts',(16.214784709265,-0.0878870578661855,
136.500346613092));
#159488=CARTESIAN_POINT('Ctrl Pts',(14.8911540502061,-0.0131814635361809,
131.959342221145));
#159489=CARTESIAN_POINT('Ctrl Pts',(14.8906106762576,0.336340102835657,
131.959480679464));
#159490=CARTESIAN_POINT('Ctrl Pts',(14.901183720497,0.688377558217891,132.029831141429));
#159491=CARTESIAN_POINT('Ctrl Pts',(14.938772402906,1.275475620005,132.273152007657));
#159492=CARTESIAN_POINT('Ctrl Pts',(14.9662295743078,1.58078693156106,132.44962751801));
#159493=CARTESIAN_POINT('Ctrl Pts',(15.0485043424753,2.10988950019956,132.974493037701));
#159494=CARTESIAN_POINT('Ctrl Pts',(15.0938936187016,2.30434941420721,133.26305544435));
#159495=CARTESIAN_POINT('Ctrl Pts',(15.1939876857224,2.56900155900805,133.897727133996));
#159496=CARTESIAN_POINT('Ctrl Pts',(15.2475830963336,2.63693241219933,134.236808972806));
#159497=CARTESIAN_POINT('Ctrl Pts',(15.3561683054966,2.63652664485352,134.922384956904));
#159498=CARTESIAN_POINT('Ctrl Pts',(15.4099388641883,2.56829763029012,135.261182222416));
#159499=CARTESIAN_POINT('Ctrl Pts',(15.5105868901176,2.30379320491567,135.893947917343));
#159500=CARTESIAN_POINT('Ctrl Pts',(15.5565351062835,2.10973207046068,136.182071896982));
#159501=CARTESIAN_POINT('Ctrl Pts',(15.6416226623923,1.57346682728598,136.713817515381));
#159502=CARTESIAN_POINT('Ctrl Pts',(15.669420809299,1.26522292492855,136.886180458388));
#159503=CARTESIAN_POINT('Ctrl Pts',(15.6975949609052,0.848442211693935,
137.059809063598));
#159504=CARTESIAN_POINT('Ctrl Pts',(15.7060181182242,0.678776904425043,
137.11125823324));
#159505=CARTESIAN_POINT('Ctrl Pts',(15.7172656973454,0.333579735722459,
137.178747635459));
#159506=CARTESIAN_POINT('Ctrl Pts',(15.7201324941116,0.160534015214026,
137.195080800611));
#159507=CARTESIAN_POINT('Ctrl Pts',(15.7203840504836,-0.0133265274405875,
137.194893664742));
#159508=CARTESIAN_POINT('Origin',(17.3095324658322,2.73849310306822,139.655633390962));
#159509=CARTESIAN_POINT('',(14.6493737823773,2.73685851198427,130.460883875229));
#159510=CARTESIAN_POINT('',(14.6493737823824,2.73685851198428,130.460883875214));
#159511=CARTESIAN_POINT('',(15.190628493629,3.68536951497202,129.686024863033));
#159512=CARTESIAN_POINT('',(18.605126018521,4.01827620696241,149.770395858136));
#159513=CARTESIAN_POINT('Origin',(15.465028260172,2.73846506067834,129.296006976405));
#159514=CARTESIAN_POINT('Origin',(14.4423646123641,2.73689541022749,129.153879602933));
#159515=CARTESIAN_POINT('',(14.6580275938616,-2.76313446829959,130.459357973818));
#159516=CARTESIAN_POINT('',(14.6580275938631,-2.76313446829959,130.459357973838));
#159517=CARTESIAN_POINT('',(17.7407389282425,-2.76368394498376,149.922828525115));
#159518=CARTESIAN_POINT('',(14.6493737823824,2.73685851198428,130.460883875214));
#159519=CARTESIAN_POINT('Origin',(17.3181862774528,-2.76149987721566,139.654107490386));
#159520=CARTESIAN_POINT('Origin',(15.4736820716518,-2.76152791963452,129.294481074998));
#159521=CARTESIAN_POINT('Origin',(16.2596385318791,-3.0395155659729,150.157404029166));
#159522=CARTESIAN_POINT('',(16.5196805691196,-2.76608012003402,151.634691519722));
#159523=CARTESIAN_POINT('Ctrl Pts',(17.8587892544387,5.68406649606213,150.864384285181));
#159524=CARTESIAN_POINT('Ctrl Pts',(17.8803999009861,5.67483034719617,150.86542412206));
#159525=CARTESIAN_POINT('Ctrl Pts',(17.9783508188883,5.63168282830363,150.868475560104));
#159526=CARTESIAN_POINT('Ctrl Pts',(18.1481232811645,5.54686197137129,150.859223056995));
#159527=CARTESIAN_POINT('Ctrl Pts',(18.3631933945532,5.41792464037205,150.811043805684));
#159528=CARTESIAN_POINT('Ctrl Pts',(18.5603311747761,5.27781203285765,150.723763167653));
#159529=CARTESIAN_POINT('Ctrl Pts',(18.7325001095741,5.13335675005504,150.594062243622));
#159530=CARTESIAN_POINT('Ctrl Pts',(18.8705588995167,4.9953934251543,150.420948432272));
#159531=CARTESIAN_POINT('Ctrl Pts',(18.9653527121365,4.87827436336384,150.206882039047));
#159532=CARTESIAN_POINT('Ctrl Pts',(19.0088360698327,4.79812181747546,149.961586023878));
#159533=CARTESIAN_POINT('Ctrl Pts',(18.9993099063281,4.77508671018202,149.760856024253));
#159534=CARTESIAN_POINT('Ctrl Pts',(18.9783553383453,4.77790752850252,149.650584360981));
#159535=CARTESIAN_POINT('Ctrl Pts',(18.9725221022922,4.77946670473843,149.624757783732));
#159536=CARTESIAN_POINT('Ctrl Pts',(17.9274913897233,5.65389539357561,151.232710594697));
#159537=CARTESIAN_POINT('Ctrl Pts',(17.9521749134293,5.63920153970202,151.234112111453));
#159538=CARTESIAN_POINT('Ctrl Pts',(18.0640572892245,5.57072866697129,151.237793130604));
#159539=CARTESIAN_POINT('Ctrl Pts',(18.2572228552344,5.43789323666701,151.221563446129));
#159540=CARTESIAN_POINT('Ctrl Pts',(18.4953424478875,5.24369949655056,151.148714398131));
#159541=CARTESIAN_POINT('Ctrl Pts',(18.7065692305997,5.0403044694732,151.02259877758));
#159542=CARTESIAN_POINT('Ctrl Pts',(18.8830571520153,4.83852431651492,150.842420720756));
#159543=CARTESIAN_POINT('Ctrl Pts',(19.0170038617902,4.65247420324261,150.609546302775));
#159544=CARTESIAN_POINT('Ctrl Pts',(19.1016398885586,4.49919095857635,150.329399715761));
#159545=CARTESIAN_POINT('Ctrl Pts',(19.131989851798,4.39622729952393,150.013951395625));
#159546=CARTESIAN_POINT('Ctrl Pts',(19.1120690066584,4.36623211354187,149.75813710317));
#159547=CARTESIAN_POINT('Ctrl Pts',(19.0854310415134,4.36906675560282,149.616328332059));
#159548=CARTESIAN_POINT('Ctrl Pts',(19.078265766194,4.37085406194063,149.583001271904));
#159549=CARTESIAN_POINT('Ctrl Pts',(17.8345625406965,5.38166643196077,151.474669762255));
#159550=CARTESIAN_POINT('Ctrl Pts',(17.859674084597,5.36307109482329,151.473955637923));
#159551=CARTESIAN_POINT('Ctrl Pts',(17.9731032668532,5.27717402724323,151.46726152533));
#159552=CARTESIAN_POINT('Ctrl Pts',(18.1652088286427,5.11649686441713,151.427323582462));
#159553=CARTESIAN_POINT('Ctrl Pts',(18.3919267981537,4.89446435532081,151.316369237397));
#159554=CARTESIAN_POINT('Ctrl Pts',(18.5825501347808,4.67396298072739,151.150374696084));
#159555=CARTESIAN_POINT('Ctrl Pts',(18.7313420940797,4.46622141098541,150.933763687288));
#159556=CARTESIAN_POINT('Ctrl Pts',(18.8345887567204,4.2838265090382,150.672616487709));
#159557=CARTESIAN_POINT('Ctrl Pts',(18.8908467441566,4.13990089484537,150.375698246391));
#159558=CARTESIAN_POINT('Ctrl Pts',(18.900833820193,4.04610736667316,150.054876766821));
#159559=CARTESIAN_POINT('Ctrl Pts',(18.8745260848819,4.01856092057753,149.800018647566));
#159560=CARTESIAN_POINT('Ctrl Pts',(18.847950180088,4.02039035674692,149.658196016061));
#159561=CARTESIAN_POINT('Ctrl Pts',(18.8410067777837,4.02180896773098,149.624787894765));
#159562=CARTESIAN_POINT('Ctrl Pts',(17.6462260514748,5.06137654967593,151.417835836187));
#159563=CARTESIAN_POINT('Ctrl Pts',(17.6688157410725,5.043216242298,151.414036406879));
#159564=CARTESIAN_POINT('Ctrl Pts',(17.7703047866832,4.96021304129056,151.393356019318));
#159565=CARTESIAN_POINT('Ctrl Pts',(17.9376526209387,4.81170767838965,151.329873819149));
#159566=CARTESIAN_POINT('Ctrl Pts',(18.1266429371576,4.61909262015257,151.194533432453));
#159567=CARTESIAN_POINT('Ctrl Pts',(18.2766528928194,4.4398513668303,151.016034714885));
#159568=CARTESIAN_POINT('Ctrl Pts',(18.385470753359,4.28176008337927,150.80299793715));
#159569=CARTESIAN_POINT('Ctrl Pts',(18.4533069975848,4.15215760050746,150.56521364884));
#159570=CARTESIAN_POINT('Ctrl Pts',(18.4831895690037,4.05644295646414,150.312784178972));
#159571=CARTESIAN_POINT('Ctrl Pts',(18.4800953507138,3.99726594629036,150.055197728674));
#159572=CARTESIAN_POINT('Ctrl Pts',(18.4559599690146,3.97983202742149,149.856654856497));
#159573=CARTESIAN_POINT('Ctrl Pts',(18.4351473563841,3.98035356208065,149.746351489287));
#159574=CARTESIAN_POINT('Ctrl Pts',(18.4298216273155,3.98106939347749,149.720339494746));
#159575=CARTESIAN_POINT('',(19.0093911677908,4.61188418703687,149.699165991196));
#159576=CARTESIAN_POINT('Ctrl Pts',(19.0093911677908,4.61188418703687,149.699165991196));
#159577=CARTESIAN_POINT('Ctrl Pts',(19.015500537071,4.61189015756661,149.737727855937));
#159578=CARTESIAN_POINT('Ctrl Pts',(19.0201475819771,4.61250126401147,149.776952028307));
#159579=CARTESIAN_POINT('Ctrl Pts',(19.0232524053809,4.61375762212829,149.816717483555));
#159580=CARTESIAN_POINT('Ctrl Pts',(19.0262253202089,4.61496060380839,149.854793501472));
#159581=CARTESIAN_POINT('Ctrl Pts',(19.0277840966013,4.6167552738848,149.893366191926));
#159582=CARTESIAN_POINT('Ctrl Pts',(19.0278298377205,4.61918822443702,149.932292573303));
#159583=CARTESIAN_POINT('Ctrl Pts',(19.0278487031587,4.62019166902332,149.948347345408));
#159584=CARTESIAN_POINT('Ctrl Pts',(19.0276098584352,4.62130381811468,149.964461804004));
#159585=CARTESIAN_POINT('Ctrl Pts',(19.0271049749971,4.62252845771671,149.980623754727));
#159586=CARTESIAN_POINT('Ctrl Pts',(19.0258742772302,4.62551362441027,150.020019930486));
#159587=CARTESIAN_POINT('Ctrl Pts',(19.0230642858215,4.62916769373579,150.059701359999));
#159588=CARTESIAN_POINT('Ctrl Pts',(19.0186172197646,4.63343797107301,150.099587736542));
#159589=CARTESIAN_POINT('Ctrl Pts',(19.0143834314118,4.63750344935059,150.13756119461));
#159590=CARTESIAN_POINT('Ctrl Pts',(19.0086656935405,4.64212756637824,150.175720699002));
#159591=CARTESIAN_POINT('Ctrl Pts',(19.0013950309014,4.64725969649565,150.213953205714));
#159592=CARTESIAN_POINT('Ctrl Pts',(18.9993908405042,4.64867439092024,150.224492165726));
#159593=CARTESIAN_POINT('Ctrl Pts',(18.9972685407139,4.65012765023049,150.235036393758));
#159594=CARTESIAN_POINT('Ctrl Pts',(18.9950264368246,4.65161832543263,150.24558286292));
#159595=CARTESIAN_POINT('Ctrl Pts',(18.9937878121247,4.65244183193189,150.25140913942));
#159596=CARTESIAN_POINT('Ctrl Pts',(18.9925127279385,4.65327790659982,150.257235578971));
#159597=CARTESIAN_POINT('Ctrl Pts',(18.9912009357774,4.65412666248646,150.263061494053));
#159598=CARTESIAN_POINT('Ctrl Pts',(18.9827757632883,4.65957791837774,150.300479265654));
#159599=CARTESIAN_POINT('Ctrl Pts',(18.9728361281526,4.66555347237378,150.337879447222));
#159600=CARTESIAN_POINT('Ctrl Pts',(18.9613462365199,4.67206205203735,150.375156989378));
#159601=CARTESIAN_POINT('Ctrl Pts',(18.9497081013584,4.67865460593218,150.412915489456));
#159602=CARTESIAN_POINT('Ctrl Pts',(18.9364791401498,4.68579407471151,150.45054810867));
#159603=CARTESIAN_POINT('Ctrl Pts',(18.9216280703525,4.69347387927701,150.487894341172));
#159604=CARTESIAN_POINT('Ctrl Pts',(18.9167497883694,4.69599654281281,150.500161838102));
#159605=CARTESIAN_POINT('Ctrl Pts',(18.9116965481905,4.69857738253454,150.512398033371));
#159606=CARTESIAN_POINT('Ctrl Pts',(18.9064674538662,4.70121580877459,150.524596100463));
#159607=CARTESIAN_POINT('Ctrl Pts',(18.9046851887652,4.70211508018138,150.528753644376));
#159608=CARTESIAN_POINT('Ctrl Pts',(18.9028823913324,4.70302114824624,150.532906997649));
#159609=CARTESIAN_POINT('Ctrl Pts',(18.9010590312277,4.70393398011984,150.537055854138));
#159610=CARTESIAN_POINT('Ctrl Pts',(18.8844178728109,4.71226507159056,150.574920990003));
#159611=CARTESIAN_POINT('Ctrl Pts',(18.8660619770264,4.72116147974709,150.612414949923));
#159612=CARTESIAN_POINT('Ctrl Pts',(18.8459853786395,4.73062400119261,150.649374483313));
#159613=CARTESIAN_POINT('Ctrl Pts',(18.8440014796444,4.73155905435378,150.653026694695));
#159614=CARTESIAN_POINT('Ctrl Pts',(18.8420007978559,4.73249961695326,150.656673655371));
#159615=CARTESIAN_POINT('Ctrl Pts',(18.8399833403143,4.73344567777125,150.66031518714));
#159616=CARTESIAN_POINT('Ctrl Pts',(18.8276480154341,4.73923017003751,150.682580576375));
#159617=CARTESIAN_POINT('Ctrl Pts',(18.8146848936636,4.74522109248284,150.704644275892));
#159618=CARTESIAN_POINT('Ctrl Pts',(18.8010939409842,4.75141845499668,150.726467622821));
#159619=CARTESIAN_POINT('Ctrl Pts',(18.7942984646446,4.7545171362536,150.737379296286));
#159620=CARTESIAN_POINT('Ctrl Pts',(18.7873460194151,4.75766742751596,150.748230877052));
#159621=CARTESIAN_POINT('Ctrl Pts',(18.7802366479733,4.76086933028016,150.759017273877));
#159622=CARTESIAN_POINT('Ctrl Pts',(18.7766819622525,4.76247028166226,150.76441047229));
#159623=CARTESIAN_POINT('Ctrl Pts',(18.7730880441955,4.76408413592108,150.76978737374));
#159624=CARTESIAN_POINT('Ctrl Pts',(18.7694548974234,4.76571089325153,150.77514732952));
#159625=CARTESIAN_POINT('Ctrl Pts',(18.7676383240373,4.76652427191676,150.77782730741));
#159626=CARTESIAN_POINT('Ctrl Pts',(18.765811943414,4.76734087634984,150.780503048798));
#159627=CARTESIAN_POINT('Ctrl Pts',(18.7639757561209,4.7681607065754,150.783174471373));
#159628=CARTESIAN_POINT('Ctrl Pts',(18.7624282261282,4.76885165562388,150.785425933722));
#159629=CARTESIAN_POINT('Ctrl Pts',(18.7603436660376,4.76978089534062,150.78843756471));
#159630=CARTESIAN_POINT('Ctrl Pts',(18.7590620273306,4.77035184413092,150.790279324772));
#159631=CARTESIAN_POINT('Ctrl Pts',(18.7589283971141,4.77041137417634,150.79047135611));
#159632=CARTESIAN_POINT('Ctrl Pts',(18.7588035288813,4.77046699410134,150.79065069989));
#159633=CARTESIAN_POINT('Ctrl Pts',(18.7586889603557,4.77051801916076,150.790815185756));
#159634=CARTESIAN_POINT('Ctrl Pts',(18.758598568586,4.77055827668696,150.790944961089));
#159635=CARTESIAN_POINT('Ctrl Pts',(18.7585145882522,4.77059567396844,150.791065487676));
#159636=CARTESIAN_POINT('Ctrl Pts',(18.7584377747101,4.77062987465357,150.791175699747));
#159637=CARTESIAN_POINT('Ctrl Pts',(18.7427442375651,4.77761731083079,150.813692786982));
#159638=CARTESIAN_POINT('Ctrl Pts',(18.7254013610764,4.78529673082924,150.837260032547));
#159639=CARTESIAN_POINT('Ctrl Pts',(18.7061931998337,4.79370349912867,150.861643479064));
#159640=CARTESIAN_POINT('Ctrl Pts',(18.6872953200397,4.8019744676389,150.885633044512));
#159641=CARTESIAN_POINT('Ctrl Pts',(18.6665914498066,4.81095000020678,150.910413063444));
#159642=CARTESIAN_POINT('Ctrl Pts',(18.643873611093,4.82064367917762,150.935713037193));
#159643=CARTESIAN_POINT('Ctrl Pts',(18.622699857766,4.82967849846426,150.959293423077));
#159644=CARTESIAN_POINT('Ctrl Pts',(18.599776322654,4.83933724842325,150.983325470976));
#159645=CARTESIAN_POINT('Ctrl Pts',(18.5749379084155,4.8496093691693,151.007546322188));
#159646=CARTESIAN_POINT('Ctrl Pts',(18.5731265794623,4.85035845844448,151.009312615666));
#159647=CARTESIAN_POINT('Ctrl Pts',(18.5713050697243,4.8511107992961,151.01107989255));
#159648=CARTESIAN_POINT('Ctrl Pts',(18.5694733164477,4.85186638268389,151.01284804095));
#159649=CARTESIAN_POINT('Ctrl Pts',(18.5449558796609,4.86197962674588,151.036514146632));
#159650=CARTESIAN_POINT('Ctrl Pts',(18.5186020159773,4.87267515880367,151.060339859999));
#159651=CARTESIAN_POINT('Ctrl Pts',(18.4902680732814,4.88394610973416,151.084046519532));
#159652=CARTESIAN_POINT('Ctrl Pts',(18.4695156567062,4.89220120756575,151.101409809898));
#159653=CARTESIAN_POINT('Ctrl Pts',(18.4477012785905,4.90076466329986,151.118708449806));
#159654=CARTESIAN_POINT('Ctrl Pts',(18.4247751170454,4.9096275470227,151.135817514645));
#159655=CARTESIAN_POINT('Ctrl Pts',(18.3977740609141,4.92006571917003,151.15596754365));
#159656=CARTESIAN_POINT('Ctrl Pts',(18.3692092526384,4.93093761255334,151.175870517343));
#159657=CARTESIAN_POINT('Ctrl Pts',(18.3390315397969,4.9422482518405,151.195279017778));
#159658=CARTESIAN_POINT('Ctrl Pts',(18.3071202020531,4.95420865560889,151.215802482089));
#159659=CARTESIAN_POINT('Ctrl Pts',(18.2734038260656,4.9666600997838,151.235772955197));
#159660=CARTESIAN_POINT('Ctrl Pts',(18.2378719169443,4.97960093312966,151.254877447792));
#159661=CARTESIAN_POINT('Ctrl Pts',(18.2029890326836,4.99230538957466,151.273632978257));
#159662=CARTESIAN_POINT('Ctrl Pts',(18.1663563212283,5.00548163002252,151.291553943544));
#159663=CARTESIAN_POINT('Ctrl Pts',(18.1280017693888,5.01910706906789,151.308318507699));
#159664=CARTESIAN_POINT('Ctrl Pts',(18.1106764072625,5.02526189696367,151.315891328419));
#159665=CARTESIAN_POINT('Ctrl Pts',(18.0930002284209,5.03150808482261,151.323227830964));
#159666=CARTESIAN_POINT('Ctrl Pts',(18.0749783669678,5.03784204093478,151.330296483783));
#159667=CARTESIAN_POINT('Ctrl Pts',(18.0274749294532,5.05453757980443,151.348928593923));
#159668=CARTESIAN_POINT('Ctrl Pts',(17.9775661933698,5.07184209113894,151.365699921857));
#159669=CARTESIAN_POINT('Ctrl Pts',(17.9252952106596,5.0898080436658,151.380080876025));
#159670=CARTESIAN_POINT('Ctrl Pts',(17.8810599546647,5.10501205300352,151.392251016247));
#159671=CARTESIAN_POINT('Ctrl Pts',(17.8351346574171,5.12068951564457,151.40270901121));
#159672=CARTESIAN_POINT('Ctrl Pts',(17.7875678303251,5.13687695182573,151.411128767089));
#159673=CARTESIAN_POINT('Ctrl Pts',(17.7873134815034,5.13696350910884,151.411173789116));
#159674=CARTESIAN_POINT('Ctrl Pts',(17.787059085774,5.13705008099148,151.411218752855));
#159675=CARTESIAN_POINT('Ctrl Pts',(17.786804643145,5.13713666747989,151.411263658254));
#159676=CARTESIAN_POINT('Origin',(18.3860172570956,4.6108717272504,149.809053790145));
#159677=CARTESIAN_POINT('Origin',(17.5670013193858,-20.2701550170912,149.926880696201));
#159678=CARTESIAN_POINT('',(17.7869656855113,5.48598638025556,151.411234961359));
#159679=CARTESIAN_POINT('Ctrl Pts',(17.7868045798642,5.13713666751144,151.411263299869));
#159680=CARTESIAN_POINT('Ctrl Pts',(17.7866214367151,5.25353464188215,151.411295592951));
#159681=CARTESIAN_POINT('Ctrl Pts',(17.7871314417319,5.36958837810028,151.411205734173));
#159682=CARTESIAN_POINT('Ctrl Pts',(17.7869656855113,5.48598638025556,151.411234961359));
#159683=CARTESIAN_POINT('',(19.0080066341158,5.48838252639704,149.699374882563));
#159684=CARTESIAN_POINT('Origin',(17.5264760320735,5.48598635204796,149.934026397755));
#159685=CARTESIAN_POINT('',(19.0093911642939,4.61188418703121,149.69916599175));
#159686=CARTESIAN_POINT('Origin',(20.3497043807186,5.49056659368763,149.436215067118));
#159687=CARTESIAN_POINT('Origin',(20.3542501960586,5.49056659368762,149.461995667018));
#159688=CARTESIAN_POINT('Origin',(20.6101766471986,5.4905665936876,150.913426696618));
#159689=CARTESIAN_POINT('Origin',(18.5286714535786,5.49056659368762,139.108624134518));
#159690=CARTESIAN_POINT('',(15.7182861536206,5.48896890084689,128.928900209889));
#159691=CARTESIAN_POINT('Origin',(16.7030926497186,5.49056659368762,128.755252253918));
#159692=CARTESIAN_POINT('',(15.7182861536206,5.48896890084689,128.928900209889));
#159693=CARTESIAN_POINT('Origin',(15.7182861536206,5.48896890084689,128.928900209889));
#159694=CARTESIAN_POINT('',(15.7196652540208,4.61247156689892,128.928657037242));
#159695=CARTESIAN_POINT('',(19.0093911642939,4.61188418703121,149.69916599175));
#159696=CARTESIAN_POINT('',(15.7182861536206,5.48896890084689,128.928900209889));
#159697=CARTESIAN_POINT('Origin',(16.5604381014256,4.61087172725039,139.455679914345));
#159698=CARTESIAN_POINT('Origin',(14.9224228568571,4.6108991365907,130.067238728311));
#159699=CARTESIAN_POINT('Origin',(12.3566858837803,14.4973641791059,133.712013119689));
#159700=CARTESIAN_POINT('',(15.7196652540158,4.61247156689931,128.92865703727));
#159701=CARTESIAN_POINT('Origin',(1.84116836823847,-0.0335515531888081,
131.375810489939));
#159702=CARTESIAN_POINT('',(26.5526523577434,4.55654473273787,127.018509129283));
#159703=CARTESIAN_POINT('',(26.5669704824415,-4.54344365282274,127.015984457585));
#159704=CARTESIAN_POINT('',(26.5526523577434,4.55654473273787,127.018509129283));
#159705=CARTESIAN_POINT('',(17.5909132444034,4.54200572788895,128.598705529056));
#159706=CARTESIAN_POINT('',(17.5909132444034,4.54200572788895,128.598705529056));
#159707=CARTESIAN_POINT('',(17.5929586907863,3.24200738870957,128.598344861672));
#159708=CARTESIAN_POINT('',(17.5929586907863,3.24200738870957,128.598344861672));
#159709=CARTESIAN_POINT('',(17.1005554416673,3.24120854228747,128.685168839857));
#159710=CARTESIAN_POINT('',(17.1005554416673,3.24120854228747,128.685168839857));
#159711=CARTESIAN_POINT('',(17.1107826735945,-3.2587831616844,128.68336550293));
#159712=CARTESIAN_POINT('',(17.1107826735945,-3.2587831616844,128.68336550293));
#159713=CARTESIAN_POINT('',(17.6031859216335,-3.25798431526405,128.596541524945));
#159714=CARTESIAN_POINT('',(17.6031859216335,-3.25798431526405,128.596541524945));
#159715=CARTESIAN_POINT('',(17.6052313680214,-4.55798265767342,128.596180857559));
#159716=CARTESIAN_POINT('',(17.6052313680214,-4.55798265767342,128.596180857559));
#159717=CARTESIAN_POINT('',(26.5669704824415,-4.54344365282274,127.015984457585));
#159718=CARTESIAN_POINT('Origin',(26.5669704824415,-4.54344365282274,127.015984457585));
#159719=CARTESIAN_POINT('',(30.4597363552535,4.55654473273787,149.176683572083));
#159720=CARTESIAN_POINT('',(26.5526523577434,4.55654473273787,127.018509129283));
#159721=CARTESIAN_POINT('',(30.4740544799515,-4.54344365282274,149.174158900385));
#159722=CARTESIAN_POINT('',(26.5669704824415,-4.54344365282274,127.015984457585));
#159723=CARTESIAN_POINT('',(30.4740544799515,-4.54344365282274,149.174158900385));
#159724=CARTESIAN_POINT('Origin',(26.5526523577434,4.55654473273787,127.018509129283));
#159725=CARTESIAN_POINT('',(21.4979972419134,4.54200572788897,150.756879971756));
#159726=CARTESIAN_POINT('',(17.5909132444034,4.54200572788895,128.598705529056));
#159727=CARTESIAN_POINT('',(30.4597363552535,4.55654473273787,149.176683572083));
#159728=CARTESIAN_POINT('Origin',(17.5909132444034,4.54200572788895,128.598705529056));
#159729=CARTESIAN_POINT('',(21.5000426882963,3.2420073887096,150.756519304372));
#159730=CARTESIAN_POINT('',(17.5929586907863,3.24200738870957,128.598344861672));
#159731=CARTESIAN_POINT('',(21.4979972419134,4.54200572788897,150.756879971756));
#159732=CARTESIAN_POINT('Origin',(17.5929586907863,3.24200738870957,128.598344861672));
#159733=CARTESIAN_POINT('',(21.0076394391673,3.24120854228745,150.843343282657));
#159734=CARTESIAN_POINT('',(17.1005554416673,3.24120854228747,128.685168839857));
#159735=CARTESIAN_POINT('',(21.5000426882963,3.2420073887096,150.756519304372));
#159736=CARTESIAN_POINT('Origin',(17.1005554416673,3.24120854228747,128.685168839857));
#159737=CARTESIAN_POINT('',(21.0178666710944,-3.25878316168441,150.84153994573));
#159738=CARTESIAN_POINT('',(17.1107826735945,-3.2587831616844,128.68336550293));
#159739=CARTESIAN_POINT('',(21.0076394391673,3.24120854228745,150.843343282657));
#159740=CARTESIAN_POINT('Origin',(17.1107826735945,-3.2587831616844,128.68336550293));
#159741=CARTESIAN_POINT('',(21.5102699191435,-3.25798431526402,150.754715967645));
#159742=CARTESIAN_POINT('',(17.6031859216335,-3.25798431526405,128.596541524945));
#159743=CARTESIAN_POINT('',(21.0178666710944,-3.25878316168441,150.84153994573));
#159744=CARTESIAN_POINT('Origin',(17.6031859216335,-3.25798431526405,128.596541524945));
#159745=CARTESIAN_POINT('',(21.5123153655314,-4.55798265767339,150.754355300259));
#159746=CARTESIAN_POINT('',(17.6052313680214,-4.55798265767342,128.596180857559));
#159747=CARTESIAN_POINT('',(21.5102699191435,-3.25798431526402,150.754715967645));
#159748=CARTESIAN_POINT('Origin',(17.6052313680214,-4.55798265767342,128.596180857559));
#159749=CARTESIAN_POINT('',(21.5123153655314,-4.55798265767339,150.754355300259));
#159750=CARTESIAN_POINT('Origin',(26.4291887836315,-2.1219048984176E-14,
149.887377855954));
#159751=CARTESIAN_POINT('Origin',(26.4291887836315,-2.1219048984176E-14,
149.887377855954));
#159752=CARTESIAN_POINT('Origin',(-6.15924143489591,24.952514954652,136.340491736592));
#159753=CARTESIAN_POINT('',(21.0787428031861,-20.7493757828675,119.352580872645));
#159754=CARTESIAN_POINT('',(21.012266743147,21.4999725592939,119.364302395635));
#159755=CARTESIAN_POINT('Origin',(21.0460952759615,-9.02974887056722E-15,
119.358337512554));
#159756=CARTESIAN_POINT('Ctrl Pts',(94.4677262089947,4.26458625199329,142.134302812303));
#159757=CARTESIAN_POINT('Ctrl Pts',(94.325324460867,3.88264561414907,142.026683431587));
#159758=CARTESIAN_POINT('Ctrl Pts',(94.0716376882548,3.10957209929612,141.841360490054));
#159759=CARTESIAN_POINT('Ctrl Pts',(93.810153878733,1.9414001629906,141.658481685112));
#159760=CARTESIAN_POINT('Ctrl Pts',(93.6806979553918,0.830568367124271,
141.569555741515));
#159761=CARTESIAN_POINT('Ctrl Pts',(93.6640015230007,-0.217429764701261,
141.556979537194));
#159762=CARTESIAN_POINT('Ctrl Pts',(93.7471059523909,-1.24660990130415,
141.611474474069));
#159763=CARTESIAN_POINT('Ctrl Pts',(93.9298885891748,-2.27247910489614,
141.735159766024));
#159764=CARTESIAN_POINT('Ctrl Pts',(94.1843275940772,-3.21196450833431,
141.913619082162));
#159765=CARTESIAN_POINT('Ctrl Pts',(94.384865518228,-3.79126873095784,142.060241775828));
#159766=CARTESIAN_POINT('Ctrl Pts',(94.4808018463151,-4.04615891951393,
142.131996757721));
#159767=CARTESIAN_POINT('Ctrl Pts',(94.8031311051781,4.17070113450257,142.052929078712));
#159768=CARTESIAN_POINT('Ctrl Pts',(94.6623836287724,3.79574718487004,141.944065691349));
#159769=CARTESIAN_POINT('Ctrl Pts',(94.4120362510534,3.03789023725012,141.756839725743));
#159770=CARTESIAN_POINT('Ctrl Pts',(94.1547643263253,1.89611374480954,141.572553509887));
#159771=CARTESIAN_POINT('Ctrl Pts',(94.0276583019129,0.812719749478585,
141.483112913603));
#159772=CARTESIAN_POINT('Ctrl Pts',(94.0112683209779,-0.208537697884529,
141.470480186353));
#159773=CARTESIAN_POINT('Ctrl Pts',(94.0928124726429,-1.21183598557444,
141.525284855749));
#159774=CARTESIAN_POINT('Ctrl Pts',(94.2724474101964,-2.2134236624816,141.649827072304));
#159775=CARTESIAN_POINT('Ctrl Pts',(94.5230912346179,-3.13277799467634,
141.829876753025));
#159776=CARTESIAN_POINT('Ctrl Pts',(94.7210926373913,-3.70094603761282,
141.978086379388));
#159777=CARTESIAN_POINT('Ctrl Pts',(94.815909527443,-3.95117347469028,142.050675379175));
#159778=CARTESIAN_POINT('Ctrl Pts',(95.1198224210223,4.03339275365646,142.146660496547));
#159779=CARTESIAN_POINT('Ctrl Pts',(94.9835402883144,3.66863510173414,142.037649619029));
#159780=CARTESIAN_POINT('Ctrl Pts',(94.7416652223918,2.93298390507885,141.850476134561));
#159781=CARTESIAN_POINT('Ctrl Pts',(94.4941624531867,1.82972313738508,141.666861333164));
#159782=CARTESIAN_POINT('Ctrl Pts',(94.3722609744833,0.786363145160593,
141.577972687657));
#159783=CARTESIAN_POINT('Ctrl Pts',(94.3565650060748,-0.195879481250129,
141.565437151993));
#159784=CARTESIAN_POINT('Ctrl Pts',(94.4347331412821,-1.16141782934051,
141.619890673295));
#159785=CARTESIAN_POINT('Ctrl Pts',(94.6073024106271,-2.12758230072278,
141.743846418259));
#159786=CARTESIAN_POINT('Ctrl Pts',(94.8488894983716,-3.01757032297491,
141.923521976027));
#159787=CARTESIAN_POINT('Ctrl Pts',(95.0403543380529,-3.56949458930854,
142.071791382735));
#159788=CARTESIAN_POINT('Ctrl Pts',(95.1321672209127,-3.81292095042804,
142.144483189647));
#159789=CARTESIAN_POINT('Ctrl Pts',(95.3363636309633,3.88796967926968,142.391394222942));
#159790=CARTESIAN_POINT('Ctrl Pts',(95.2062096599398,3.53399597741717,142.283370298785));
#159791=CARTESIAN_POINT('Ctrl Pts',(94.9757611852104,2.82182955193183,142.098191305131));
#159792=CARTESIAN_POINT('Ctrl Pts',(94.7410727240179,1.75930054987824,141.917154090713));
#159793=CARTESIAN_POINT('Ctrl Pts',(94.6258920995078,0.758276101163494,
141.829742066319));
#159794=CARTESIAN_POINT('Ctrl Pts',(94.6110992405489,-0.182710149363758,
141.817432444289));
#159795=CARTESIAN_POINT('Ctrl Pts',(94.6849437563614,-1.1083203585478,141.87096423382));
#159796=CARTESIAN_POINT('Ctrl Pts',(94.848346310829,-2.03702895054977,141.993040920939));
#159797=CARTESIAN_POINT('Ctrl Pts',(95.077944026924,-2.89596691080905,142.170474073356));
#159798=CARTESIAN_POINT('Ctrl Pts',(95.2605531255443,-3.43071685761424,
142.317260735522));
#159799=CARTESIAN_POINT('Ctrl Pts',(95.3482499064457,-3.66695270109413,
142.389297701919));
#159800=CARTESIAN_POINT('',(95.2116320414304,3.87890261200112,142.275538234229));
#159801=CARTESIAN_POINT('Origin',(94.5824319951644,3.87766013850041,143.052704236177));
#159802=CARTESIAN_POINT('',(95.223491004657,-3.65821211009624,142.273447286233));
#159803=CARTESIAN_POINT('Ctrl Pts',(95.2116318269622,3.87890261158699,142.275538499172));
#159804=CARTESIAN_POINT('Ctrl Pts',(95.0892916816967,3.54282600750017,142.175974488895));
#159805=CARTESIAN_POINT('Ctrl Pts',(94.8641911706135,2.84386470343991,141.998174645644));
#159806=CARTESIAN_POINT('Ctrl Pts',(94.629784427461,1.78908951785421,141.820372677863));
#159807=CARTESIAN_POINT('Ctrl Pts',(94.5118334959788,0.770149152459641,
141.732389968258));
#159808=CARTESIAN_POINT('Ctrl Pts',(94.496668722276,-0.188296407942078,
141.719992216783));
#159809=CARTESIAN_POINT('Ctrl Pts',(94.5722972036391,-1.1308039059681,141.773880662021));
#159810=CARTESIAN_POINT('Ctrl Pts',(94.7394761249336,-2.07536362700424,
141.896676127896));
#159811=CARTESIAN_POINT('Ctrl Pts',(94.9673857696971,-2.92284253173479,
142.069917541593));
#159812=CARTESIAN_POINT('Ctrl Pts',(95.14392684748,-3.4417481453771,142.20937126949));
#159813=CARTESIAN_POINT('Ctrl Pts',(95.2234908094786,-3.65821211046655,
142.27344752735));
#159814=CARTESIAN_POINT('Origin',(94.5942416492558,-3.65942148632551,143.05082648727));
#159815=CARTESIAN_POINT('Ctrl Pts',(100.709300696936,5.04237442459277,150.282068014958));
#159816=CARTESIAN_POINT('Ctrl Pts',(100.727900795881,-6.7790538657833,150.27878831567));
#159817=CARTESIAN_POINT('Ctrl Pts',(99.5012583427497,5.04146860010937,146.69589528654));
#159818=CARTESIAN_POINT('Ctrl Pts',(99.5198584416948,-6.7799596902667,146.692615587252));
#159819=CARTESIAN_POINT('Ctrl Pts',(97.4016151358028,5.03896189264658,143.82346459845));
#159820=CARTESIAN_POINT('Ctrl Pts',(97.4202152347478,-6.78246639772949,
143.820184899162));
#159821=CARTESIAN_POINT('Ctrl Pts',(94.4103710760951,5.03485430220433,141.664775950885));
#159822=CARTESIAN_POINT('Ctrl Pts',(94.4289711750401,-6.78657398817173,
141.661496251597));
#159823=CARTESIAN_POINT('',(97.16866993185,-4.72410467554793,144.11266556739));
#159824=CARTESIAN_POINT('Ctrl Pts',(95.2234913950221,-3.65821210935081,
142.273446804006));
#159825=CARTESIAN_POINT('Ctrl Pts',(95.2467072678134,-3.72130470321278,
142.292142621898));
#159826=CARTESIAN_POINT('Ctrl Pts',(95.2748644610139,-3.78234564067068,
142.314939154039));
#159827=CARTESIAN_POINT('Ctrl Pts',(95.3069266235745,-3.84060070705387,
142.341129033054));
#159828=CARTESIAN_POINT('Ctrl Pts',(95.3630114364024,-3.94250351813844,
142.386941740159));
#159829=CARTESIAN_POINT('Ctrl Pts',(95.4310450012107,-4.03588190091921,
142.443137694358));
#159830=CARTESIAN_POINT('Ctrl Pts',(95.5063030800419,-4.12035383948242,
142.506553038376));
#159831=CARTESIAN_POINT('Ctrl Pts',(95.5905482312874,-4.21491313930498,
142.577541234342));
#159832=CARTESIAN_POINT('Ctrl Pts',(95.6838463850794,-4.29831182574749,
142.657576009313));
#159833=CARTESIAN_POINT('Ctrl Pts',(95.7819301502628,-4.37102508631497,
142.743838974376));
#159834=CARTESIAN_POINT('Ctrl Pts',(95.8913775114615,-4.45216261685718,
142.840096024437));
#159835=CARTESIAN_POINT('Ctrl Pts',(96.0067836061993,-4.51999534577716,
142.944108012202));
#159836=CARTESIAN_POINT('Ctrl Pts',(96.1245864449981,-4.57509531248624,
143.053498457647));
#159837=CARTESIAN_POINT('Ctrl Pts',(96.252371147288,-4.634864100012,143.172157953862));
#159838=CARTESIAN_POINT('Ctrl Pts',(96.3829759713566,-4.67965091346211,
143.2971459968));
#159839=CARTESIAN_POINT('Ctrl Pts',(96.513330033225,-4.70934161504182,143.42615701659));
#159840=CARTESIAN_POINT('Ctrl Pts',(96.6470643254029,-4.73980223056167,
143.558513440069));
#159841=CARTESIAN_POINT('Ctrl Pts',(96.7805346806551,-4.75437365891532,
143.695104185896));
#159842=CARTESIAN_POINT('Ctrl Pts',(96.9110983918428,-4.75202486117502,
143.833436285795));
#159843=CARTESIAN_POINT('Ctrl Pts',(96.9985940960846,-4.75045084255575,
143.926137882508));
#159844=CARTESIAN_POINT('Ctrl Pts',(97.0847844692051,-4.74127820475585,
144.019621493763));
#159845=CARTESIAN_POINT('Ctrl Pts',(97.168671748338,-4.72410467227896,144.112663929037));
#159846=CARTESIAN_POINT('',(97.153448356702,4.94989036380522,144.115349759976));
#159847=CARTESIAN_POINT('Ctrl Pts',(97.1534510310516,4.94989036871313,144.115347348054));
#159848=CARTESIAN_POINT('Ctrl Pts',(97.0659102985489,4.96757874934412,144.018325642839));
#159849=CARTESIAN_POINT('Ctrl Pts',(96.9758866343682,4.97655737323447,143.920815999854));
#159850=CARTESIAN_POINT('Ctrl Pts',(96.8845082164897,4.9772843793877,143.824195088114));
#159851=CARTESIAN_POINT('Ctrl Pts',(96.753482688462,4.97832681771523,143.685652462043));
#159852=CARTESIAN_POINT('Ctrl Pts',(96.6196717801744,4.96240387464917,143.548937076949));
#159853=CARTESIAN_POINT('Ctrl Pts',(96.4857353063917,4.93053759771028,143.416539758115));
#159854=CARTESIAN_POINT('Ctrl Pts',(96.3555356989818,4.89956039911845,143.287836362785));
#159855=CARTESIAN_POINT('Ctrl Pts',(96.2252174360236,4.85351710908179,143.163213444886));
#159856=CARTESIAN_POINT('Ctrl Pts',(96.09787659053,4.79250224244665,143.044982433951));
#159857=CARTESIAN_POINT('Ctrl Pts',(95.9807258681,4.73636993330757,142.936212555041));
#159858=CARTESIAN_POINT('Ctrl Pts',(95.8660951089851,4.66756630602553,142.83285252219));
#159859=CARTESIAN_POINT('Ctrl Pts',(95.7575771952769,4.58551682113803,142.737294315022));
#159860=CARTESIAN_POINT('Ctrl Pts',(95.6604238270679,4.51205997383748,142.65174344725));
#159861=CARTESIAN_POINT('Ctrl Pts',(95.5681700069202,4.42798635034682,142.572445874935));
#159862=CARTESIAN_POINT('Ctrl Pts',(95.4851091592593,4.33284712380514,142.502236728833));
#159863=CARTESIAN_POINT('Ctrl Pts',(95.4108924557532,4.24783812176753,142.439503304766));
#159864=CARTESIAN_POINT('Ctrl Pts',(95.3440152452747,4.15399454704945,142.384025908196));
#159865=CARTESIAN_POINT('Ctrl Pts',(95.289209369605,4.0517725391194,142.338977034317));
#159866=CARTESIAN_POINT('Ctrl Pts',(95.259519461425,3.99639595782553,142.314572772681));
#159867=CARTESIAN_POINT('Ctrl Pts',(95.2333721263064,3.9385605546291,142.293228968045));
#159868=CARTESIAN_POINT('Ctrl Pts',(95.2116324703669,3.87890261282936,142.275537704344));
#159869=CARTESIAN_POINT('',(100.3971489688,2.11466427441707,149.409381531096));
#159870=CARTESIAN_POINT('Ctrl Pts',(100.397149868591,2.11466427596188,149.409381179598));
#159871=CARTESIAN_POINT('Ctrl Pts',(100.264072070223,2.4743631149336,149.070307282051));
#159872=CARTESIAN_POINT('Ctrl Pts',(99.9316309122332,3.18218183511712,148.28374709774));
#159873=CARTESIAN_POINT('Ctrl Pts',(99.2367363880305,4.03704249542641,146.932753463133));
#159874=CARTESIAN_POINT('Ctrl Pts',(98.3041095906132,4.63847370651756,145.487158534252));
#159875=CARTESIAN_POINT('Ctrl Pts',(97.5462262568398,4.87042480372463,144.550915761011));
#159876=CARTESIAN_POINT('Ctrl Pts',(97.1534470196683,4.94989036130278,144.115350966093));
#159877=CARTESIAN_POINT('',(100.403437304611,-1.88162507939484,149.408270627991));
#159878=CARTESIAN_POINT('Ctrl Pts',(100.403437652402,-1.88162317480153,
149.408272487378));
#159879=CARTESIAN_POINT('Ctrl Pts',(100.451208759698,-1.75118679936034,
149.531126155632));
#159880=CARTESIAN_POINT('Ctrl Pts',(100.545485504079,-1.43297394048954,
149.782281369385));
#159881=CARTESIAN_POINT('Ctrl Pts',(100.644986088431,-0.868477907273701,
150.064530940924));
#159882=CARTESIAN_POINT('Ctrl Pts',(100.69686050395,-0.212788963995321,
150.219404994051));
#159883=CARTESIAN_POINT('Ctrl Pts',(100.695307264391,0.458828142569949,
150.218119833334));
#159884=CARTESIAN_POINT('Ctrl Pts',(100.640359242456,1.11382689997406,150.060732638077));
#159885=CARTESIAN_POINT('Ctrl Pts',(100.538802206203,1.67318407177052,149.778262943369));
#159886=CARTESIAN_POINT('Ctrl Pts',(100.444203553735,1.98735761693585,149.529289759105));
#159887=CARTESIAN_POINT('Ctrl Pts',(100.397149868591,2.11466427596188,149.409381179598));
#159888=CARTESIAN_POINT('Ctrl Pts',(97.168669023838,-4.72410467713493,144.112666386824));
#159889=CARTESIAN_POINT('Ctrl Pts',(97.5655380434849,-4.64275293009404,
144.553083450934));
#159890=CARTESIAN_POINT('Ctrl Pts',(98.3258634243098,-4.40699925250942,
145.494588767759));
#159891=CARTESIAN_POINT('Ctrl Pts',(99.2574692905987,-3.79861237595365,
146.945295844755));
#159892=CARTESIAN_POINT('Ctrl Pts',(99.9451052029796,-2.94278987349825,
148.290837223702));
#159893=CARTESIAN_POINT('Ctrl Pts',(100.272985516958,-2.23746403900694,
149.072839132248));
#159894=CARTESIAN_POINT('Ctrl Pts',(100.403436966518,-1.8816250457219,149.408270723756));
#159895=CARTESIAN_POINT('Ctrl Pts',(93.6948982478023,-3.9130261905305,142.678416629155));
#159896=CARTESIAN_POINT('Ctrl Pts',(93.743554307992,-4.08317118406646,142.715180369127));
#159897=CARTESIAN_POINT('Ctrl Pts',(93.890833594482,-4.43602161921736,142.827213486021));
#159898=CARTESIAN_POINT('Ctrl Pts',(94.197684598825,-4.87048287682669,143.067043278988));
#159899=CARTESIAN_POINT('Ctrl Pts',(94.5858697526221,-5.23220927751511,
143.384411304587));
#159900=CARTESIAN_POINT('Ctrl Pts',(95.0284082738768,-5.50573316404525,
143.76865508919));
#159901=CARTESIAN_POINT('Ctrl Pts',(95.5061222115966,-5.6797337413587,144.215123578903));
#159902=CARTESIAN_POINT('Ctrl Pts',(95.9650706075177,-5.73397405955418,
144.681053992722));
#159903=CARTESIAN_POINT('Ctrl Pts',(96.2562974300626,-5.69489479826764,
145.001037870784));
#159904=CARTESIAN_POINT('Ctrl Pts',(96.3841297881998,-5.66022393088418,
145.146508645044));
#159905=CARTESIAN_POINT('Ctrl Pts',(94.0201637971862,-3.98769337013459,
141.94166108681));
#159906=CARTESIAN_POINT('Ctrl Pts',(94.0755116171319,-4.17658156420627,
141.983279312062));
#159907=CARTESIAN_POINT('Ctrl Pts',(94.2425795356422,-4.56610838669949,
142.109730188625));
#159908=CARTESIAN_POINT('Ctrl Pts',(94.5866480995851,-5.03825401711204,
142.377170408612));
#159909=CARTESIAN_POINT('Ctrl Pts',(95.0169249190105,-5.42560988395097,
142.727049095028));
#159910=CARTESIAN_POINT('Ctrl Pts',(95.5036527056414,-5.71562220389437,
143.147755229396));
#159911=CARTESIAN_POINT('Ctrl Pts',(96.0270857752493,-5.89931148731261,
143.635508492719));
#159912=CARTESIAN_POINT('Ctrl Pts',(96.5298127726263,-5.9566654395584,144.145373780338));
#159913=CARTESIAN_POINT('Ctrl Pts',(96.8495393014006,-5.91530475223614,
144.497000776349));
#159914=CARTESIAN_POINT('Ctrl Pts',(96.990121998386,-5.87841909048293,144.65727863506));
#159915=CARTESIAN_POINT('Ctrl Pts',(94.792363611226,-3.80564312789954,141.784343691287));
#159916=CARTESIAN_POINT('Ctrl Pts',(94.8353416091631,-3.94957461808571,
141.817287026332));
#159917=CARTESIAN_POINT('Ctrl Pts',(94.9665075650647,-4.25112502864957,
141.918519941624));
#159918=CARTESIAN_POINT('Ctrl Pts',(95.2489514150549,-4.6328552561169,142.142626516623));
#159919=CARTESIAN_POINT('Ctrl Pts',(95.6179342728045,-4.9586911421452,142.448605660312));
#159920=CARTESIAN_POINT('Ctrl Pts',(96.0479270829259,-5.20909416509736,
142.826287646371));
#159921=CARTESIAN_POINT('Ctrl Pts',(96.5175822681404,-5.36947399865914,
143.26851859957));
#159922=CARTESIAN_POINT('Ctrl Pts',(96.9700113870813,-5.41929000533494,
143.728991628168));
#159923=CARTESIAN_POINT('Ctrl Pts',(97.2558433417816,-5.38335705658195,
144.042280799348));
#159924=CARTESIAN_POINT('Ctrl Pts',(97.3808064392917,-5.35176423600097,
144.18379587502));
#159925=CARTESIAN_POINT('Ctrl Pts',(95.3016037801828,-3.53423675537427,
142.351088487871));
#159926=CARTESIAN_POINT('Ctrl Pts',(95.3245221219672,-3.61084095345401,
142.369802503292));
#159927=CARTESIAN_POINT('Ctrl Pts',(95.3971006883962,-3.78064007830534,
142.429364954977));
#159928=CARTESIAN_POINT('Ctrl Pts',(95.5757299983015,-4.0269752505514,142.579031028893));
#159929=CARTESIAN_POINT('Ctrl Pts',(95.8363816489282,-4.26069787329206,
142.805057879427));
#159930=CARTESIAN_POINT('Ctrl Pts',(96.1608724850215,-4.45180724034671,
143.099781910541));
#159931=CARTESIAN_POINT('Ctrl Pts',(96.5266915181716,-4.57730816593525,
143.451532755502));
#159932=CARTESIAN_POINT('Ctrl Pts',(96.8809858101989,-4.61586438445729,
143.814693375449));
#159933=CARTESIAN_POINT('Ctrl Pts',(97.1016886587558,-4.58807854415974,
144.054908268628));
#159934=CARTESIAN_POINT('Ctrl Pts',(97.1970215311566,-4.56442041860899,
144.161339578343));
#159935=CARTESIAN_POINT('',(96.4276511501619,-5.70697315835852,144.973748692482));
#159936=CARTESIAN_POINT('Origin',(96.4260783789126,-4.72539616721717,144.782471517403));
#159937=CARTESIAN_POINT('Ctrl Pts',(94.5946916752436,-3.92833378532365,
142.087508698775));
#159938=CARTESIAN_POINT('Ctrl Pts',(94.6072841821975,-3.98846146113012,
142.104301905679));
#159939=CARTESIAN_POINT('Ctrl Pts',(94.6220231953396,-4.04932725666999,
142.123731558378));
#159940=CARTESIAN_POINT('Ctrl Pts',(94.6389082768763,-4.11065296415126,
142.146050941591));
#159941=CARTESIAN_POINT('Ctrl Pts',(94.6555164167165,-4.17097283429421,
142.168004252077));
#159942=CARTESIAN_POINT('Ctrl Pts',(94.674200804506,-4.2317376421803,142.192753727171));
#159943=CARTESIAN_POINT('Ctrl Pts',(94.6949609514218,-4.29263674381567,
142.220522459942));
#159944=CARTESIAN_POINT('Ctrl Pts',(94.715381301438,-4.35253906416544,142.247836681031));
#159945=CARTESIAN_POINT('Ctrl Pts',(94.7378100155495,-4.41257124202651,
142.278072578247));
#159946=CARTESIAN_POINT('Ctrl Pts',(94.7622465591094,-4.47239350470747,
142.311418386374));
#159947=CARTESIAN_POINT('Ctrl Pts',(94.7866831026693,-4.53221576738843,
142.3447641945));
#159948=CARTESIAN_POINT('Ctrl Pts',(94.8131274756349,-4.59182808787051,
142.381220462011));
#159949=CARTESIAN_POINT('Ctrl Pts',(94.8415790742591,-4.65084677191736,
142.420943627582));
#159950=CARTESIAN_POINT('Ctrl Pts',(94.8687546763644,-4.7072185876321,142.458885289707));
#159951=CARTESIAN_POINT('Ctrl Pts',(94.8977615006632,-4.76304838976179,
142.499807595353));
#159952=CARTESIAN_POINT('Ctrl Pts',(94.928598963509,-4.81796525172841,142.54381256834));
#159953=CARTESIAN_POINT('Ctrl Pts',(94.9589917576618,-4.87209022593974,
142.587183000349));
#159954=CARTESIAN_POINT('Ctrl Pts',(94.9911627759117,-4.92532816324288,
142.63354821058));
#159955=CARTESIAN_POINT('Ctrl Pts',(95.0251114089696,-4.97729183372492,
142.68296713936));
#159956=CARTESIAN_POINT('Ctrl Pts',(95.058395671812,-5.02823858211499,142.731418946304));
#159957=CARTESIAN_POINT('Ctrl Pts',(95.0933886544008,-5.07796014305279,
142.78280641666));
#159958=CARTESIAN_POINT('Ctrl Pts',(95.1300897399471,-5.12606451376125,
142.837142732317));
#159959=CARTESIAN_POINT('Ctrl Pts',(95.1387658922046,-5.13743640748879,
142.849987860485));
#159960=CARTESIAN_POINT('Ctrl Pts',(95.1475375018997,-5.14871781501934,
142.862997584704));
#159961=CARTESIAN_POINT('Ctrl Pts',(95.156404560575,-5.15990336111806,142.876171695935));
#159962=CARTESIAN_POINT('Ctrl Pts',(95.1769795765034,-5.18585816728068,
142.906740744631));
#159963=CARTESIAN_POINT('Ctrl Pts',(95.1980685090438,-5.21129696288514,
142.938195204438));
#159964=CARTESIAN_POINT('Ctrl Pts',(95.2196712502921,-5.23615116776965,
142.970529156747));
#159965=CARTESIAN_POINT('Ctrl Pts',(95.2304726209163,-5.24857827021191,
142.986696132901));
#159966=CARTESIAN_POINT('Ctrl Pts',(95.2414024437426,-5.26085924098744,
143.003082970078));
#159967=CARTESIAN_POINT('Ctrl Pts',(95.2524607049315,-5.27298528412071,
143.019688407892));
#159968=CARTESIAN_POINT('Ctrl Pts',(95.257989835526,-5.27904830568736,143.027991126799));
#159969=CARTESIAN_POINT('Ctrl Pts',(95.2635510757132,-5.28507259667165,
143.036348494827));
#159970=CARTESIAN_POINT('Ctrl Pts',(95.2691444237609,-5.29105705605127,
143.044760335691));
#159971=CARTESIAN_POINT('Ctrl Pts',(95.2719410977847,-5.29404928574108,
143.048966256123));
#159972=CARTESIAN_POINT('Ctrl Pts',(95.2747457987738,-5.29703155760949,
143.053185794708));
#159973=CARTESIAN_POINT('Ctrl Pts',(95.2775585265105,-5.30000373341748,
143.057418927516));
#159974=CARTESIAN_POINT('Ctrl Pts',(95.2789648903789,-5.30148982132147,
143.05953549392));
#159975=CARTESIAN_POINT('Ctrl Pts',(95.2803732609343,-5.30297338521556,
143.061655458876));
#159976=CARTESIAN_POINT('Ctrl Pts',(95.2817836381493,-5.30445440777924,
143.063778819269));
#159977=CARTESIAN_POINT('Ctrl Pts',(95.2831940153643,-5.30593543034291,
143.065902179662));
#159978=CARTESIAN_POINT('Ctrl Pts',(95.2852296355216,-5.30806426132359,
143.068967562828));
#159979=CARTESIAN_POINT('Ctrl Pts',(95.2860207897461,-5.30888983415799,
143.070159083596));
#159980=CARTESIAN_POINT('Ctrl Pts',(95.29977098247,-5.32323821937621,143.090867612585));
#159981=CARTESIAN_POINT('Ctrl Pts',(95.3151341469759,-5.33876599641073,
143.113940975202));
#159982=CARTESIAN_POINT('Ctrl Pts',(95.3321099272088,-5.35524689040698,
143.139511997507));
#159983=CARTESIAN_POINT('Ctrl Pts',(95.3489094742827,-5.37155668887929,
143.164817555605));
#159984=CARTESIAN_POINT('Ctrl Pts',(95.3672883285572,-5.38880007239327,
143.192569727119));
#159985=CARTESIAN_POINT('Ctrl Pts',(95.3872460659309,-5.40670751916013,
143.222905563591));
#159986=CARTESIAN_POINT('Ctrl Pts',(95.4067573385441,-5.42421436721271,
143.252562771935));
#159987=CARTESIAN_POINT('Ctrl Pts',(95.4277776435826,-5.44235591927885,
143.284689928006));
#159988=CARTESIAN_POINT('Ctrl Pts',(95.4503065070759,-5.46083095757515,
143.319414767716));
#159989=CARTESIAN_POINT('Ctrl Pts',(95.4724724642041,-5.47900839057976,
143.353580242087));
#159990=CARTESIAN_POINT('Ctrl Pts',(95.4960987700176,-5.49750867406295,
143.390260996447));
#159991=CARTESIAN_POINT('Ctrl Pts',(95.5211848963973,-5.51599617363321,
143.429569587366));
#159992=CARTESIAN_POINT('Ctrl Pts',(95.5455569630813,-5.53395743897682,
143.467759285713));
#159993=CARTESIAN_POINT('Ctrl Pts',(95.5713069272671,-5.55190649923997,
143.508429917924));
#159994=CARTESIAN_POINT('Ctrl Pts',(95.5984342332853,-5.56949020663385,
143.551667475252));
#159995=CARTESIAN_POINT('Ctrl Pts',(95.6186688954836,-5.58260615626295,
143.583919014208));
#159996=CARTESIAN_POINT('Ctrl Pts',(95.6396698941508,-5.59551789842759,
143.617598482181));
#159997=CARTESIAN_POINT('Ctrl Pts',(95.661436972806,-5.60806242852013,143.652732066203));
#159998=CARTESIAN_POINT('Ctrl Pts',(95.6904862361588,-5.62480373607302,
143.699619604533));
#159999=CARTESIAN_POINT('Ctrl Pts',(95.7208999093872,-5.64089259177349,
143.749098762162));
#160000=CARTESIAN_POINT('Ctrl Pts',(95.7526773221263,-5.65590294464707,
143.801200738942));
#160001=CARTESIAN_POINT('Ctrl Pts',(95.7685660284959,-5.66340812108386,
143.827251727332));
#160002=CARTESIAN_POINT('Ctrl Pts',(95.7847956686639,-5.67064298583235,
143.853957809213));
#160003=CARTESIAN_POINT('Ctrl Pts',(95.8013661525195,-5.67755026824592,
143.881318681812));
#160004=CARTESIAN_POINT('Ctrl Pts',(95.8096513944473,-5.6810039094527,143.894999118111));
#160005=CARTESIAN_POINT('Ctrl Pts',(95.8180218472537,-5.68437562754898,
143.908843258848));
#160006=CARTESIAN_POINT('Ctrl Pts',(95.8264774992646,-5.68765800287411,
143.922850681624));
#160007=CARTESIAN_POINT('Ctrl Pts',(95.8320690644977,-5.68982857655982,
143.932113529491));
#160008=CARTESIAN_POINT('Ctrl Pts',(95.8380393093066,-5.69208814865569,
143.942013881579));
#160009=CARTESIAN_POINT('Ctrl Pts',(95.8437108975836,-5.6941782216613,143.951429056206));
#160010=CARTESIAN_POINT('Ctrl Pts',(95.8466159734104,-5.69524878959892,
143.956251655252));
#160011=CARTESIAN_POINT('Ctrl Pts',(95.8494426936656,-5.69627576843121,
143.960946755587));
#160012=CARTESIAN_POINT('Ctrl Pts',(95.8521000410666,-5.69722957306762,
143.965362351826));
#160013=CARTESIAN_POINT('Ctrl Pts',(95.8876723499013,-5.7099975811501,144.024471278662));
#160014=CARTESIAN_POINT('Ctrl Pts',(95.9220548804864,-5.72024626941926,
144.082306677532));
#160015=CARTESIAN_POINT('Ctrl Pts',(95.955248172871,-5.72831884084642,144.138658626608));
#160016=CARTESIAN_POINT('Ctrl Pts',(95.9890946552891,-5.73655026735611,
144.196119490434));
#160017=CARTESIAN_POINT('Ctrl Pts',(96.021704635216,-5.7425195833988,144.252038215401));
#160018=CARTESIAN_POINT('Ctrl Pts',(96.0530786745858,-5.74658390705029,
144.306246926715));
#160019=CARTESIAN_POINT('Ctrl Pts',(96.085399727975,-5.7507709108397,144.362091908355));
#160020=CARTESIAN_POINT('Ctrl Pts',(96.1164091026634,-5.75293667524588,
144.416122349026));
#160021=CARTESIAN_POINT('Ctrl Pts',(96.1461073897856,-5.75345688194664,
144.468208200209));
#160022=CARTESIAN_POINT('Ctrl Pts',(96.1590723910637,-5.75368398193097,
144.490946653925));
#160023=CARTESIAN_POINT('Ctrl Pts',(96.1717875220325,-5.75359723721135,
144.513315153081));
#160024=CARTESIAN_POINT('Ctrl Pts',(96.1842528300077,-5.75322671858692,
144.535305717831));
#160025=CARTESIAN_POINT('Ctrl Pts',(96.2140135587319,-5.75234211113953,
144.58780784881));
#160026=CARTESIAN_POINT('Ctrl Pts',(96.2423502790985,-5.749841982628,144.638152608364));
#160027=CARTESIAN_POINT('Ctrl Pts',(96.2692636041749,-5.74611596217628,
144.686265851186));
#160028=CARTESIAN_POINT('Ctrl Pts',(96.2967084946548,-5.74231634905034,
144.735329379239));
#160029=CARTESIAN_POINT('Ctrl Pts',(96.3226732081329,-5.7372422921589,144.782072904419));
#160030=CARTESIAN_POINT('Ctrl Pts',(96.3471583424773,-5.73127376595626,
144.826461201895));
#160031=CARTESIAN_POINT('Ctrl Pts',(96.3722830473292,-5.72514933726687,
144.872008955781));
#160032=CARTESIAN_POINT('Ctrl Pts',(96.3958498685693,-5.71808342889945,
144.915077380993));
#160033=CARTESIAN_POINT('Ctrl Pts',(96.4178593893165,-5.71044664608885,
144.95566538353));
#160034=CARTESIAN_POINT('Ctrl Pts',(96.4211582959249,-5.70930200356936,
144.961748933978));
#160035=CARTESIAN_POINT('Ctrl Pts',(96.424422216655,-5.70814445968925,144.967776817202));
#160036=CARTESIAN_POINT('Ctrl Pts',(96.4276511533426,-5.70697518124098,
144.973749086811));
#160037=CARTESIAN_POINT('Ctrl Pts',(46.0788495272599,-8.05252143938036,
146.288922141324));
#160038=CARTESIAN_POINT('Ctrl Pts',(45.9880609926109,-8.16322880697465,
145.977772078405));
#160039=CARTESIAN_POINT('Ctrl Pts',(45.7994922443366,-8.35031067032238,
145.232841472766));
#160040=CARTESIAN_POINT('Ctrl Pts',(45.595594892883,-8.37180617735996,144.001345451837));
#160041=CARTESIAN_POINT('Ctrl Pts',(45.5003027990559,-8.05912368336601,
142.714039383314));
#160042=CARTESIAN_POINT('Ctrl Pts',(45.5182680777391,-7.4578196428506,141.583394803538));
#160043=CARTESIAN_POINT('Ctrl Pts',(45.6204150203276,-6.64097899990721,
140.678497336286));
#160044=CARTESIAN_POINT('Ctrl Pts',(45.7705368431435,-5.69964184453771,
140.032177372085));
#160045=CARTESIAN_POINT('Ctrl Pts',(45.9153295749133,-4.84202852027521,
139.689046596473));
#160046=CARTESIAN_POINT('Ctrl Pts',(46.0037739583116,-4.3117657385131,139.572935038824));
#160047=CARTESIAN_POINT('Ctrl Pts',(46.035646729361,-4.11818143590307,139.54229639283));
#160048=CARTESIAN_POINT('Ctrl Pts',(46.3362716867489,-6.53003741894398,
145.884574100139));
#160049=CARTESIAN_POINT('Ctrl Pts',(46.2465821908671,-6.61724703464641,
145.662644640647));
#160050=CARTESIAN_POINT('Ctrl Pts',(46.0606170235145,-6.76824259322373,
145.126576057234));
#160051=CARTESIAN_POINT('Ctrl Pts',(45.8600169789493,-6.80048023565777,
144.229068979079));
#160052=CARTESIAN_POINT('Ctrl Pts',(45.7663729040281,-6.57994028199158,
143.289221553569));
#160053=CARTESIAN_POINT('Ctrl Pts',(45.7842580175622,-6.1429024671548,142.471701432123));
#160054=CARTESIAN_POINT('Ctrl Pts',(45.885543403094,-5.550920127617,141.830975748337));
#160055=CARTESIAN_POINT('Ctrl Pts',(46.034968332973,-4.87786404776204,141.388235045773));
#160056=CARTESIAN_POINT('Ctrl Pts',(46.1797023896077,-4.27548810490898,
141.165229672644));
#160057=CARTESIAN_POINT('Ctrl Pts',(46.2683547176375,-3.90838758777078,
141.095688795383));
#160058=CARTESIAN_POINT('Ctrl Pts',(46.3003354431618,-3.77501126904855,
141.078486179093));
#160059=CARTESIAN_POINT('Ctrl Pts',(47.5411678644865,-5.6196269798719,145.367772703107));
#160060=CARTESIAN_POINT('Ctrl Pts',(47.4567005603587,-5.6735582042356,145.216692900741));
#160061=CARTESIAN_POINT('Ctrl Pts',(47.2829935018905,-5.76476706996246,
144.854924187768));
#160062=CARTESIAN_POINT('Ctrl Pts',(47.0975908720934,-5.77557260627988,
144.256703390162));
#160063=CARTESIAN_POINT('Ctrl Pts',(47.0110339405536,-5.62384586859696,
143.631348870314));
#160064=CARTESIAN_POINT('Ctrl Pts',(47.0275751460305,-5.33175612882522,
143.08220807961));
#160065=CARTESIAN_POINT('Ctrl Pts',(47.1235249583571,-4.93493511480553,
142.642897466375));
#160066=CARTESIAN_POINT('Ctrl Pts',(47.2680941387717,-4.47773164599018,
142.32932716126));
#160067=CARTESIAN_POINT('Ctrl Pts',(47.4109838899983,-4.06133055703064,
142.163019363412));
#160068=CARTESIAN_POINT('Ctrl Pts',(47.4995824081453,-3.80394222364136,
142.106824516817));
#160069=CARTESIAN_POINT('Ctrl Pts',(47.5316865599187,-3.70998577779816,
142.092012095983));
#160070=CARTESIAN_POINT('Ctrl Pts',(49.085823466348,-5.78047467324188,144.999177546568));
#160071=CARTESIAN_POINT('Ctrl Pts',(49.0080675852836,-5.80813151968957,
144.864841948352));
#160072=CARTESIAN_POINT('Ctrl Pts',(48.8500905300059,-5.84600797378507,
144.554899167795));
#160073=CARTESIAN_POINT('Ctrl Pts',(48.6841202887859,-5.81401689355999,
144.070310691762));
#160074=CARTESIAN_POINT('Ctrl Pts',(48.6065150760652,-5.67306666243705,
143.567862263895));
#160075=CARTESIAN_POINT('Ctrl Pts',(48.6211264587277,-5.43349925308774,
143.106992946301));
#160076=CARTESIAN_POINT('Ctrl Pts',(48.7099577896873,-5.10370888932707,
142.7047527862));
#160077=CARTESIAN_POINT('Ctrl Pts',(48.8479614629199,-4.70105978697968,
142.380794222149));
#160078=CARTESIAN_POINT('Ctrl Pts',(48.9881514924996,-4.30757071617114,
142.179159564002));
#160079=CARTESIAN_POINT('Ctrl Pts',(49.0764615863807,-4.0511088505606,142.09635474851));
#160080=CARTESIAN_POINT('Ctrl Pts',(49.1086423835475,-3.95590192902217,
142.071681143907));
#160081=CARTESIAN_POINT('Origin',(48.9387462821982,-4.8069199738566,139.198070090029));
#160082=CARTESIAN_POINT('',(48.9057735093079,-5.78172535422313,144.973729670506));
#160083=CARTESIAN_POINT('Ctrl Pts',(48.9057735093079,-5.78172535422313,
144.973729670506));
#160084=CARTESIAN_POINT('Ctrl Pts',(48.8574830042264,-5.79875125836896,
144.886741723157));
#160085=CARTESIAN_POINT('Ctrl Pts',(48.8130418788545,-5.8111995246564,144.798629889593));
#160086=CARTESIAN_POINT('Ctrl Pts',(48.7726367086002,-5.81891384412796,
144.709933253049));
#160087=CARTESIAN_POINT('Ctrl Pts',(48.7585750597405,-5.8215985513305,144.679065397518));
#160088=CARTESIAN_POINT('Ctrl Pts',(48.7450021368848,-5.82371012549766,
144.648126322326));
#160089=CARTESIAN_POINT('Ctrl Pts',(48.7319255740939,-5.82524255184348,
144.617137367132));
#160090=CARTESIAN_POINT('Ctrl Pts',(48.6962719955212,-5.82942075096211,
144.532645198465));
#160091=CARTESIAN_POINT('Ctrl Pts',(48.6643077444896,-5.82929399145005,
144.447785980287));
#160092=CARTESIAN_POINT('Ctrl Pts',(48.6359541682921,-5.82484331547223,
144.363010384092));
#160093=CARTESIAN_POINT('Ctrl Pts',(48.6080496963055,-5.82046313562193,
144.279577584198));
#160094=CARTESIAN_POINT('Ctrl Pts',(48.5836421004334,-5.8118960502912,144.196225488765));
#160095=CARTESIAN_POINT('Ctrl Pts',(48.5626654288617,-5.79911081975773,
144.113335535882));
#160096=CARTESIAN_POINT('Ctrl Pts',(48.5598696769203,-5.79740681571865,
144.102288037431));
#160097=CARTESIAN_POINT('Ctrl Pts',(48.5571348872439,-5.79562784941034,
144.091248682514));
#160098=CARTESIAN_POINT('Ctrl Pts',(48.5544609211838,-5.79377381185531,
144.08021831539));
#160099=CARTESIAN_POINT('Ctrl Pts',(48.5511232491381,-5.7914595830357,144.066450097253));
#160100=CARTESIAN_POINT('Ctrl Pts',(48.5478803414289,-5.78902839204097,
144.052695883244));
#160101=CARTESIAN_POINT('Ctrl Pts',(48.5447307972159,-5.78648057560322,
144.038957589553));
#160102=CARTESIAN_POINT('Ctrl Pts',(48.5221573243652,-5.76821981744402,
143.94049223118));
#160103=CARTESIAN_POINT('Ctrl Pts',(48.5045343563197,-5.74398192497538,
143.842897887433));
#160104=CARTESIAN_POINT('Ctrl Pts',(48.4918543546712,-5.71388516193183,
143.746894525912));
#160105=CARTESIAN_POINT('Ctrl Pts',(48.4845454288058,-5.69653697728886,
143.691556879149));
#160106=CARTESIAN_POINT('Ctrl Pts',(48.4788793532058,-5.67724131526062,
143.63674821976));
#160107=CARTESIAN_POINT('Ctrl Pts',(48.4748586649403,-5.65601566467528,
143.582610646526));
#160108=CARTESIAN_POINT('Ctrl Pts',(48.4747413674277,-5.65539643835058,
143.581031264524));
#160109=CARTESIAN_POINT('Ctrl Pts',(48.4746254677557,-5.65477557022504,
143.579452456466));
#160110=CARTESIAN_POINT('Ctrl Pts',(48.474510967766,-5.65415306061376,143.577874225666));
#160111=CARTESIAN_POINT('Ctrl Pts',(48.4692585741228,-5.62559702726476,
143.505476931644));
#160112=CARTESIAN_POINT('Ctrl Pts',(48.466950212038,-5.59358706740297,143.43429152169));
#160113=CARTESIAN_POINT('Ctrl Pts',(48.4675859848779,-5.55825509465883,
143.364633654463));
#160114=CARTESIAN_POINT('Ctrl Pts',(48.4679108010891,-5.54020399715544,
143.32904546463));
#160115=CARTESIAN_POINT('Ctrl Pts',(48.4690041002126,-5.52128551225177,
143.293855973406));
#160116=CARTESIAN_POINT('Ctrl Pts',(48.4708659099544,-5.50151600329219,
143.259108081192));
#160117=CARTESIAN_POINT('Ctrl Pts',(48.4717968148254,-5.4916312488124,143.241734135085));
#160118=CARTESIAN_POINT('Ctrl Pts',(48.4729198473072,-5.48153372475322,
143.22447059585));
#160119=CARTESIAN_POINT('Ctrl Pts',(48.4742350105987,-5.47122544851078,
143.207322943274));
#160120=CARTESIAN_POINT('Ctrl Pts',(48.4748925922445,-5.46607131038957,
143.198749116987));
#160121=CARTESIAN_POINT('Ctrl Pts',(48.4755982065885,-5.46086448384824,
143.190204263258));
#160122=CARTESIAN_POINT('Ctrl Pts',(48.476351854012,-5.4556052200133,143.181689073789));
#160123=CARTESIAN_POINT('Ctrl Pts',(48.4767286777238,-5.45297558809582,
143.177431479055));
#160124=CARTESIAN_POINT('Ctrl Pts',(48.4771175097053,-5.4503328468415,143.173181300447));
#160125=CARTESIAN_POINT('Ctrl Pts',(48.4775183500038,-5.44767702770147,
143.168938624996));
#160126=CARTESIAN_POINT('Ctrl Pts',(48.4778243720832,-5.44564943891133,
143.165699548563));
#160127=CARTESIAN_POINT('Ctrl Pts',(48.478231074737,-5.44301375622949,143.161513471526));
#160128=CARTESIAN_POINT('Ctrl Pts',(48.4785244702588,-5.44114456717572,
143.158559835133));
#160129=CARTESIAN_POINT('Ctrl Pts',(48.4786153762513,-5.44056541557508,
143.157644677171));
#160130=CARTESIAN_POINT('Ctrl Pts',(48.4786951456533,-5.44006017141317,
143.156847647423));
#160131=CARTESIAN_POINT('Ctrl Pts',(48.4787568958971,-5.43967036809464,
143.156233195461));
#160132=CARTESIAN_POINT('Ctrl Pts',(48.4802449745291,-5.43027675353651,
143.141425920541));
#160133=CARTESIAN_POINT('Ctrl Pts',(48.4819591686244,-5.4204941631384,143.126350799725));
#160134=CARTESIAN_POINT('Ctrl Pts',(48.4839048570574,-5.41030171981581,
143.111028284083));
#160135=CARTESIAN_POINT('Ctrl Pts',(48.4884010326069,-5.38674860942085,
143.075620395019));
#160136=CARTESIAN_POINT('Ctrl Pts',(48.4941346838576,-5.36100732183593,
143.038888481324));
#160137=CARTESIAN_POINT('Ctrl Pts',(48.5011476052396,-5.33282369208186,
143.001107300327));
#160138=CARTESIAN_POINT('Ctrl Pts',(48.5078840387509,-5.30575121577626,
142.964815660952));
#160139=CARTESIAN_POINT('Ctrl Pts',(48.5158012921635,-5.27642492613411,
142.927555634262));
#160140=CARTESIAN_POINT('Ctrl Pts',(48.5249180660653,-5.24461405749319,
142.889613059426));
#160141=CARTESIAN_POINT('Ctrl Pts',(48.5335054703596,-5.21465030135375,
142.853873637389));
#160142=CARTESIAN_POINT('Ctrl Pts',(48.5431573793493,-5.18248189349009,
142.81752855818));
#160143=CARTESIAN_POINT('Ctrl Pts',(48.5538682402161,-5.14791443396958,
142.780856891134));
#160144=CARTESIAN_POINT('Ctrl Pts',(48.5610547769995,-5.12472112369863,
142.756251746186));
#160145=CARTESIAN_POINT('Ctrl Pts',(48.5687176082766,-5.10044776238925,
142.73150038102));
#160146=CARTESIAN_POINT('Ctrl Pts',(48.5768483642691,-5.07503604108531,
142.706698594798));
#160147=CARTESIAN_POINT('Ctrl Pts',(48.5883349654884,-5.03913602032692,
142.671660250501));
#160148=CARTESIAN_POINT('Ctrl Pts',(48.6007570081408,-5.00096318819923,
142.636519730009));
#160149=CARTESIAN_POINT('Ctrl Pts',(48.6140606015791,-4.96037412893768,
142.601565895071));
#160150=CARTESIAN_POINT('Ctrl Pts',(48.6155444485146,-4.95584693472676,
142.597667238584));
#160151=CARTESIAN_POINT('Ctrl Pts',(48.6170392298211,-4.95128969428845,
142.593770945232));
#160152=CARTESIAN_POINT('Ctrl Pts',(48.6185448454909,-4.94670221900433,
142.589877447084));
#160153=CARTESIAN_POINT('Ctrl Pts',(48.6312990436561,-4.90784132639545,
142.556895293708));
#160154=CARTESIAN_POINT('Ctrl Pts',(48.6447969328006,-4.86682337149193,
142.524122734055));
#160155=CARTESIAN_POINT('Ctrl Pts',(48.659112698478,-4.8235493389134,142.491842849455));
#160156=CARTESIAN_POINT('Ctrl Pts',(48.6730539457726,-4.78140740929511,
142.460407447117));
#160157=CARTESIAN_POINT('Ctrl Pts',(48.6877710045931,-4.73712575480717,
142.429439330805));
#160158=CARTESIAN_POINT('Ctrl Pts',(48.703303248073,-4.69063288592935,142.399235166709));
#160159=CARTESIAN_POINT('Ctrl Pts',(48.7056309371197,-4.68366538366385,
142.394708718098));
#160160=CARTESIAN_POINT('Ctrl Pts',(48.7079768766572,-4.67664826045055,
142.390199491961));
#160161=CARTESIAN_POINT('Ctrl Pts',(48.7103411371858,-4.66958131864314,
142.385708556192));
#160162=CARTESIAN_POINT('Ctrl Pts',(48.7260142670445,-4.62273322584015,
142.355937294251));
#160163=CARTESIAN_POINT('Ctrl Pts',(48.7424950052783,-4.57369357852764,
142.326967368551));
#160164=CARTESIAN_POINT('Ctrl Pts',(48.7598002750494,-4.52243128457966,
142.299109381492));
#160165=CARTESIAN_POINT('Ctrl Pts',(48.7766824729776,-4.47242222929603,
142.2719324546));
#160166=CARTESIAN_POINT('Ctrl Pts',(48.7943494995698,-4.42029781174223,
142.24581383713));
#160167=CARTESIAN_POINT('Ctrl Pts',(48.8127870284115,-4.36605564997263,
142.221070016252));
#160168=CARTESIAN_POINT('Ctrl Pts',(48.8294029814107,-4.31717246078438,
142.198770815082));
#160169=CARTESIAN_POINT('Ctrl Pts',(48.8466444608402,-4.26656957193763,
142.177588497048));
#160170=CARTESIAN_POINT('Ctrl Pts',(48.864477872093,-4.21426504024486,142.157774539181));
#160171=CARTESIAN_POINT('Ctrl Pts',(48.8835392481959,-4.15835894710614,
142.136596240893));
#160172=CARTESIAN_POINT('Ctrl Pts',(48.9032769193088,-4.10050744227999,
142.116981385794));
#160173=CARTESIAN_POINT('Ctrl Pts',(48.9236451106707,-4.04081169564955,
142.099235508675));
#160174=CARTESIAN_POINT('Ctrl Pts',(48.9282346510359,-4.02736052397112,
142.095236851263));
#160175=CARTESIAN_POINT('Ctrl Pts',(48.9328560941336,-4.0138158715974,142.09133316896));
#160176=CARTESIAN_POINT('Ctrl Pts',(48.9375087193678,-4.00017917397872,
142.087528100711));
#160177=CARTESIAN_POINT('Origin',(48.9104317825618,-8.72626638758926,145.547624122242));
#160178=CARTESIAN_POINT('Origin',(10.4437182387877,-3.3884479131999,144.495399400904));
#160179=CARTESIAN_POINT('',(48.9057735357879,-5.78174222830161,144.973732958521));
#160180=CARTESIAN_POINT('Ctrl Pts',(46.0225958916338,4.1854380591026,139.544563094783));
#160181=CARTESIAN_POINT('Ctrl Pts',(45.9812730775996,4.43160751792965,139.583694415389));
#160182=CARTESIAN_POINT('Ctrl Pts',(45.8817256585986,5.01513721022549,139.72158867393));
#160183=CARTESIAN_POINT('Ctrl Pts',(45.7266500710242,5.91846538933026,140.119945925672));
#160184=CARTESIAN_POINT('Ctrl Pts',(45.5790466613153,6.84385432790675,140.806566615535));
#160185=CARTESIAN_POINT('Ctrl Pts',(45.4852947783209,7.63098616909916,141.748557124114));
#160186=CARTESIAN_POINT('Ctrl Pts',(45.4813493332435,8.19023998484079,142.906059572216));
#160187=CARTESIAN_POINT('Ctrl Pts',(45.5942140393653,8.45348830956667,144.205359185367));
#160188=CARTESIAN_POINT('Ctrl Pts',(45.8026477379926,8.38883204657363,145.364075241063));
#160189=CARTESIAN_POINT('Ctrl Pts',(45.9794174121251,8.20606751734297,146.040910018887));
#160190=CARTESIAN_POINT('Ctrl Pts',(46.0534055265581,8.11631521630629,146.293329214793));
#160191=CARTESIAN_POINT('Ctrl Pts',(46.2883692083799,3.84230106733182,141.08057138548));
#160192=CARTESIAN_POINT('Ctrl Pts',(46.2471489482482,4.01187144162188,141.102561270826));
#160193=CARTESIAN_POINT('Ctrl Pts',(46.1479570361563,4.41631048619959,141.186121368824));
#160194=CARTESIAN_POINT('Ctrl Pts',(45.9938835061498,5.05252428928464,141.447777275722));
#160195=CARTESIAN_POINT('Ctrl Pts',(45.8478708762706,5.71572290838207,141.921029285075));
#160196=CARTESIAN_POINT('Ctrl Pts',(45.7556082758894,6.28688824505787,142.590694965869));
#160197=CARTESIAN_POINT('Ctrl Pts',(45.7520119369578,6.69282762784374,143.429483847216));
#160198=CARTESIAN_POINT('Ctrl Pts',(45.8631813379175,6.87599162214231,144.378537428345));
#160199=CARTESIAN_POINT('Ctrl Pts',(46.0683011093412,6.81206541535659,145.221882022372));
#160200=CARTESIAN_POINT('Ctrl Pts',(46.2425858947116,6.66552440867401,145.708123051829));
#160201=CARTESIAN_POINT('Ctrl Pts',(46.3156201733044,6.59488103790824,145.888155999971));
#160202=CARTESIAN_POINT('Ctrl Pts',(47.5199218191278,3.78062210798581,142.094063635992));
#160203=CARTESIAN_POINT('Ctrl Pts',(47.4786970341152,3.90003471796203,142.112982235428));
#160204=CARTESIAN_POINT('Ctrl Pts',(47.3800382801279,4.18312907406931,142.179733051624));
#160205=CARTESIAN_POINT('Ctrl Pts',(47.2289770169779,4.62151410983383,142.372846739715));
#160206=CARTESIAN_POINT('Ctrl Pts',(47.0887712885677,5.07077755475171,142.706010783594));
#160207=CARTESIAN_POINT('Ctrl Pts',(47.0021425885985,5.4530433520793,143.16336790427));
#160208=CARTESIAN_POINT('Ctrl Pts',(46.9992581570219,5.7246874050313,143.725580656898));
#160209=CARTESIAN_POINT('Ctrl Pts',(47.1020581503972,5.85252013288016,144.356769743511));
#160210=CARTESIAN_POINT('Ctrl Pts',(47.291745722439,5.82101797727647,144.919622760124));
#160211=CARTESIAN_POINT('Ctrl Pts',(47.4546670828204,5.73217254703968,145.248311075454));
#160212=CARTESIAN_POINT('Ctrl Pts',(47.5233698054881,5.68855250677466,145.370874265986));
#160213=CARTESIAN_POINT('Ctrl Pts',(49.0960992191677,4.03151001320818,142.073867792845));
#160214=CARTESIAN_POINT('Ctrl Pts',(49.0547651127025,4.15250410057625,142.105334310947));
#160215=CARTESIAN_POINT('Ctrl Pts',(48.9565482606377,4.43320198484628,142.201278771501));
#160216=CARTESIAN_POINT('Ctrl Pts',(48.8089901856194,4.84282216533669,142.428579800424));
#160217=CARTESIAN_POINT('Ctrl Pts',(48.6758786708201,5.23430742494674,142.765592341929));
#160218=CARTESIAN_POINT('Ctrl Pts',(48.5961869355628,5.55001534344916,143.177738603068));
#160219=CARTESIAN_POINT('Ctrl Pts',(48.5940181499387,5.77411730330242,143.645008539377));
#160220=CARTESIAN_POINT('Ctrl Pts',(48.685995886383,5.89927909395418,144.151035032819));
#160221=CARTESIAN_POINT('Ctrl Pts',(48.8559164790919,5.91554136284544,144.609747053932));
#160222=CARTESIAN_POINT('Ctrl Pts',(49.004327214937,5.87676381771975,144.893388080051));
#160223=CARTESIAN_POINT('Ctrl Pts',(49.0675053554823,5.85445183185201,145.002383852898));
#160224=CARTESIAN_POINT('',(48.8874340390554,5.85518035418594,144.976887878439));
#160225=CARTESIAN_POINT('Origin',(48.8828366595184,8.79945069508729,145.552470666265));
#160226=CARTESIAN_POINT('Ctrl Pts',(48.9248217637666,4.07524046612488,142.089743831931));
#160227=CARTESIAN_POINT('Ctrl Pts',(48.9088894384633,4.12146053551437,142.102686008398));
#160228=CARTESIAN_POINT('Ctrl Pts',(48.8936098512241,4.16551766241371,142.116452986942));
#160229=CARTESIAN_POINT('Ctrl Pts',(48.879013781374,4.20742683554834,142.130726436299));
#160230=CARTESIAN_POINT('Ctrl Pts',(48.8637859130388,4.2511500690684,142.145617719345));
#160231=CARTESIAN_POINT('Ctrl Pts',(48.8493018159786,4.29253570059324,142.161060172306));
#160232=CARTESIAN_POINT('Ctrl Pts',(48.8355701607073,4.33163089141771,142.17673234098));
#160233=CARTESIAN_POINT('Ctrl Pts',(48.8318014092585,4.34236084743149,142.181033680274));
#160234=CARTESIAN_POINT('Ctrl Pts',(48.8280892000489,4.3529184239031,142.185352551563));
#160235=CARTESIAN_POINT('Ctrl Pts',(48.8244334187919,4.36330491679753,142.189682819269));
#160236=CARTESIAN_POINT('Ctrl Pts',(48.8104461361547,4.40304438738069,142.206250735686));
#160237=CARTESIAN_POINT('Ctrl Pts',(48.7972868627936,4.44027862099375,142.222981686069));
#160238=CARTESIAN_POINT('Ctrl Pts',(48.7849407050485,4.47510737564834,142.239554542838));
#160239=CARTESIAN_POINT('Ctrl Pts',(48.7757581914447,4.50101142774503,142.251880683965));
#160240=CARTESIAN_POINT('Ctrl Pts',(48.7670248487054,4.52558515411604,142.264120430663));
#160241=CARTESIAN_POINT('Ctrl Pts',(48.7587268923065,4.5488723158606,142.276158338025));
#160242=CARTESIAN_POINT('Ctrl Pts',(48.7468529536423,4.58219501809265,142.293383949585));
#160243=CARTESIAN_POINT('Ctrl Pts',(48.7358978629908,4.61287532880214,142.310189894057));
#160244=CARTESIAN_POINT('Ctrl Pts',(48.7258666794082,4.64103991314218,142.326281092176));
#160245=CARTESIAN_POINT('Ctrl Pts',(48.7176588038369,4.6640851900906,142.339447489827));
#160246=CARTESIAN_POINT('Ctrl Pts',(48.7100689965524,4.68544632172692,142.352136432435));
#160247=CARTESIAN_POINT('Ctrl Pts',(48.7030940396954,4.7051903667889,142.364211306854));
#160248=CARTESIAN_POINT('Ctrl Pts',(48.7013109664932,4.71023772096972,142.367298119494));
#160249=CARTESIAN_POINT('Ctrl Pts',(48.6998394384133,4.71440730500938,142.369867794337));
#160250=CARTESIAN_POINT('Ctrl Pts',(48.6981205105038,4.71929092858846,142.372899133817));
#160251=CARTESIAN_POINT('Ctrl Pts',(48.6966593374644,4.72344224818082,142.375475921067));
#160252=CARTESIAN_POINT('Ctrl Pts',(48.6950192868673,4.72810971549003,142.378386076254));
#160253=CARTESIAN_POINT('Ctrl Pts',(48.6928656811989,4.73425220792585,142.382259196829));
#160254=CARTESIAN_POINT('Ctrl Pts',(48.69204717446,4.73658674461746,142.383731228286));
#160255=CARTESIAN_POINT('Ctrl Pts',(48.6911545979916,4.73913410396654,142.385342717972));
#160256=CARTESIAN_POINT('Ctrl Pts',(48.6901701315476,4.74194575257293,142.387129951436));
#160257=CARTESIAN_POINT('Ctrl Pts',(48.6835481969699,4.76085808141801,142.399151633986));
#160258=CARTESIAN_POINT('Ctrl Pts',(48.6770636059516,4.7794709581225,142.411340421246));
#160259=CARTESIAN_POINT('Ctrl Pts',(48.6707163584928,4.79778440127906,142.423681254348));
#160260=CARTESIAN_POINT('Ctrl Pts',(48.6692228600872,4.80209352871312,142.426585035031));
#160261=CARTESIAN_POINT('Ctrl Pts',(48.6677369620367,4.80638608609014,142.429497239768));
#160262=CARTESIAN_POINT('Ctrl Pts',(48.6662586623385,4.81066208145745,142.432417678715));
#160263=CARTESIAN_POINT('Ctrl Pts',(48.655171653674,4.84273135519406,142.454320498521));
#160264=CARTESIAN_POINT('Ctrl Pts',(48.6445125102291,4.87386872771066,142.476686013722));
#160265=CARTESIAN_POINT('Ctrl Pts',(48.6342809787104,4.90408376147835,142.499430874036));
#160266=CARTESIAN_POINT('Ctrl Pts',(48.6180120989511,4.95212786420115,142.535596857293));
#160267=CARTESIAN_POINT('Ctrl Pts',(48.6028051993584,4.99783953900665,142.572720744986));
#160268=CARTESIAN_POINT('Ctrl Pts',(48.5886903281095,5.04127728535629,142.61049650008));
#160269=CARTESIAN_POINT('Ctrl Pts',(48.5742119799819,5.0858336119734,142.649245031567));
#160270=CARTESIAN_POINT('Ctrl Pts',(48.5608825032169,5.12799749856814,142.6886794128));
#160271=CARTESIAN_POINT('Ctrl Pts',(48.5486991875105,5.16785428489672,142.728505144144));
#160272=CARTESIAN_POINT('Ctrl Pts',(48.5447821694551,5.18066851014064,142.741309385002));
#160273=CARTESIAN_POINT('Ctrl Pts',(48.5409833685402,5.19324441894756,142.754154350228));
#160274=CARTESIAN_POINT('Ctrl Pts',(48.5373019856571,5.20558528587342,142.767031014309));
#160275=CARTESIAN_POINT('Ctrl Pts',(48.5317708300825,5.22412702876113,142.786377774637));
#160276=CARTESIAN_POINT('Ctrl Pts',(48.5265047900417,5.24213816872921,142.80579598422));
#160277=CARTESIAN_POINT('Ctrl Pts',(48.5214984305421,5.25963270414364,142.825254404319));
#160278=CARTESIAN_POINT('Ctrl Pts',(48.5104020313479,5.29840865475055,142.868383228195));
#160279=CARTESIAN_POINT('Ctrl Pts',(48.5006077938204,5.33464508048347,142.911705535247));
#160280=CARTESIAN_POINT('Ctrl Pts',(48.4921198079405,5.36850506162563,142.954916641507));
#160281=CARTESIAN_POINT('Ctrl Pts',(48.4895903889023,5.37859533299852,142.967793547334));
#160282=CARTESIAN_POINT('Ctrl Pts',(48.4871767689155,5.38847462600499,142.980660866471));
#160283=CARTESIAN_POINT('Ctrl Pts',(48.4848785630768,5.39814739688027,142.99351124648));
#160284=CARTESIAN_POINT('Ctrl Pts',(48.4798734089431,5.41921326848959,143.021497483195));
#160285=CARTESIAN_POINT('Ctrl Pts',(48.4754172858013,5.43929967677792,143.049403125118));
#160286=CARTESIAN_POINT('Ctrl Pts',(48.4715101193556,5.45845409577054,143.077158071069));
#160287=CARTESIAN_POINT('Ctrl Pts',(48.4695565361327,5.46803130526684,143.091035544044));
#160288=CARTESIAN_POINT('Ctrl Pts',(48.4677401921302,5.47737547828869,143.104875366129));
#160289=CARTESIAN_POINT('Ctrl Pts',(48.466061077691,5.48649272826543,143.118669513915));
#160290=CARTESIAN_POINT('Ctrl Pts',(48.4652215204714,5.4910513532538,143.125566587808));
#160291=CARTESIAN_POINT('Ctrl Pts',(48.464416270646,5.49555324489794,143.132452244518));
#160292=CARTESIAN_POINT('Ctrl Pts',(48.4636453270126,5.49999916308236,143.139325504608));
#160293=CARTESIAN_POINT('Ctrl Pts',(48.4631422494356,5.5029003372419,143.143810635404));
#160294=CARTESIAN_POINT('Ctrl Pts',(48.4627271566693,5.50534082490976,143.147609135156));
#160295=CARTESIAN_POINT('Ctrl Pts',(48.4622551083268,5.50817764338732,143.152053631565));
#160296=CARTESIAN_POINT('Ctrl Pts',(48.4620037639343,5.50968812092225,143.154420124886));
#160297=CARTESIAN_POINT('Ctrl Pts',(48.461736662224,5.51131047506557,143.15697005603));
#160298=CARTESIAN_POINT('Ctrl Pts',(48.461435413493,5.51316975414571,143.159907129807));
#160299=CARTESIAN_POINT('Ctrl Pts',(48.4606569046263,5.51797463828491,143.167497329341));
#160300=CARTESIAN_POINT('Ctrl Pts',(48.4599162273016,5.52273771424791,143.17511224162));
#160301=CARTESIAN_POINT('Ctrl Pts',(48.459213646533,5.52745867760706,143.182751407617));
#160302=CARTESIAN_POINT('Ctrl Pts',(48.4514706867652,5.57948718591747,143.266940667586));
#160303=CARTESIAN_POINT('Ctrl Pts',(48.448353044463,5.62640005932763,143.354072810273));
#160304=CARTESIAN_POINT('Ctrl Pts',(48.4499804128068,5.66795182294563,143.443443931927));
#160305=CARTESIAN_POINT('Ctrl Pts',(48.4512447100305,5.7002332542409,143.512876068429));
#160306=CARTESIAN_POINT('Ctrl Pts',(48.4553731825803,5.72927947792775,143.58365999408));
#160307=CARTESIAN_POINT('Ctrl Pts',(48.4624330309206,5.75497534443534,143.655484935499));
#160308=CARTESIAN_POINT('Ctrl Pts',(48.4706470433165,5.78487204417221,143.739052022313));
#160309=CARTESIAN_POINT('Ctrl Pts',(48.4828287068606,5.81023470834922,143.824027338883));
#160310=CARTESIAN_POINT('Ctrl Pts',(48.4988171960137,5.83102386157057,143.909935807251));
#160311=CARTESIAN_POINT('Ctrl Pts',(48.5069927734158,5.84165421755082,143.953864368975));
#160312=CARTESIAN_POINT('Ctrl Pts',(48.5161640811989,5.85108838792821,143.998037560987));
#160313=CARTESIAN_POINT('Ctrl Pts',(48.5263120580339,5.85931795799407,144.042395450064));
#160314=CARTESIAN_POINT('Ctrl Pts',(48.5353637138622,5.86665845916609,144.081961203092));
#160315=CARTESIAN_POINT('Ctrl Pts',(48.5451875327568,5.8730383748811,144.121662641184));
#160316=CARTESIAN_POINT('Ctrl Pts',(48.555812740026,5.87845101381005,144.161452853898));
#160317=CARTESIAN_POINT('Ctrl Pts',(48.578289600787,5.88990106165131,144.245626183242));
#160318=CARTESIAN_POINT('Ctrl Pts',(48.6043523108742,5.89702341201655,144.330199990794));
#160319=CARTESIAN_POINT('Ctrl Pts',(48.63403389734,5.89986022843376,144.414775080605));
#160320=CARTESIAN_POINT('Ctrl Pts',(48.6642639406615,5.90274946359261,144.500912950354));
#160321=CARTESIAN_POINT('Ctrl Pts',(48.6982481968732,5.90119208749396,144.587052284651));
#160322=CARTESIAN_POINT('Ctrl Pts',(48.7360268924637,5.89522534133957,144.672718311044));
#160323=CARTESIAN_POINT('Ctrl Pts',(48.7400930294678,5.89458313792431,144.68193858174));
#160324=CARTESIAN_POINT('Ctrl Pts',(48.7442031245072,5.89388985851974,144.691153320021));
#160325=CARTESIAN_POINT('Ctrl Pts',(48.7483572288102,5.89314555373829,144.700361898933));
#160326=CARTESIAN_POINT('Ctrl Pts',(48.7903100036049,5.88562873456459,144.79336039129));
#160327=CARTESIAN_POINT('Ctrl Pts',(48.8367525975183,5.87290511982796,144.885734945757));
#160328=CARTESIAN_POINT('Ctrl Pts',(48.8874340618173,5.85516576140854,144.97688502578));
#160329=CARTESIAN_POINT('Origin',(48.9235486361196,4.8835311182205,139.200683316394));
#160330=CARTESIAN_POINT('Origin',(10.4331297884161,3.34111880277824,144.497266430389));
#160331=CARTESIAN_POINT('',(96.4093348692712,5.9299457611023,144.976966946015));
#160332=CARTESIAN_POINT('',(48.8874340344061,5.85518334895249,144.976888463869));
#160333=CARTESIAN_POINT('Ctrl Pts',(96.4093348654697,5.92994817616452,144.976967418175));
#160334=CARTESIAN_POINT('Ctrl Pts',(96.3879022801485,5.93765465679943,144.937376728462));
#160335=CARTESIAN_POINT('Ctrl Pts',(96.3649282432297,5.94484703642197,144.8953296167));
#160336=CARTESIAN_POINT('Ctrl Pts',(96.3404133194485,5.95116639403942,144.850822032184));
#160337=CARTESIAN_POINT('Ctrl Pts',(96.3163617535213,5.95736630914868,144.807155687847));
#160338=CARTESIAN_POINT('Ctrl Pts',(96.2908269994181,5.96272563710496,144.76112044886));
#160339=CARTESIAN_POINT('Ctrl Pts',(96.2638096495332,5.96686787341956,144.712745233282));
#160340=CARTESIAN_POINT('Ctrl Pts',(96.2375327979243,5.97089657828627,144.665695897699));
#160341=CARTESIAN_POINT('Ctrl Pts',(96.2098535080668,5.97377363439324,144.616432647817));
#160342=CARTESIAN_POINT('Ctrl Pts',(96.1807723742022,5.97512135805271,144.565020584938));
#160343=CARTESIAN_POINT('Ctrl Pts',(96.1757443005913,5.97535437695075,144.5561315355));
#160344=CARTESIAN_POINT('Ctrl Pts',(96.1706743206981,5.97554160861103,144.547178354883));
#160345=CARTESIAN_POINT('Ctrl Pts',(96.165562437728,5.97568101560295,144.53816151594));
#160346=CARTESIAN_POINT('Ctrl Pts',(96.1369556496969,5.97646115597219,144.487702066485));
#160347=CARTESIAN_POINT('Ctrl Pts',(96.107036591701,5.97574528489729,144.435245319868));
#160348=CARTESIAN_POINT('Ctrl Pts',(96.0758058458112,5.97316344779516,144.380900667205));
#160349=CARTESIAN_POINT('Ctrl Pts',(96.0455244413974,5.97066009248959,144.32820796461));
#160350=CARTESIAN_POINT('Ctrl Pts',(96.0140098822271,5.96640205378425,144.273740128256));
#160351=CARTESIAN_POINT('Ctrl Pts',(95.9812627241773,5.96003601986145,144.217642802994));
#160352=CARTESIAN_POINT('Ctrl Pts',(95.962724450751,5.95643218720757,144.185885923432));
#160353=CARTESIAN_POINT('Ctrl Pts',(95.9437911631774,5.9521525367929,144.153607698493));
#160354=CARTESIAN_POINT('Ctrl Pts',(95.9244629647314,5.94713142687235,144.120841865845));
#160355=CARTESIAN_POINT('Ctrl Pts',(95.9096823563841,5.94329169709042,144.095785265723));
#160356=CARTESIAN_POINT('Ctrl Pts',(95.8946708071211,5.93901834229097,144.070443622098));
#160357=CARTESIAN_POINT('Ctrl Pts',(95.8794283635279,5.9342817523375,144.044834308875));
#160358=CARTESIAN_POINT('Ctrl Pts',(95.8718071417313,5.93191345736077,144.032029652263));
#160359=CARTESIAN_POINT('Ctrl Pts',(95.8641281963653,5.92942934523654,144.019158079849));
#160360=CARTESIAN_POINT('Ctrl Pts',(95.8563915332562,5.92682571266049,144.006222002307));
#160361=CARTESIAN_POINT('Ctrl Pts',(95.8511704408754,5.92506864943911,143.997492081548));
#160362=CARTESIAN_POINT('Ctrl Pts',(95.8462652957885,5.92337618064007,143.989303169993));
#160363=CARTESIAN_POINT('Ctrl Pts',(95.8409832275859,5.92150813516453,143.980500826323));
#160364=CARTESIAN_POINT('Ctrl Pts',(95.8384382781412,5.92060809353057,143.976259775512));
#160365=CARTESIAN_POINT('Ctrl Pts',(95.8358058307864,5.91966660169065,143.971876463109));
#160366=CARTESIAN_POINT('Ctrl Pts',(95.8330083965617,5.9186525275665,143.967222690912));
#160367=CARTESIAN_POINT('Ctrl Pts',(95.8003309432189,5.90680690146184,143.912860939527));
#160368=CARTESIAN_POINT('Ctrl Pts',(95.7688813316534,5.89357318545835,143.860839945248));
#160369=CARTESIAN_POINT('Ctrl Pts',(95.7386589333837,5.87935081357124,143.811174028236));
#160370=CARTESIAN_POINT('Ctrl Pts',(95.7077195738219,5.86479104654975,143.760329894337));
#160371=CARTESIAN_POINT('Ctrl Pts',(95.6780663437034,5.84919546427068,143.711953379574));
#160372=CARTESIAN_POINT('Ctrl Pts',(95.6496986267706,5.83295573741233,143.666018673787));
#160373=CARTESIAN_POINT('Ctrl Pts',(95.6199435544842,5.81592178830307,143.617837479144));
#160374=CARTESIAN_POINT('Ctrl Pts',(95.5916028083606,5.79817958420435,143.572342295301));
#160375=CARTESIAN_POINT('Ctrl Pts',(95.5646757498473,5.78013497109662,143.529466183462));
#160376=CARTESIAN_POINT('Ctrl Pts',(95.5375525157259,5.76195889494971,143.486277700062));
#160377=CARTESIAN_POINT('Ctrl Pts',(95.5118636428781,5.74347602511105,143.44574586582));
#160378=CARTESIAN_POINT('Ctrl Pts',(95.48760855564,5.72505224209099,143.407775112115));
#160379=CARTESIAN_POINT('Ctrl Pts',(95.4626908584376,5.70612515095711,143.368767058502));
#160380=CARTESIAN_POINT('Ctrl Pts',(95.4392863541096,5.68726054276461,143.332461268972));
#160381=CARTESIAN_POINT('Ctrl Pts',(95.4173945017372,5.6688022191041,143.298736076541));
#160382=CARTESIAN_POINT('Ctrl Pts',(95.3971293265148,5.65171544376276,143.267516839247));
#160383=CARTESIAN_POINT('Ctrl Pts',(95.3781603603905,5.63497615912823,143.238508358011));
#160384=CARTESIAN_POINT('Ctrl Pts',(95.3604872361498,5.61881776534264,143.211608081182));
#160385=CARTESIAN_POINT('Ctrl Pts',(95.3423922747224,5.60227368924745,143.184065725627));
#160386=CARTESIAN_POINT('Ctrl Pts',(95.3256557539659,5.5863385644449,143.158733001856));
#160387=CARTESIAN_POINT('Ctrl Pts',(95.3102773408986,5.57122403518025,143.135500486791));
#160388=CARTESIAN_POINT('Ctrl Pts',(95.302588134365,5.56366677054793,143.123884229258));
#160389=CARTESIAN_POINT('Ctrl Pts',(95.2952384556976,5.5563140548991,143.112793074231));
#160390=CARTESIAN_POINT('Ctrl Pts',(95.2882282687808,5.54918884354847,143.102213870378));
#160391=CARTESIAN_POINT('Ctrl Pts',(95.2847231753224,5.54562623787317,143.096924268452));
#160392=CARTESIAN_POINT('Ctrl Pts',(95.2813029548454,5.54212048042549,143.09176267315));
#160393=CARTESIAN_POINT('Ctrl Pts',(95.2779676031805,5.53867422137471,143.086727477895));
#160394=CARTESIAN_POINT('Ctrl Pts',(95.276299927348,5.53695109184932,143.084209880267));
#160395=CARTESIAN_POINT('Ctrl Pts',(95.2746534687213,5.53524283515298,143.081723883828));
#160396=CARTESIAN_POINT('Ctrl Pts',(95.2730282267972,5.53354977110422,143.079269293557));
#160397=CARTESIAN_POINT('Ctrl Pts',(95.2722156058352,5.53270323907984,143.078041998422));
#160398=CARTESIAN_POINT('Ctrl Pts',(95.271408289049,5.5318605051085,143.076822554903));
#160399=CARTESIAN_POINT('Ctrl Pts',(95.270606276377,5.53102160834656,143.075610938833));
#160400=CARTESIAN_POINT('Ctrl Pts',(95.269804263705,5.53018271158462,143.074399322764));
#160401=CARTESIAN_POINT('Ctrl Pts',(95.2696238401053,5.52999491397255,143.074126875397));
#160402=CARTESIAN_POINT('Ctrl Pts',(95.2682161506428,5.52851646836343,143.071999549035));
#160403=CARTESIAN_POINT('Ctrl Pts',(95.2279525004652,5.4862290048292,143.011152375909));
#160404=CARTESIAN_POINT('Ctrl Pts',(95.1893336361188,5.44185914784464,142.953075557469));
#160405=CARTESIAN_POINT('Ctrl Pts',(95.1523589348027,5.39580271620714,142.897819507129));
#160406=CARTESIAN_POINT('Ctrl Pts',(95.1145070697088,5.34865367172546,142.841252598171));
#160407=CARTESIAN_POINT('Ctrl Pts',(95.0783783024679,5.2997374734881,142.787641662398));
#160408=CARTESIAN_POINT('Ctrl Pts',(95.0439719984758,5.24945744839374,142.736990312517));
#160409=CARTESIAN_POINT('Ctrl Pts',(95.0090901976324,5.19848255082424,142.685638958434));
#160410=CARTESIAN_POINT('Ctrl Pts',(94.9759787975812,5.14610618341306,142.637329212914));
#160411=CARTESIAN_POINT('Ctrl Pts',(94.9446371796085,5.09272158028245,142.592018014268));
#160412=CARTESIAN_POINT('Ctrl Pts',(94.9126430019111,5.03822546331901,142.545763397087));
#160413=CARTESIAN_POINT('Ctrl Pts',(94.8824930698343,4.98267899110765,142.502633151469));
#160414=CARTESIAN_POINT('Ctrl Pts',(94.8541867767856,4.92646770024733,142.462538193143));
#160415=CARTESIAN_POINT('Ctrl Pts',(94.8447279887801,4.90768422044484,142.449140122607));
#160416=CARTESIAN_POINT('Ctrl Pts',(94.8354750654485,4.88882621996806,142.436080649246));
#160417=CARTESIAN_POINT('Ctrl Pts',(94.8264279855324,4.86990721043875,142.423355507832));
#160418=CARTESIAN_POINT('Ctrl Pts',(94.7978384827799,4.81012161331499,142.383143033877));
#160419=CARTESIAN_POINT('Ctrl Pts',(94.7713045495697,4.74973024913611,142.346272127812));
#160420=CARTESIAN_POINT('Ctrl Pts',(94.7468255618325,4.68912977215539,142.312581600246));
#160421=CARTESIAN_POINT('Ctrl Pts',(94.7224659380738,4.62882479407817,142.279055353796));
#160422=CARTESIAN_POINT('Ctrl Pts',(94.7001412680888,4.56831272953028,142.248677949744));
#160423=CARTESIAN_POINT('Ctrl Pts',(94.6798510077905,4.50793940352672,142.221257865545));
#160424=CARTESIAN_POINT('Ctrl Pts',(94.6590115065883,4.44593182051244,142.193095541886));
#160425=CARTESIAN_POINT('Ctrl Pts',(94.6403180451523,4.38407075363898,142.168052361701));
#160426=CARTESIAN_POINT('Ctrl Pts',(94.6237701114008,4.32268169250134,142.145894009655));
#160427=CARTESIAN_POINT('Ctrl Pts',(94.6078575973277,4.2636498934888,142.124586510237));
#160428=CARTESIAN_POINT('Ctrl Pts',(94.5939290039647,4.20505415878326,142.105945975219));
#160429=CARTESIAN_POINT('Ctrl Pts',(94.5819839425882,4.14714157564843,142.089747519112));
#160430=CARTESIAN_POINT('Ctrl Pts',(96.3661306018733,5.88291686074446,145.149898346109));
#160431=CARTESIAN_POINT('Ctrl Pts',(96.2336307187006,5.91850508830459,144.999258634303));
#160432=CARTESIAN_POINT('Ctrl Pts',(95.9370400132557,5.95617374018587,144.673941950275));
#160433=CARTESIAN_POINT('Ctrl Pts',(95.472942825783,5.89655306604187,144.203772602427));
#160434=CARTESIAN_POINT('Ctrl Pts',(94.9958612560931,5.71763898647953,143.758389400028));
#160435=CARTESIAN_POINT('Ctrl Pts',(94.555371030275,5.43972288207611,143.375854787691));
#160436=CARTESIAN_POINT('Ctrl Pts',(94.1702186344531,5.07392883860579,143.060374039712));
#160437=CARTESIAN_POINT('Ctrl Pts',(93.8704660552985,4.64012915261243,142.825076373237));
#160438=CARTESIAN_POINT('Ctrl Pts',(93.7286434289597,4.29258168026775,142.716188456363));
#160439=CARTESIAN_POINT('Ctrl Pts',(93.6824704065431,4.12946066360959,142.680822116564));
#160440=CARTESIAN_POINT('Ctrl Pts',(96.9714505281978,6.10328824348366,144.660808028422));
#160441=CARTESIAN_POINT('Ctrl Pts',(96.8257383760717,6.14113800679038,144.494833769542));
#160442=CARTESIAN_POINT('Ctrl Pts',(96.5001479545226,6.18096509138251,144.137379834234));
#160443=CARTESIAN_POINT('Ctrl Pts',(95.9917921991142,6.11788775435994,143.622927634238));
#160444=CARTESIAN_POINT('Ctrl Pts',(95.4689973774376,5.92895072694103,143.1363614066));
#160445=CARTESIAN_POINT('Ctrl Pts',(94.9843959772261,5.63416432191659,142.717469726455));
#160446=CARTESIAN_POINT('Ctrl Pts',(94.5572977666698,5.24224883370102,142.369569651044));
#160447=CARTESIAN_POINT('Ctrl Pts',(94.2209968549404,4.7705309705759,142.107074318414));
#160448=CARTESIAN_POINT('Ctrl Pts',(94.0600652555401,4.38673321527885,141.984161786722));
#160449=CARTESIAN_POINT('Ctrl Pts',(94.0075287315537,4.20564485165057,141.944128106535));
#160450=CARTESIAN_POINT('Ctrl Pts',(97.3637713394669,5.57813458096049,144.187008423291));
#160451=CARTESIAN_POINT('Ctrl Pts',(97.2342536699332,5.61054098777057,144.040464696439));
#160452=CARTESIAN_POINT('Ctrl Pts',(96.9431219835961,5.64514693642928,143.721878689172));
#160453=CARTESIAN_POINT('Ctrl Pts',(96.4855868046259,5.59028826864809,143.257126694955));
#160454=CARTESIAN_POINT('Ctrl Pts',(96.0166230847366,5.42531605607883,142.81601143113));
#160455=CARTESIAN_POINT('Ctrl Pts',(95.5888074887858,5.17092447178584,142.440184895844));
#160456=CARTESIAN_POINT('Ctrl Pts',(95.2229838512101,4.84160297747934,142.136297152508));
#160457=CARTESIAN_POINT('Ctrl Pts',(94.9473498528165,4.46078720565056,141.916704379541));
#160458=CARTESIAN_POINT('Ctrl Pts',(94.8210499420246,4.16391263158191,141.818358906195));
#160459=CARTESIAN_POINT('Ctrl Pts',(94.7802440927429,4.02591020899387,141.786670775179));
#160460=CARTESIAN_POINT('Ctrl Pts',(97.1824258872755,4.79023850550465,144.164071510899));
#160461=CARTESIAN_POINT('Ctrl Pts',(97.0836215903891,4.8145008331457,144.053860578577));
#160462=CARTESIAN_POINT('Ctrl Pts',(96.8587285933397,4.84130595567975,143.809415735873));
#160463=CARTESIAN_POINT('Ctrl Pts',(96.500372920897,4.79878572780782,143.442656766612));
#160464=CARTESIAN_POINT('Ctrl Pts',(96.1352968151614,4.66973483371144,143.091842617071));
#160465=CARTESIAN_POINT('Ctrl Pts',(95.812959853118,4.47586755049402,142.798912924401));
#160466=CARTESIAN_POINT('Ctrl Pts',(95.5553004265918,4.24031177287435,142.575007892362));
#160467=CARTESIAN_POINT('Ctrl Pts',(95.3817764691332,3.99565053281577,142.42897685697));
#160468=CARTESIAN_POINT('Ctrl Pts',(95.3120114122748,3.82896265543311,142.371205203281));
#160469=CARTESIAN_POINT('Ctrl Pts',(95.2902462064996,3.75548982853259,142.353203306798));
#160470=CARTESIAN_POINT('Origin',(96.4108977428719,4.94854001386976,144.785115057418));
#160471=CARTESIAN_POINT('Ctrl Pts',(99.337665144168,2.68440392044039,150.587524550829));
#160472=CARTESIAN_POINT('Ctrl Pts',(99.2089333694121,3.10483363460895,150.220822132441));
#160473=CARTESIAN_POINT('Ctrl Pts',(98.8898355193563,3.90863669901366,149.388392501021));
#160474=CARTESIAN_POINT('Ctrl Pts',(98.2113149059165,4.86229080216582,147.979203699892));
#160475=CARTESIAN_POINT('Ctrl Pts',(97.2929264091547,5.52570727006287,146.495303422543));
#160476=CARTESIAN_POINT('Ctrl Pts',(96.5392326064044,5.77525244071227,145.547689944802));
#160477=CARTESIAN_POINT('Ctrl Pts',(96.1403894431067,5.86040135165679,145.102694169841));
#160478=CARTESIAN_POINT('Ctrl Pts',(100.198533022308,2.94032235979275,150.543534132445));
#160479=CARTESIAN_POINT('Ctrl Pts',(100.063340485816,3.37708324184719,150.14543555162));
#160480=CARTESIAN_POINT('Ctrl Pts',(99.7265888703645,4.21189614517861,149.240770382132));
#160481=CARTESIAN_POINT('Ctrl Pts',(99.003229305022,5.20064103458805,147.707164647165));
#160482=CARTESIAN_POINT('Ctrl Pts',(98.0176374078238,5.88575980160995,146.094117975522));
#160483=CARTESIAN_POINT('Ctrl Pts',(97.2078126465949,6.14188910510591,145.06902836783));
#160484=CARTESIAN_POINT('Ctrl Pts',(96.7800495443887,6.22910329868521,144.589455396234));
#160485=CARTESIAN_POINT('Ctrl Pts',(100.725073827536,2.56916981763826,149.916219881134));
#160486=CARTESIAN_POINT('Ctrl Pts',(100.585641409138,2.98204277130932,149.52870008216));
#160487=CARTESIAN_POINT('Ctrl Pts',(100.240256210392,3.77148792109875,148.647183663979));
#160488=CARTESIAN_POINT('Ctrl Pts',(99.5060453138298,4.70885122818818,147.14616146401));
#160489=CARTESIAN_POINT('Ctrl Pts',(98.5111164333379,5.3621183262696,145.55464168182));
#160490=CARTESIAN_POINT('Ctrl Pts',(97.6933636465612,5.60851073757937,144.532109119388));
#160491=CARTESIAN_POINT('Ctrl Pts',(97.2606142673858,5.69264552708383,144.051133856188));
#160492=CARTESIAN_POINT('Ctrl Pts',(100.366821732785,1.95896330808857,149.361400025247));
#160493=CARTESIAN_POINT('Ctrl Pts',(100.229802846635,2.33270258792801,149.015374490835));
#160494=CARTESIAN_POINT('Ctrl Pts',(99.8938301235163,3.04783157046187,148.228190526516));
#160495=CARTESIAN_POINT('Ctrl Pts',(99.1940999116348,3.90105719122696,146.882688260846));
#160496=CARTESIAN_POINT('Ctrl Pts',(98.2574617032448,4.5022176010466,145.4408636212));
#160497=CARTESIAN_POINT('Ctrl Pts',(97.4882720841481,4.73273141335164,144.498248046442));
#160498=CARTESIAN_POINT('Ctrl Pts',(97.0796829339219,4.81186143846457,144.050511405843));
#160499=CARTESIAN_POINT('',(99.4646532247826,2.77892645244027,150.519323369438));
#160500=CARTESIAN_POINT('Origin',(99.4656911297407,2.11308049683359,149.773231206415));
#160501=CARTESIAN_POINT('Ctrl Pts',(99.4646532213738,2.77892893000186,150.519326147371));
#160502=CARTESIAN_POINT('Ctrl Pts',(99.3239171368583,3.22476130620004,150.121270917057));
#160503=CARTESIAN_POINT('Ctrl Pts',(99.1608443399036,3.6176556021037,149.698516751233));
#160504=CARTESIAN_POINT('Ctrl Pts',(98.882723762233,4.13159959597354,149.048756371723));
#160505=CARTESIAN_POINT('Ctrl Pts',(98.7844315917337,4.29039944274377,148.829524813939));
#160506=CARTESIAN_POINT('Ctrl Pts',(98.628613971959,4.51071461205603,148.499009472181));
#160507=CARTESIAN_POINT('Ctrl Pts',(98.54861031565,4.61640448870926,148.333330753123));
#160508=CARTESIAN_POINT('Ctrl Pts',(98.4516063785492,4.73211758154008,148.139762058688));
#160509=CARTESIAN_POINT('Ctrl Pts',(98.4021877775759,4.78810662569635,148.042962783291));
#160510=CARTESIAN_POINT('Ctrl Pts',(98.3808119507347,4.81170504940579,148.001479921152));
#160511=CARTESIAN_POINT('Ctrl Pts',(98.3665177486058,4.8273495077737,147.973825873703));
#160512=CARTESIAN_POINT('Ctrl Pts',(98.3602561392484,4.83415188671379,147.961743928129));
#160513=CARTESIAN_POINT('Ctrl Pts',(97.8338816271381,5.40033632575454,146.949694082833));
#160514=CARTESIAN_POINT('Ctrl Pts',(97.186303247573,5.74404489420849,145.934192155672));
#160515=CARTESIAN_POINT('Ctrl Pts',(96.4093348705373,5.92994495608164,144.976966788632));
#160516=CARTESIAN_POINT('Ctrl Pts',(99.2551003701486,-2.56421655977614,
150.476238993132));
#160517=CARTESIAN_POINT('Ctrl Pts',(99.3174552930352,-2.37766070250849,
150.64908579837));
#160518=CARTESIAN_POINT('Ctrl Pts',(99.430556511845,-1.94379233761575,150.979414891096));
#160519=CARTESIAN_POINT('Ctrl Pts',(99.544239747873,-1.17789014277733,151.34060331677));
#160520=CARTESIAN_POINT('Ctrl Pts',(99.6007567400978,-0.317978856341414,
151.53240043465));
#160521=CARTESIAN_POINT('Ctrl Pts',(99.598827858709,0.563752712360761,151.530820248987));
#160522=CARTESIAN_POINT('Ctrl Pts',(99.5384938659652,1.42275402103272,151.33594849633));
#160523=CARTESIAN_POINT('Ctrl Pts',(99.4220301598475,2.18186997988765,150.974451180374));
#160524=CARTESIAN_POINT('Ctrl Pts',(99.3083038290003,2.61046752158253,150.64687566607));
#160525=CARTESIAN_POINT('Ctrl Pts',(99.2466552601123,2.79308974077101,150.477682111874));
#160526=CARTESIAN_POINT('Ctrl Pts',(100.138640963592,-2.8682884689841,150.454890705336));
#160527=CARTESIAN_POINT('Ctrl Pts',(100.208694670114,-2.66120055593453,
150.654037028246));
#160528=CARTESIAN_POINT('Ctrl Pts',(100.33547556727,-2.17890690967943,151.035071772476));
#160529=CARTESIAN_POINT('Ctrl Pts',(100.462353777589,-1.32568626788162,
151.452270093545));
#160530=CARTESIAN_POINT('Ctrl Pts',(100.52521100835,-0.366620043423776,
151.673941830286));
#160531=CARTESIAN_POINT('Ctrl Pts',(100.523061572049,0.617123998003932,
151.672105262439));
#160532=CARTESIAN_POINT('Ctrl Pts',(100.455947608549,1.57516724292511,151.446862022936));
#160533=CARTESIAN_POINT('Ctrl Pts',(100.325961028424,2.42080884665813,151.029297046142));
#160534=CARTESIAN_POINT('Ctrl Pts',(100.198485119226,2.89723385429586,150.651438085986));
#160535=CARTESIAN_POINT('Ctrl Pts',(100.129232668393,3.09995683942337,150.456496763744));
#160536=CARTESIAN_POINT('Ctrl Pts',(100.704778319826,-2.48166119443758,
149.81962164672));
#160537=CARTESIAN_POINT('Ctrl Pts',(100.770438131139,-2.30048411696688,
149.999089011321));
#160538=CARTESIAN_POINT('Ctrl Pts',(100.889538473198,-1.87930457518617,
150.341464410159));
#160539=CARTESIAN_POINT('Ctrl Pts',(101.009339216701,-1.13628925491381,
150.714884803515));
#160540=CARTESIAN_POINT('Ctrl Pts',(101.068992594997,-0.30237225732779,
150.912880544087));
#160541=CARTESIAN_POINT('Ctrl Pts',(101.067076707445,0.552612099428047,
150.911234705967));
#160542=CARTESIAN_POINT('Ctrl Pts',(101.003629074577,1.38564136001251,150.710031243453));
#160543=CARTESIAN_POINT('Ctrl Pts',(100.881100700713,2.12206307750808,150.336250397738));
#160544=CARTESIAN_POINT('Ctrl Pts',(100.761453366347,2.53811247991719,149.996699652054));
#160545=CARTESIAN_POINT('Ctrl Pts',(100.696584401853,2.71545984408411,149.821018624374));
#160546=CARTESIAN_POINT('Ctrl Pts',(100.334781367952,-1.82687938005125,
149.264716871263));
#160547=CARTESIAN_POINT('Ctrl Pts',(100.388756689852,-1.68973809771872,
149.40003391948));
#160548=CARTESIAN_POINT('Ctrl Pts',(100.487210316049,-1.37242048959108,
149.656635744138));
#160549=CARTESIAN_POINT('Ctrl Pts',(100.587396109514,-0.81669095021094,
149.934335249489));
#160550=CARTESIAN_POINT('Ctrl Pts',(100.637803032097,-0.195451852887956,
150.080979856501));
#160551=CARTESIAN_POINT('Ctrl Pts',(100.636319551743,0.440722019788662,
150.079763411599));
#160552=CARTESIAN_POINT('Ctrl Pts',(100.582977621096,1.06130906049409,149.930737936671));
#160553=CARTESIAN_POINT('Ctrl Pts',(100.480737465914,1.61213168830484,149.652741371662));
#160554=CARTESIAN_POINT('Ctrl Pts',(100.381941016435,1.92558686572514,149.398223483122));
#160555=CARTESIAN_POINT('Ctrl Pts',(100.32865219777,2.05981521819971,149.265761252093));
#160556=CARTESIAN_POINT('',(99.473036986738,-2.54943487890472,150.517848022843));
#160557=CARTESIAN_POINT('Origin',(99.4719804878147,-1.88317108232132,149.772117288637));
#160558=CARTESIAN_POINT('Ctrl Pts',(99.4730370929753,-2.54942168937959,
150.517834241583));
#160559=CARTESIAN_POINT('Ctrl Pts',(99.4967907636544,-2.45800372718185,
150.599438108881));
#160560=CARTESIAN_POINT('Ctrl Pts',(99.5190422531628,-2.36280845187909,
150.676878686175));
#160561=CARTESIAN_POINT('Ctrl Pts',(99.5397843712218,-2.26429015953294,
150.749807891744));
#160562=CARTESIAN_POINT('Ctrl Pts',(99.5588049325091,-2.17394870008527,
150.816684110471));
#160563=CARTESIAN_POINT('Ctrl Pts',(99.5765561600325,-2.08081184155517,
150.879767029523));
#160564=CARTESIAN_POINT('Ctrl Pts',(99.5930244071844,-1.98519308909147,
150.938780862268));
#160565=CARTESIAN_POINT('Ctrl Pts',(99.6116311293227,-1.87715781721955,
151.005457903125));
#160566=CARTESIAN_POINT('Ctrl Pts',(99.6286004374752,-1.76595472631711,
151.06694195465));
#160567=CARTESIAN_POINT('Ctrl Pts',(99.643952288382,-1.65209645148321,151.123024043958));
#160568=CARTESIAN_POINT('Ctrl Pts',(99.6589673571929,-1.54073594898108,
151.177875829266));
#160569=CARTESIAN_POINT('Ctrl Pts',(99.672435055107,-1.42683458110589,151.227560161432));
#160570=CARTESIAN_POINT('Ctrl Pts',(99.6843608369159,-1.31083708730611,
151.271851020231));
#160571=CARTESIAN_POINT('Ctrl Pts',(99.6886764526795,-1.26886075226889,
151.287878676236));
#160572=CARTESIAN_POINT('Ctrl Pts',(99.6927866424733,-1.22661521653128,
151.303197623039));
#160573=CARTESIAN_POINT('Ctrl Pts',(99.6966927939439,-1.18412164531507,
151.317796448963));
#160574=CARTESIAN_POINT('Ctrl Pts',(99.7082673799082,-1.05820602307792,
151.361055233705));
#160575=CARTESIAN_POINT('Ctrl Pts',(99.7180514421784,-0.930114803646029,
151.397994194935));
#160576=CARTESIAN_POINT('Ctrl Pts',(99.7260629675267,-0.800515119850276,
151.42849131307));
#160577=CARTESIAN_POINT('Ctrl Pts',(99.7342791243167,-0.667605183764806,
151.459767392636));
#160578=CARTESIAN_POINT('Ctrl Pts',(99.7406310504297,-0.533107903563072,
151.484268636455));
#160579=CARTESIAN_POINT('Ctrl Pts',(99.7451235870627,-0.397717906999669,
151.501817647624));
#160580=CARTESIAN_POINT('Ctrl Pts',(99.7459852571904,-0.371750057398373,
151.505183554222));
#160581=CARTESIAN_POINT('Ctrl Pts',(99.7467784829984,-0.345749317034777,
151.50829356699));
#160582=CARTESIAN_POINT('Ctrl Pts',(99.7475032390071,-0.319720526119759,
151.511146234637));
#160583=CARTESIAN_POINT('Ctrl Pts',(99.7513019523685,-0.183294039644338,
151.526098117166));
#160584=CARTESIAN_POINT('Ctrl Pts',(99.7532207755369,-0.0460971937661941,
151.533984298809));
#160585=CARTESIAN_POINT('Ctrl Pts',(99.7532263328386,0.0911428227613257,
151.53483434725));
#160586=CARTESIAN_POINT('Ctrl Pts',(99.7532266541401,0.0990775060141712,
151.53488349374));
#160587=CARTESIAN_POINT('Ctrl Pts',(99.7532205761433,0.107012333705595,
151.534909106638));
#160588=CARTESIAN_POINT('Ctrl Pts',(99.7532080909945,0.114947165176344,
151.534911186577));
#160589=CARTESIAN_POINT('Ctrl Pts',(99.7529922360277,0.252131977130439,
151.534947146512));
#160590=CARTESIAN_POINT('Ctrl Pts',(99.750862512385,0.389312840358846,151.527953067603));
#160591=CARTESIAN_POINT('Ctrl Pts',(99.7468548063207,0.525763867825583,
151.513907100217));
#160592=CARTESIAN_POINT('Ctrl Pts',(99.746460230677,0.539198049657002,151.512524215212));
#160593=CARTESIAN_POINT('Ctrl Pts',(99.7460474402716,0.552625155116682,
151.511072934287));
#160594=CARTESIAN_POINT('Ctrl Pts',(99.7456164621056,0.566044489218804,
151.50955320999));
#160595=CARTESIAN_POINT('Ctrl Pts',(99.7412592908233,0.701713397260867,
151.494188860731));
#160596=CARTESIAN_POINT('Ctrl Pts',(99.7350442956388,0.8365891929933,151.471832748309));
#160597=CARTESIAN_POINT('Ctrl Pts',(99.7269706645698,0.969980999090229,
151.44267400733));
#160598=CARTESIAN_POINT('Ctrl Pts',(99.7190966259891,1.10007515605482,151.414236114952));
#160599=CARTESIAN_POINT('Ctrl Pts',(99.7094546995143,1.22875858640403,151.379327502489));
#160600=CARTESIAN_POINT('Ctrl Pts',(99.6980307644927,1.35536927061228,151.338080916739));
#160601=CARTESIAN_POINT('Ctrl Pts',(99.695791476652,1.38018714336065,151.329995876184));
#160602=CARTESIAN_POINT('Ctrl Pts',(99.6934836773458,1.40492528777928,151.321667186016));
#160603=CARTESIAN_POINT('Ctrl Pts',(99.6911071985347,1.4295785787438,151.313095661014));
#160604=CARTESIAN_POINT('Ctrl Pts',(99.6875196942425,1.46679489506052,151.300156188299));
#160605=CARTESIAN_POINT('Ctrl Pts',(99.6837756845175,1.50381785429284,151.286663340033));
#160606=CARTESIAN_POINT('Ctrl Pts',(99.679874274618,1.5406332263635,151.272624883438));
#160607=CARTESIAN_POINT('Ctrl Pts',(99.6671718234397,1.66049898730303,151.226917609886));
#160608=CARTESIAN_POINT('Ctrl Pts',(99.6528294412209,1.77812313234566,151.175445798303));
#160609=CARTESIAN_POINT('Ctrl Pts',(99.6368427551107,1.89301492572233,151.118461815472));
#160610=CARTESIAN_POINT('Ctrl Pts',(99.6208560690006,2.007906719099,151.061477832642));
#160611=CARTESIAN_POINT('Ctrl Pts',(99.6032251344703,2.12006702692561,150.998981439821));
#160612=CARTESIAN_POINT('Ctrl Pts',(99.5839310026564,2.22896582916987,150.931191398442));
#160613=CARTESIAN_POINT('Ctrl Pts',(99.5654544575536,2.33325005665961,150.866273952601));
#160614=CARTESIAN_POINT('Ctrl Pts',(99.5454524324123,2.43454341641421,150.796500723107));
#160615=CARTESIAN_POINT('Ctrl Pts',(99.5239442995816,2.53243417303878,150.722234507839));
#160616=CARTESIAN_POINT('Ctrl Pts',(99.5053093488977,2.61724811000267,150.657889207859));
#160617=CARTESIAN_POINT('Ctrl Pts',(99.4855436277826,2.69950746674519,150.590170673406));
#160618=CARTESIAN_POINT('Ctrl Pts',(99.4646532434582,2.77891385967415,150.519309253246));
#160619=CARTESIAN_POINT('Ctrl Pts',(96.1095365604538,-5.64870947579686,
145.045115075205));
#160620=CARTESIAN_POINT('Ctrl Pts',(96.5308572053903,-5.56138843522124,
145.511012473416));
#160621=CARTESIAN_POINT('Ctrl Pts',(97.3048934612808,-5.30688486101267,
146.482060103913));
#160622=CARTESIAN_POINT('Ctrl Pts',(98.2343781408756,-4.6269474203888,147.991604985967));
#160623=CARTESIAN_POINT('Ctrl Pts',(98.9053783050068,-3.67234523172437,
149.395383695081));
#160624=CARTESIAN_POINT('Ctrl Pts',(99.219715834908,-2.87142907890009,150.223119336563));
#160625=CARTESIAN_POINT('Ctrl Pts',(99.3457480689541,-2.45535167201243,
150.586091782663));
#160626=CARTESIAN_POINT('Ctrl Pts',(96.7468070029816,-6.0153691110066,144.527455594643));
#160627=CARTESIAN_POINT('Ctrl Pts',(97.1986237871683,-5.92590634547683,
145.029389432178));
#160628=CARTESIAN_POINT('Ctrl Pts',(98.030381371963,-5.66464784836167,146.07975379349));
#160629=CARTESIAN_POINT('Ctrl Pts',(99.0279249426309,-4.96236056855711,
147.720706798807));
#160630=CARTESIAN_POINT('Ctrl Pts',(99.7432909122569,-3.97258298620063,
149.248390941142));
#160631=CARTESIAN_POINT('Ctrl Pts',(100.075045233077,-3.14077141997281,
150.1479213953));
#160632=CARTESIAN_POINT('Ctrl Pts',(100.207417619345,-2.7085365723338,150.541960252375));
#160633=CARTESIAN_POINT('Ctrl Pts',(97.2250643942494,-5.47673623309786,
143.989247026138));
#160634=CARTESIAN_POINT('Ctrl Pts',(97.6822311747899,-5.3903411805755,144.492877723975));
#160635=CARTESIAN_POINT('Ctrl Pts',(98.522147759943,-5.13884423720621,145.540803825402));
#160636=CARTESIAN_POINT('Ctrl Pts',(99.5292924902613,-4.46910785789018,
147.159680949567));
#160637=CARTESIAN_POINT('Ctrl Pts',(100.255659340856,-3.5306784397147,148.654798928096));
#160638=CARTESIAN_POINT('Ctrl Pts',(100.596147424224,-2.74400478658357,
149.531291089658));
#160639=CARTESIAN_POINT('Ctrl Pts',(100.73278812393,-2.33538045653838,149.91485216498));
#160640=CARTESIAN_POINT('Ctrl Pts',(97.0443195895004,-4.59591890240999,
143.993153840071));
#160641=CARTESIAN_POINT('Ctrl Pts',(97.4760971262335,-4.51459389265265,
144.462367854611));
#160642=CARTESIAN_POINT('Ctrl Pts',(98.2660806423517,-4.2791698662904,145.428649758681));
#160643=CARTESIAN_POINT('Ctrl Pts',(99.2143313698502,-3.66285513158594,
146.895045994121));
#160644=CARTESIAN_POINT('Ctrl Pts',(99.9068334220222,-2.80861603887669,
148.235172164511));
#160645=CARTESIAN_POINT('Ctrl Pts',(100.238241619548,-2.0959246702422,149.017878068064));
#160646=CARTESIAN_POINT('Ctrl Pts',(100.372616530784,-1.725995449577,149.360371055165));
#160647=CARTESIAN_POINT('Ctrl Pts',(96.427651149101,-5.7069724840649,144.973748561044));
#160648=CARTESIAN_POINT('Ctrl Pts',(96.8158651387083,-5.61306171775944,
145.452438011694));
#160649=CARTESIAN_POINT('Ctrl Pts',(97.171604962232,-5.48012191275615,145.945011203003));
#160650=CARTESIAN_POINT('Ctrl Pts',(97.6564854549691,-5.21073108191675,
146.692342036475));
#160651=CARTESIAN_POINT('Ctrl Pts',(97.8099907649047,-5.10928297209183,
146.942820946374));
#160652=CARTESIAN_POINT('Ctrl Pts',(98.0280644635696,-4.93837235096895,
147.318647637176));
#160653=CARTESIAN_POINT('Ctrl Pts',(98.134055249843,-4.84823465053843,147.506583806796));
#160654=CARTESIAN_POINT('Ctrl Pts',(98.2523801652375,-4.73463088675781,
147.72541212867));
#160655=CARTESIAN_POINT('Ctrl Pts',(98.3102098271935,-4.67568945239159,
147.834656478391));
#160656=CARTESIAN_POINT('Ctrl Pts',(98.3347083642041,-4.64996734854966,
147.881432356425));
#160657=CARTESIAN_POINT('Ctrl Pts',(98.3509772541781,-4.63271639820428,
147.912605932851));
#160658=CARTESIAN_POINT('Ctrl Pts',(98.3599854147836,-4.62306026553232,
147.929934964988));
#160659=CARTESIAN_POINT('Ctrl Pts',(98.8257446738414,-4.11935561886744,
148.828797248321));
#160660=CARTESIAN_POINT('Ctrl Pts',(99.194390231184,-3.44146052063285,149.721292814617));
#160661=CARTESIAN_POINT('Ctrl Pts',(99.473036986738,-2.54943487890472,150.517848022843));
#160662=CARTESIAN_POINT('Origin',(10.4321358521839,3.97302152633873,143.060605499564));
#160663=CARTESIAN_POINT('',(49.4092281495269,-5.40355622549669,146.366089006391));
#160664=CARTESIAN_POINT('Ctrl Pts',(49.4092280986553,-5.40355634587169,
146.366088876705));
#160665=CARTESIAN_POINT('Ctrl Pts',(49.3491597421002,-5.45696437357856,
146.213866663286));
#160666=CARTESIAN_POINT('Ctrl Pts',(49.290306060662,-5.50657128304731,146.06068333748));
#160667=CARTESIAN_POINT('Ctrl Pts',(49.2328669231528,-5.55235928450432,
145.906764540479));
#160668=CARTESIAN_POINT('Ctrl Pts',(49.1754277856436,-5.59814728596133,
145.752845743478));
#160669=CARTESIAN_POINT('Ctrl Pts',(49.1194032009783,-5.64012204557869,
145.598193572679));
#160670=CARTESIAN_POINT('Ctrl Pts',(49.0648470750591,-5.67835385863493,
145.442664128815));
#160671=CARTESIAN_POINT('Ctrl Pts',(49.0102909491892,-5.71658567165666,
145.28713468509));
#160672=CARTESIAN_POINT('Ctrl Pts',(48.9572032709229,-5.75106745791676,
145.130726057922));
#160673=CARTESIAN_POINT('Ctrl Pts',(48.9057735451051,-5.78174806146419,
144.973734095918));
#160674=CARTESIAN_POINT('',(38.9567113513846,-2.64466323934818,150.517847233856));
#160675=CARTESIAN_POINT('',(10.4426172265712,-2.68952697959015,150.5178394068));
#160676=CARTESIAN_POINT('',(47.1095722443351,-3.69329671363621,149.41195583582));
#160677=CARTESIAN_POINT('Origin',(78.0899422202629,1.83103694728723,145.20567672441));
#160678=CARTESIAN_POINT('Ctrl Pts',(47.1095722444578,-3.69329671364967,
149.411955835804));
#160679=CARTESIAN_POINT('Ctrl Pts',(47.2250608567621,-3.70596734775424,
149.396325837562));
#160680=CARTESIAN_POINT('Ctrl Pts',(47.3379399188308,-3.72201473963128,
149.376504407765));
#160681=CARTESIAN_POINT('Ctrl Pts',(47.4482092787277,-3.7413423142383,149.352413744352));
#160682=CARTESIAN_POINT('Ctrl Pts',(47.497914144081,-3.75005438524646,149.341554669969));
#160683=CARTESIAN_POINT('Ctrl Pts',(47.5470887605488,-3.75943237519231,
149.329827732654));
#160684=CARTESIAN_POINT('Ctrl Pts',(47.5957331098251,-3.76946464813312,
149.317223755553));
#160685=CARTESIAN_POINT('Ctrl Pts',(47.6740135964019,-3.78560899416637,
149.296940917465));
#160686=CARTESIAN_POINT('Ctrl Pts',(47.7509208738446,-3.8034483330406,149.274387246225));
#160687=CARTESIAN_POINT('Ctrl Pts',(47.8264548506386,-3.82292449585361,
149.249517889484));
#160688=CARTESIAN_POINT('Ctrl Pts',(47.8642218390356,-3.83266257726011,
149.237083211113));
#160689=CARTESIAN_POINT('Ctrl Pts',(47.9016455019917,-3.84280968744087,
149.224069472177));
#160690=CARTESIAN_POINT('Ctrl Pts',(47.9387258262457,-3.85335739730775,
149.210470352909));
#160691=CARTESIAN_POINT('Ctrl Pts',(47.9572659883727,-3.8586312522412,149.203670793275));
#160692=CARTESIAN_POINT('Ctrl Pts',(47.9757203158068,-3.86400524608101,
149.196724879813));
#160693=CARTESIAN_POINT('Ctrl Pts',(47.9940888067782,-3.86947825385059,
149.189631776819));
#160694=CARTESIAN_POINT('Ctrl Pts',(48.0032730522639,-3.87221475773538,
149.186085225322));
#160695=CARTESIAN_POINT('Ctrl Pts',(48.0124358386328,-3.87497601440758,
149.182501875903));
#160696=CARTESIAN_POINT('Ctrl Pts',(48.0215771656565,-3.87776187865116,
149.178881621419));
#160697=CARTESIAN_POINT('Ctrl Pts',(48.0307184926802,-3.88054774289474,
149.175261366934));
#160698=CARTESIAN_POINT('Ctrl Pts',(48.0384895838107,-3.88293795566613,
149.172151843211));
#160699=CARTESIAN_POINT('Ctrl Pts',(48.0489367684588,-3.88619314595116,
149.167910033663));
#160700=CARTESIAN_POINT('Ctrl Pts',(48.1325142456436,-3.91223466823139,
149.13397555728));
#160701=CARTESIAN_POINT('Ctrl Pts',(48.2105006971708,-3.93849865056287,
149.099313094295));
#160702=CARTESIAN_POINT('Ctrl Pts',(48.2828960847917,-3.96496078184916,
149.063908828405));
#160703=CARTESIAN_POINT('Ctrl Pts',(48.3190937786021,-3.97819184749231,
149.046206695461));
#160704=CARTESIAN_POINT('Ctrl Pts',(48.3538937064191,-3.99147243962569,
149.028319103758));
#160705=CARTESIAN_POINT('Ctrl Pts',(48.3872958632832,-4.00479940600968,
149.010244344515));
#160706=CARTESIAN_POINT('Ctrl Pts',(48.4039969417152,-4.01146288920168,
149.001206964894));
#160707=CARTESIAN_POINT('Ctrl Pts',(48.420348577408,-4.01813796530156,148.992122792891));
#160708=CARTESIAN_POINT('Ctrl Pts',(48.4363507697328,-4.02482423463313,
148.982991614239));
#160709=CARTESIAN_POINT('Ctrl Pts',(48.4523529620575,-4.0315105039647,148.973860435586));
#160710=CARTESIAN_POINT('Ctrl Pts',(48.4665509922826,-4.03757028624714,
148.965559208935));
#160711=CARTESIAN_POINT('Ctrl Pts',(48.4833090159683,-4.04491621910288,
148.955456843318));
#160712=CARTESIAN_POINT('Ctrl Pts',(48.5503411107113,-4.07429995052582,
148.915047380851));
#160713=CARTESIAN_POINT('Ctrl Pts',(48.6170655970785,-4.10661450778534,
148.869993246045));
#160714=CARTESIAN_POINT('Ctrl Pts',(48.6834821181227,-4.14163300915733,
148.820141215516));
#160715=CARTESIAN_POINT('Ctrl Pts',(48.7166903786448,-4.15914225984333,
148.795215200252));
#160716=CARTESIAN_POINT('Ctrl Pts',(48.7498216466353,-4.1773267332877,148.769089329175));
#160717=CARTESIAN_POINT('Ctrl Pts',(48.7828758700986,-4.19615338042924,
148.741742335125));
#160718=CARTESIAN_POINT('Ctrl Pts',(48.7994029818303,-4.20556670400001,
148.7280688381));
#160719=CARTESIAN_POINT('Ctrl Pts',(48.815910832362,-4.21514052762869,148.714090030498));
#160720=CARTESIAN_POINT('Ctrl Pts',(48.8323994147077,-4.22487041093803,
148.699803147087));
#160721=CARTESIAN_POINT('Ctrl Pts',(48.8406437058805,-4.2297353525927,148.692659705382));
#160722=CARTESIAN_POINT('Ctrl Pts',(48.8488831800026,-4.23463930647713,
148.685439242854));
#160723=CARTESIAN_POINT('Ctrl Pts',(48.8571178361721,-4.23958169931045,
148.678141405679));
#160724=CARTESIAN_POINT('Ctrl Pts',(48.8653524923415,-4.24452409214377,
148.670843568505));
#160725=CARTESIAN_POINT('Ctrl Pts',(48.8726808850653,-4.24895488646809,
148.66428518402));
#160726=CARTESIAN_POINT('Ctrl Pts',(48.8818073499018,-4.25452360954717,
148.656015410472));
#160727=CARTESIAN_POINT('Ctrl Pts',(48.954819068594,-4.29907339417987,148.589857222094));
#160728=CARTESIAN_POINT('Ctrl Pts',(49.0211326158252,-4.34298379382797,
148.52295350218));
#160729=CARTESIAN_POINT('Ctrl Pts',(49.080747947528,-4.3862268024775,148.455313496479));
#160730=CARTESIAN_POINT('Ctrl Pts',(49.1105556133794,-4.40784830680226,
148.421493493629));
#160731=CARTESIAN_POINT('Ctrl Pts',(49.1386887253575,-4.42930296893276,
148.387489422859));
#160732=CARTESIAN_POINT('Ctrl Pts',(49.165147277924,-4.45058726912027,148.353302546057));
#160733=CARTESIAN_POINT('Ctrl Pts',(49.1783765542072,-4.46122941921402,
148.336209107656));
#160734=CARTESIAN_POINT('Ctrl Pts',(49.1911871906381,-4.47182897919932,
148.319069967993));
#160735=CARTESIAN_POINT('Ctrl Pts',(49.2035791865256,-4.482385509894,148.301885288595));
#160736=CARTESIAN_POINT('Ctrl Pts',(49.2097751844694,-4.48766377524133,
148.293292948896));
#160737=CARTESIAN_POINT('Ctrl Pts',(49.2158665222773,-4.49293128328941,
148.284689224277));
#160738=CARTESIAN_POINT('Ctrl Pts',(49.221853199863,-4.49818797909476,148.276074135321));
#160739=CARTESIAN_POINT('Ctrl Pts',(49.2278398774487,-4.5034446749001,148.267459046365));
#160740=CARTESIAN_POINT('Ctrl Pts',(49.2329204522465,-4.50796435012504,
148.260030839577));
#160741=CARTESIAN_POINT('Ctrl Pts',(49.239499251867,-4.5139255748782,148.25019479617));
#160742=CARTESIAN_POINT('Ctrl Pts',(49.2921296488308,-4.56161537290345,
148.17150644892));
#160743=CARTESIAN_POINT('Ctrl Pts',(49.3390031528632,-4.61090243896194,
148.087760156192));
#160744=CARTESIAN_POINT('Ctrl Pts',(49.380119120392,-4.66137771917959,147.998763592685));
#160745=CARTESIAN_POINT('Ctrl Pts',(49.4006771041563,-4.68661535928841,
147.954265310931));
#160746=CARTESIAN_POINT('Ctrl Pts',(49.4197957024886,-4.71214922277214,
147.908454436313));
#160747=CARTESIAN_POINT('Ctrl Pts',(49.4374748269396,-4.73792309186303,
147.861307082455));
#160748=CARTESIAN_POINT('Ctrl Pts',(49.4463143891651,-4.75081002640847,
147.837733405526));
#160749=CARTESIAN_POINT('Ctrl Pts',(49.4547940828577,-4.76375692252418,
147.813825587123));
#160750=CARTESIAN_POINT('Ctrl Pts',(49.4629138964232,-4.77675641113063,
147.78958070489));
#160751=CARTESIAN_POINT('Ctrl Pts',(49.4669738032059,-4.78325615543385,
147.777458263774));
#160752=CARTESIAN_POINT('Ctrl Pts',(49.4709437399531,-4.78976904542875,
147.765251555352));
#160753=CARTESIAN_POINT('Ctrl Pts',(49.4748237051864,-4.79629414152205,
147.752960213411));
#160754=CARTESIAN_POINT('Ctrl Pts',(49.4784039650958,-4.80231521092417,
147.741618307971));
#160755=CARTESIAN_POINT('Ctrl Pts',(49.4815970221161,-4.80779628353553,
147.731249998675));
#160756=CARTESIAN_POINT('Ctrl Pts',(49.4852626826503,-4.81426031384824,
147.718960370922));
#160757=CARTESIAN_POINT('Ctrl Pts',(49.4855695369027,-4.81480142101586,
147.717931600118));
#160758=CARTESIAN_POINT('Ctrl Pts',(49.4858797028569,-4.81534938937098,
147.716889351646));
#160759=CARTESIAN_POINT('Ctrl Pts',(49.486193684848,-4.81590509673314,147.715831919202));
#160760=CARTESIAN_POINT('Ctrl Pts',(49.5512303180725,-4.93101149428575,
147.496800739188));
#160761=CARTESIAN_POINT('Ctrl Pts',(49.577334938451,-5.03759764333394,147.274340771407));
#160762=CARTESIAN_POINT('Ctrl Pts',(49.5645073883648,-5.13556346529849,
147.049151818323));
#160763=CARTESIAN_POINT('Ctrl Pts',(49.5516798382786,-5.23352928726304,
146.823962865239));
#160764=CARTESIAN_POINT('Ctrl Pts',(49.4999201179697,-5.32287493596084,
146.59604521302));
#160765=CARTESIAN_POINT('Ctrl Pts',(49.409228157871,-5.40355629319227,146.366089026851));
#160766=CARTESIAN_POINT('Ctrl Pts',(46.6241051349778,-7.32511472728899,
147.989854517212));
#160767=CARTESIAN_POINT('Ctrl Pts',(46.5537157353721,-7.41755726094091,
147.775546153899));
#160768=CARTESIAN_POINT('Ctrl Pts',(46.4047646446039,-7.60394202424138,
147.307357450064));
#160769=CARTESIAN_POINT('Ctrl Pts',(46.2105242916428,-7.8201965195852,146.648322053017));
#160770=CARTESIAN_POINT('Ctrl Pts',(46.0890577707829,-7.939124533019,146.203240389833));
#160771=CARTESIAN_POINT('Ctrl Pts',(46.0413559492253,-7.98304327208021,
146.022524042131));
#160772=CARTESIAN_POINT('Ctrl Pts',(46.9398378390672,-5.94714561945616,
147.399100431922));
#160773=CARTESIAN_POINT('Ctrl Pts',(46.8697497468136,-6.02854475709611,
147.210712584582));
#160774=CARTESIAN_POINT('Ctrl Pts',(46.7215167708399,-6.1926836074711,146.799123352895));
#160775=CARTESIAN_POINT('Ctrl Pts',(46.5284183447193,-6.38318097309383,
146.219681184828));
#160776=CARTESIAN_POINT('Ctrl Pts',(46.4077662646162,-6.48797605067776,
145.828311551126));
#160777=CARTESIAN_POINT('Ctrl Pts',(46.3603984301429,-6.52668138904934,
145.669397775977));
#160778=CARTESIAN_POINT('Ctrl Pts',(48.1092317625503,-5.18444440048026,
146.768005238018));
#160779=CARTESIAN_POINT('Ctrl Pts',(48.0402970656098,-5.25307065169244,
146.597191040467));
#160780=CARTESIAN_POINT('Ctrl Pts',(47.8947955416849,-5.39066904764671,
146.225153440396));
#160781=CARTESIAN_POINT('Ctrl Pts',(47.7059995187861,-5.54827456352389,
145.704630860055));
#160782=CARTESIAN_POINT('Ctrl Pts',(47.5883979384804,-5.63374760400384,
145.354785493422));
#160783=CARTESIAN_POINT('Ctrl Pts',(47.5422785802052,-5.66509900665306,
145.212986568709));
#160784=CARTESIAN_POINT('Ctrl Pts',(49.5798793716172,-5.39730189362096,
146.394690665637));
#160785=CARTESIAN_POINT('Ctrl Pts',(49.5124053079744,-5.45745952492184,
146.224801672306));
#160786=CARTESIAN_POINT('Ctrl Pts',(49.3703582684564,-5.57676031435096,
145.856584151351));
#160787=CARTESIAN_POINT('Ctrl Pts',(49.1869927219503,-5.70987697211657,
145.346474617428));
#160788=CARTESIAN_POINT('Ctrl Pts',(49.0732366813086,-5.7799663706731,145.006350194313));
#160789=CARTESIAN_POINT('Ctrl Pts',(49.0286905233209,-5.80529721278276,
144.868893549847));
#160790=CARTESIAN_POINT('Origin',(49.4136832107095,-8.23492065935952,147.357731263197));
#160791=CARTESIAN_POINT('Ctrl Pts',(45.9818308006136,-4.36386233890014,
139.457590298979));
#160792=CARTESIAN_POINT('Ctrl Pts',(46.0577929151188,-3.88656671250596,
139.336024689025));
#160793=CARTESIAN_POINT('Ctrl Pts',(46.1911667285702,-2.88574456343811,
139.125038002339));
#160794=CARTESIAN_POINT('Ctrl Pts',(46.3079233121362,-1.38770401599913,
138.941983369662));
#160795=CARTESIAN_POINT('Ctrl Pts',(46.3305159825606,-0.371913621033629,
138.9052711071));
#160796=CARTESIAN_POINT('Ctrl Pts',(46.3283370115851,0.114046639445121,
138.907567120453));
#160797=CARTESIAN_POINT('Ctrl Pts',(46.1843239563542,-3.94379274885482,
141.045963619328));
#160798=CARTESIAN_POINT('Ctrl Pts',(46.2608245032563,-3.51190343660015,
140.936336715849));
#160799=CARTESIAN_POINT('Ctrl Pts',(46.3952244407994,-2.60648107776861,
140.746127006659));
#160800=CARTESIAN_POINT('Ctrl Pts',(46.513041603105,-1.25166766168089,140.581163907621));
#160801=CARTESIAN_POINT('Ctrl Pts',(46.5359620147019,-0.333143630120858,
140.548086533492));
#160802=CARTESIAN_POINT('Ctrl Pts',(46.5338464962686,0.106283523993099,
140.550155751043));
#160803=CARTESIAN_POINT('Ctrl Pts',(47.4378078356412,-3.8343211672685,142.121689142346));
#160804=CARTESIAN_POINT('Ctrl Pts',(47.5172130409551,-3.41696992847953,
142.010153939069));
#160805=CARTESIAN_POINT('Ctrl Pts',(47.6570624441036,-2.53923231521643,
141.815778143772));
#160806=CARTESIAN_POINT('Ctrl Pts',(47.7800889888078,-1.21952845390115,
141.646213777249));
#160807=CARTESIAN_POINT('Ctrl Pts',(47.8041216550563,-0.322730017030245,
141.612114186466));
#160808=CARTESIAN_POINT('Ctrl Pts',(47.8019622839384,0.106274688630286,
141.614239265262));
#160809=CARTESIAN_POINT('Ctrl Pts',(49.072697213247,-4.09392505430371,142.110136489086));
#160810=CARTESIAN_POINT('Ctrl Pts',(49.1558216943686,-3.65247770942299,
141.983865354168));
#160811=CARTESIAN_POINT('Ctrl Pts',(49.3026329125726,-2.71992117719697,
141.762605846383));
#160812=CARTESIAN_POINT('Ctrl Pts',(49.432234898711,-1.3084544943288,141.568205313321));
#160813=CARTESIAN_POINT('Ctrl Pts',(49.4575701896293,-0.346235519011063,
141.528972447798));
#160814=CARTESIAN_POINT('Ctrl Pts',(49.4552830858161,0.114024853025236,
141.531406204995));
#160815=CARTESIAN_POINT('Origin',(49.3053670001028,0.0391433951441804,138.53495912845));
#160816=CARTESIAN_POINT('Ctrl Pts',(46.3285875541939,-0.0453398318882474,
138.90752266128));
#160817=CARTESIAN_POINT('Ctrl Pts',(46.3292442208751,0.445985702815633,
138.90547547437));
#160818=CARTESIAN_POINT('Ctrl Pts',(46.3027202641352,1.47862733617782,138.943836932465));
#160819=CARTESIAN_POINT('Ctrl Pts',(46.1794352511173,2.97588016689551,139.130537365369));
#160820=CARTESIAN_POINT('Ctrl Pts',(46.0427961861896,3.9705349119133,139.342385458527));
#160821=CARTESIAN_POINT('Ctrl Pts',(45.9679913898148,4.43115774305712,139.460032410545));
#160822=CARTESIAN_POINT('Ctrl Pts',(46.5340727615371,-0.0378409420050605,
140.550116857512));
#160823=CARTESIAN_POINT('Ctrl Pts',(46.5348132498481,0.406438148398626,
140.548272721693));
#160824=CARTESIAN_POINT('Ctrl Pts',(46.5082651455313,1.34019173849624,140.582837843699));
#160825=CARTESIAN_POINT('Ctrl Pts',(46.3843580200113,2.69426001015636,140.751089543413));
#160826=CARTESIAN_POINT('Ctrl Pts',(46.2469931540946,3.5940664573222,140.942079807452));
#160827=CARTESIAN_POINT('Ctrl Pts',(46.1718065030185,4.01084563788002,141.048173637582));
#160828=CARTESIAN_POINT('Ctrl Pts',(47.8021843455376,-0.0344318706058168,
141.614201840284));
#160829=CARTESIAN_POINT('Ctrl Pts',(47.8030018749016,0.399310045394509,
141.612295274549));
#160830=CARTESIAN_POINT('Ctrl Pts',(47.7753793534869,1.31097231063154,141.647900621391));
#160831=CARTESIAN_POINT('Ctrl Pts',(47.6462983109395,2.62983125453292,141.820797693363));
#160832=CARTESIAN_POINT('Ctrl Pts',(47.5035770892202,3.50199158089965,142.015910523487));
#160833=CARTESIAN_POINT('Ctrl Pts',(47.4256304130497,3.90472204054626,142.123839733063));
#160834=CARTESIAN_POINT('Ctrl Pts',(49.4555224071342,-0.0369336755933763,
141.531364648942));
#160835=CARTESIAN_POINT('Ctrl Pts',(49.4563690431696,0.428409084164662,
141.529163521016));
#160836=CARTESIAN_POINT('Ctrl Pts',(49.4271957672958,1.40657748778552,141.570089986329));
#160837=CARTESIAN_POINT('Ctrl Pts',(49.2911528064204,2.81701045540398,141.768245070864));
#160838=CARTESIAN_POINT('Ctrl Pts',(49.1413059324474,3.74349484399151,141.990258669654));
#160839=CARTESIAN_POINT('Ctrl Pts',(49.0596954111229,4.16947605872563,142.112431337084));
#160840=CARTESIAN_POINT('Ctrl Pts',(46.0161346091238,8.04686257481308,146.026975529383));
#160841=CARTESIAN_POINT('Ctrl Pts',(46.0701379205231,7.99734211175707,146.230946628465));
#160842=CARTESIAN_POINT('Ctrl Pts',(46.1955438597492,7.87416261053135,146.687012632762));
#160843=CARTESIAN_POINT('Ctrl Pts',(46.3910983490287,7.65552025469006,147.34440254582));
#160844=CARTESIAN_POINT('Ctrl Pts',(46.5338233533296,7.47738131305873,147.790445316799));
#160845=CARTESIAN_POINT('Ctrl Pts',(46.6009706655345,7.38965660591495,147.993991853346));
#160846=CARTESIAN_POINT('Ctrl Pts',(46.339758162072,6.59170813014846,145.673040991343));
#160847=CARTESIAN_POINT('Ctrl Pts',(46.3933659254992,6.54808517167697,145.852403893947));
#160848=CARTESIAN_POINT('Ctrl Pts',(46.5178920837304,6.43959031579536,146.253430150673));
#160849=CARTESIAN_POINT('Ctrl Pts',(46.7122329313617,6.24706378925182,146.831420218524));
#160850=CARTESIAN_POINT('Ctrl Pts',(46.8542094315672,6.09023923413186,147.223539299679));
#160851=CARTESIAN_POINT('Ctrl Pts',(46.9210374701065,6.01301872846379,147.402466891096));
#160852=CARTESIAN_POINT('Ctrl Pts',(47.5243433476267,5.73410275588817,145.216152331719));
#160853=CARTESIAN_POINT('Ctrl Pts',(47.5765156814216,5.69878741311937,145.376200040928));
#160854=CARTESIAN_POINT('Ctrl Pts',(47.6978558665834,5.61027001230812,145.73476648539));
#160855=CARTESIAN_POINT('Ctrl Pts',(47.8878268680074,5.450892217511,146.254207184608));
#160856=CARTESIAN_POINT('Ctrl Pts',(48.0271307214227,5.31943503759318,146.608705840733));
#160857=CARTESIAN_POINT('Ctrl Pts',(48.0928248514571,5.25435476791681,146.770945110899));
#160858=CARTESIAN_POINT('Ctrl Pts',(49.0103064657029,5.87916884795805,144.872138221871));
#160859=CARTESIAN_POINT('Ctrl Pts',(49.0606815677909,5.85064681493126,145.027288004096));
#160860=CARTESIAN_POINT('Ctrl Pts',(49.1780346028805,5.77796257100624,145.376032072945));
#160861=CARTESIAN_POINT('Ctrl Pts',(49.3625438159987,5.64310735085286,145.885431893024));
#160862=CARTESIAN_POINT('Ctrl Pts',(49.4985134059075,5.52908729390024,146.236384822334));
#160863=CARTESIAN_POINT('Ctrl Pts',(49.5627946372691,5.47204839422951,146.397749756044));
#160864=CARTESIAN_POINT('',(49.3921071370737,5.47779704596669,146.36910776447));
#160865=CARTESIAN_POINT('Origin',(49.3876377743159,8.30858703474018,147.362326448108));
#160866=CARTESIAN_POINT('Ctrl Pts',(48.887434025587,5.85518895743199,144.97688956023));
#160867=CARTESIAN_POINT('Ctrl Pts',(48.9306897550823,5.82949635711896,145.108669038189));
#160868=CARTESIAN_POINT('Ctrl Pts',(48.9751043926647,5.80114206631471,145.239976811865));
#160869=CARTESIAN_POINT('Ctrl Pts',(49.0205765812721,5.77014957205661,145.370681194462));
#160870=CARTESIAN_POINT('Ctrl Pts',(49.0293081778864,5.76419837493542,145.395779127496));
#160871=CARTESIAN_POINT('Ctrl Pts',(49.0380787584918,5.75814991559219,145.420854810407));
#160872=CARTESIAN_POINT('Ctrl Pts',(49.0468875752625,5.75200433966445,145.445907535824));
#160873=CARTESIAN_POINT('Ctrl Pts',(49.101570725823,5.71385398843274,145.601429212747));
#160874=CARTESIAN_POINT('Ctrl Pts',(49.1577283395669,5.67196688856135,145.75606162316));
#160875=CARTESIAN_POINT('Ctrl Pts',(49.2153072140572,5.62627621912166,145.909943315272));
#160876=CARTESIAN_POINT('Ctrl Pts',(49.219843822728,5.62267627575719,145.922067571345));
#160877=CARTESIAN_POINT('Ctrl Pts',(49.2243892370016,5.61905269833621,145.93418714346));
#160878=CARTESIAN_POINT('Ctrl Pts',(49.2289433747957,5.61540548943111,145.946301935296));
#160879=CARTESIAN_POINT('Ctrl Pts',(49.2821898449036,5.57276273053368,146.087946727469));
#160880=CARTESIAN_POINT('Ctrl Pts',(49.3366294769991,5.52688881483523,146.228938194885));
#160881=CARTESIAN_POINT('Ctrl Pts',(49.3921048021131,5.47779893615921,146.369101802441));
#160882=CARTESIAN_POINT('Origin',(10.4447115478058,-4.01955337529683,143.058388065124));
#160883=CARTESIAN_POINT('',(47.0978472346802,3.75861943712466,149.414023271397));
#160884=CARTESIAN_POINT('Ctrl Pts',(49.3921071370737,5.47779704596669,146.36910776447));
#160885=CARTESIAN_POINT('Ctrl Pts',(49.4361507302258,5.43880070204039,146.48045098635));
#160886=CARTESIAN_POINT('Ctrl Pts',(49.4706982859556,5.39657329383826,146.594657875756));
#160887=CARTESIAN_POINT('Ctrl Pts',(49.4957503680475,5.35075653442217,146.711508385595));
#160888=CARTESIAN_POINT('Ctrl Pts',(49.5082764090935,5.32784815471413,146.769933640515));
#160889=CARTESIAN_POINT('Ctrl Pts',(49.5184285820122,5.30404225791503,146.829019263037));
#160890=CARTESIAN_POINT('Ctrl Pts',(49.5262069586772,5.27929316857397,146.888734263028));
#160891=CARTESIAN_POINT('Ctrl Pts',(49.5300961470098,5.26691862390344,146.918591763023));
#160892=CARTESIAN_POINT('Ctrl Pts',(49.5333918863107,5.25430826082335,146.948606598876));
#160893=CARTESIAN_POINT('Ctrl Pts',(49.5360941856033,5.24145634520237,146.978774621788));
#160894=CARTESIAN_POINT('Ctrl Pts',(49.5379370818315,5.23269168064885,146.999348410852));
#160895=CARTESIAN_POINT('Ctrl Pts',(49.5395474500292,5.22343650687812,147.020869714439));
#160896=CARTESIAN_POINT('Ctrl Pts',(49.5408363523507,5.21446088356659,147.041543643582));
#160897=CARTESIAN_POINT('Ctrl Pts',(49.5414374098535,5.21027525549866,147.051184576037));
#160898=CARTESIAN_POINT('Ctrl Pts',(49.5419685582334,5.20615113024434,147.060641537434));
#160899=CARTESIAN_POINT('Ctrl Pts',(49.5424207725859,5.20217013861614,147.069734049073));
#160900=CARTESIAN_POINT('Ctrl Pts',(49.5481085276126,5.15209896104572,147.184095697475));
#160901=CARTESIAN_POINT('Ctrl Pts',(49.5452460076019,5.10122031784624,147.294445737981));
#160902=CARTESIAN_POINT('Ctrl Pts',(49.5338326352621,5.04990109989827,147.400864052974));
#160903=CARTESIAN_POINT('Ctrl Pts',(49.5281259490923,5.02424149092427,147.454073210471));
#160904=CARTESIAN_POINT('Ctrl Pts',(49.5202815505016,4.99847131783018,147.506299708939));
#160905=CARTESIAN_POINT('Ctrl Pts',(49.5102993713006,4.97263391743248,147.557555018204));
#160906=CARTESIAN_POINT('Ctrl Pts',(49.5053082817001,4.95971521723364,147.583182672837));
#160907=CARTESIAN_POINT('Ctrl Pts',(49.4997827469708,4.9467796950444,147.608567522475));
#160908=CARTESIAN_POINT('Ctrl Pts',(49.4937227588561,4.93383259825042,147.633711106031));
#160909=CARTESIAN_POINT('Ctrl Pts',(49.4906927647988,4.92735904985344,147.646282897809));
#160910=CARTESIAN_POINT('Ctrl Pts',(49.4875291573966,4.9208826068105,147.658794372571));
#160911=CARTESIAN_POINT('Ctrl Pts',(49.4842319356302,4.91440391703237,147.671245723755));
#160912=CARTESIAN_POINT('Ctrl Pts',(49.4811025386957,4.90825498518383,147.683063315347));
#160913=CARTESIAN_POINT('Ctrl Pts',(49.4775545266859,4.90156201404105,147.695858784716));
#160914=CARTESIAN_POINT('Ctrl Pts',(49.4744371246675,4.89586880492085,147.70669375997));
#160915=CARTESIAN_POINT('Ctrl Pts',(49.4742699431049,4.895563486713,147.707274823331));
#160916=CARTESIAN_POINT('Ctrl Pts',(49.474103999966,4.89526105462038,147.707850253944));
#160917=CARTESIAN_POINT('Ctrl Pts',(49.4739394262268,4.89496175022421,147.70841960043));
#160918=CARTESIAN_POINT('Ctrl Pts',(49.448072640778,4.84791874909003,147.797906316196));
#160919=CARTESIAN_POINT('Ctrl Pts',(49.4139503782418,4.79914848496446,147.887360904827));
#160920=CARTESIAN_POINT('Ctrl Pts',(49.3715727001156,4.7486118832405,147.976707891572));
#160921=CARTESIAN_POINT('Ctrl Pts',(49.3503838610525,4.72334358237852,148.021381384944));
#160922=CARTESIAN_POINT('Ctrl Pts',(49.3271311680859,4.69763370090939,148.066027980018));
#160923=CARTESIAN_POINT('Ctrl Pts',(49.3018146284735,4.67147762747258,148.11063783537));
#160924=CARTESIAN_POINT('Ctrl Pts',(49.2891563586674,4.65839959075418,148.132942763046));
#160925=CARTESIAN_POINT('Ctrl Pts',(49.2759821271991,4.64521000649151,148.155238506045));
#160926=CARTESIAN_POINT('Ctrl Pts',(49.2622919349606,4.63190830800298,148.177523823348));
#160927=CARTESIAN_POINT('Ctrl Pts',(49.2554468388413,4.62525745875873,148.188666481999));
#160928=CARTESIAN_POINT('Ctrl Pts',(49.2484727525294,4.61857858098203,148.199806534241));
#160929=CARTESIAN_POINT('Ctrl Pts',(49.2413696761348,4.61187160489373,148.210943823517));
#160930=CARTESIAN_POINT('Ctrl Pts',(49.2346321898464,4.60550983192086,148.221507884724));
#160931=CARTESIAN_POINT('Ctrl Pts',(49.227059866239,4.59846277627678,148.233156671138));
#160932=CARTESIAN_POINT('Ctrl Pts',(49.2206980704094,4.59260844559814,148.242796270887));
#160933=CARTESIAN_POINT('Ctrl Pts',(49.2203528660537,4.59229077736359,148.243319335743));
#160934=CARTESIAN_POINT('Ctrl Pts',(49.2200112259285,4.59197663175015,148.243836491342));
#160935=CARTESIAN_POINT('Ctrl Pts',(49.2196734768118,4.59166631229651,148.244347245497));
#160936=CARTESIAN_POINT('Ctrl Pts',(49.1671762623241,4.54343256092357,148.323735078496));
#160937=CARTESIAN_POINT('Ctrl Pts',(49.1119271759838,4.49707551576149,148.397537522733));
#160938=CARTESIAN_POINT('Ctrl Pts',(49.0539255915381,4.45299316675182,148.465968084059));
#160939=CARTESIAN_POINT('Ctrl Pts',(49.0249247993152,4.43095199224698,148.500183364723));
#160940=CARTESIAN_POINT('Ctrl Pts',(48.9952358841048,4.40947851381734,148.53305551054));
#160941=CARTESIAN_POINT('Ctrl Pts',(48.9648587766526,4.38861674296047,148.564609948554));
#160942=CARTESIAN_POINT('Ctrl Pts',(48.9496702229265,4.37818585753203,148.580387167561));
#160943=CARTESIAN_POINT('Ctrl Pts',(48.9343096212152,4.36790785115326,148.595834927884));
#160944=CARTESIAN_POINT('Ctrl Pts',(48.918776963434,4.35778786171874,148.610956331161));
#160945=CARTESIAN_POINT('Ctrl Pts',(48.9049524615912,4.348780786783,148.62441480494));
#160946=CARTESIAN_POINT('Ctrl Pts',(48.8900288329631,4.3393055695298,148.638492995324));
#160947=CARTESIAN_POINT('Ctrl Pts',(48.8765769164015,4.33094975518149,148.650847922563));
#160948=CARTESIAN_POINT('Ctrl Pts',(48.8749147971136,4.32991731046401,148.652374497812));
#160949=CARTESIAN_POINT('Ctrl Pts',(48.8732751464897,4.32890201005717,148.653874800516));
#160950=CARTESIAN_POINT('Ctrl Pts',(48.8716628140952,4.32790689195046,148.655344440179));
#160951=CARTESIAN_POINT('Ctrl Pts',(48.7928437216884,4.27926040548347,148.727187978661));
#160952=CARTESIAN_POINT('Ctrl Pts',(48.7091012997476,4.23260602872896,148.794063467525));
#160953=CARTESIAN_POINT('Ctrl Pts',(48.6204350301956,4.18827300205104,148.856169581348));
#160954=CARTESIAN_POINT('Ctrl Pts',(48.5312371012076,4.14367414630336,148.918648094975));
#160955=CARTESIAN_POINT('Ctrl Pts',(48.4370560991793,4.10142442556188,148.976300218093));
#160956=CARTESIAN_POINT('Ctrl Pts',(48.3378915759401,4.06180865192953,149.029313001505));
#160957=CARTESIAN_POINT('Ctrl Pts',(48.3155991775574,4.05290294070131,149.041230389383));
#160958=CARTESIAN_POINT('Ctrl Pts',(48.2930549322134,4.04413014298943,149.052913251231));
#160959=CARTESIAN_POINT('Ctrl Pts',(48.2702588353468,4.03549315764655,149.064363580206));
#160960=CARTESIAN_POINT('Ctrl Pts',(48.2327585047276,4.02128503211499,149.08319974873));
#160961=CARTESIAN_POINT('Ctrl Pts',(48.1945766302123,4.00744447862358,149.101406673959));
#160962=CARTESIAN_POINT('Ctrl Pts',(48.1557131926094,3.99398369318984,149.118992912761));
#160963=CARTESIAN_POINT('Ctrl Pts',(48.136281473808,3.98725330047297,149.127786032162));
#160964=CARTESIAN_POINT('Ctrl Pts',(48.1166793642531,3.98061783810165,149.136423971038));
#160965=CARTESIAN_POINT('Ctrl Pts',(48.0969068616784,3.97407874625011,149.144907764067));
#160966=CARTESIAN_POINT('Ctrl Pts',(48.0771343591037,3.96753965439857,149.153391557096));
#160967=CARTESIAN_POINT('Ctrl Pts',(48.0552578353902,3.96048695014219,149.162507265567));
#160968=CARTESIAN_POINT('Ctrl Pts',(48.037078172702,3.95475197591698,149.169897704169));
#160969=CARTESIAN_POINT('Ctrl Pts',(47.9369529244939,3.92316636689794,149.210600852084));
#160970=CARTESIAN_POINT('Ctrl Pts',(47.8341972039513,3.89454764491787,149.246814174914));
#160971=CARTESIAN_POINT('Ctrl Pts',(47.7288107311118,3.86907372372077,149.278671429963));
#160972=CARTESIAN_POINT('Ctrl Pts',(47.6233303443575,3.84357710173865,149.310557074231));
#160973=CARTESIAN_POINT('Ctrl Pts',(47.5152145146778,3.82123076803661,149.33807905775));
#160974=CARTESIAN_POINT('Ctrl Pts',(47.4044630302007,3.80216936475247,149.361342960505));
#160975=CARTESIAN_POINT('Ctrl Pts',(47.3044088952034,3.78494907893479,149.382359831546));
#160976=CARTESIAN_POINT('Ctrl Pts',(47.2022036665947,3.77040919993785,149.399901165777));
#160977=CARTESIAN_POINT('Ctrl Pts',(47.0978472346802,3.75861943712466,149.414023271397));
#160978=CARTESIAN_POINT('',(38.9483300367407,2.68372196522192,150.519324999229));
#160979=CARTESIAN_POINT('Origin',(84.8264838120473,-2.60418696047202,144.299062259712));
#160980=CARTESIAN_POINT('',(10.4342334294899,2.6388562881557,150.519317696389));
#160981=CARTESIAN_POINT('Origin',(10.4384246768163,-0.0245075772277829,
147.534945843904));
#160982=CARTESIAN_POINT('Ctrl Pts',(38.9483300382364,2.68372101404257,150.519323933408));
#160983=CARTESIAN_POINT('Ctrl Pts',(38.6027432695898,2.64416611286694,150.554139247846));
#160984=CARTESIAN_POINT('Ctrl Pts',(38.266183212812,2.604090445613,150.588057906848));
#160985=CARTESIAN_POINT('Ctrl Pts',(37.9386436491546,2.56353408926601,150.621074225556));
#160986=CARTESIAN_POINT('Ctrl Pts',(37.8962911845616,2.55828995439867,150.625343396747));
#160987=CARTESIAN_POINT('Ctrl Pts',(37.8540895096113,2.55303784646761,150.629597485271));
#160988=CARTESIAN_POINT('Ctrl Pts',(37.8120385840336,2.54777790769498,150.633836482566));
#160989=CARTESIAN_POINT('Ctrl Pts',(37.5010385754246,2.50887648088693,150.665187235899));
#160990=CARTESIAN_POINT('Ctrl Pts',(37.1982862600139,2.46954281254957,150.695712266618));
#160991=CARTESIAN_POINT('Ctrl Pts',(36.9037811468005,2.42981074257045,150.725406929677));
#160992=CARTESIAN_POINT('Ctrl Pts',(36.8511029967784,2.42270386445818,150.730718416117));
#160993=CARTESIAN_POINT('Ctrl Pts',(36.7986886496763,2.4155843587941,150.73600334356));
#160994=CARTESIAN_POINT('Ctrl Pts',(36.7465380234107,2.4084525704991,150.741261695967));
#160995=CARTESIAN_POINT('Ctrl Pts',(36.4676886727713,2.37031890505036,150.769378101448));
#160996=CARTESIAN_POINT('Ctrl Pts',(36.1963813298171,2.33183026043562,150.796734448863));
#160997=CARTESIAN_POINT('Ctrl Pts',(35.9326187900983,2.29301640643672,150.823327121199));
#160998=CARTESIAN_POINT('Ctrl Pts',(35.8789578999625,2.28511996307746,150.828737239217));
#160999=CARTESIAN_POINT('Ctrl Pts',(35.8256092008524,2.27721021023271,150.834115759836));
#161000=CARTESIAN_POINT('Ctrl Pts',(35.7725725908774,2.2692876224765,150.839462668646));
#161001=CARTESIAN_POINT('Ctrl Pts',(35.5236784004087,2.23210790705111,150.864555044279));
#161002=CARTESIAN_POINT('Ctrl Pts',(35.2816596094678,2.19464180178193,150.888950959313));
#161003=CARTESIAN_POINT('Ctrl Pts',(35.0465224406967,2.15691561437506,150.912647574482));
#161004=CARTESIAN_POINT('Ctrl Pts',(34.9908865278496,2.14798920395007,150.918254441415));
#161005=CARTESIAN_POINT('Ctrl Pts',(34.9356357602717,2.13904843085661,150.923822172934));
#161006=CARTESIAN_POINT('Ctrl Pts',(34.8807700058312,2.13009399901494,150.929350757835));
#161007=CARTESIAN_POINT('Ctrl Pts',(34.7750750055704,2.11284391860519,150.940001186112));
#161008=CARTESIAN_POINT('Ctrl Pts',(34.6708089477046,2.09554298275572,150.950506323685));
#161009=CARTESIAN_POINT('Ctrl Pts',(34.5679736963875,2.07819246308016,150.960865825684));
#161010=CARTESIAN_POINT('Ctrl Pts',(34.3952114943478,2.04904376215035,150.978269686271));
#161011=CARTESIAN_POINT('Ctrl Pts',(34.2264863600537,2.01975324056144,150.995263064868));
#161012=CARTESIAN_POINT('Ctrl Pts',(34.0617918219847,1.99033795250279,151.011847298683));
#161013=CARTESIAN_POINT('Ctrl Pts',(33.8659875723369,1.95536631061334,151.031564184842));
#161014=CARTESIAN_POINT('Ctrl Pts',(33.6758817556065,1.92021657413703,151.050702627247));
#161015=CARTESIAN_POINT('Ctrl Pts',(33.4914778686697,1.88490334935071,151.069263352936));
#161016=CARTESIAN_POINT('Ctrl Pts',(33.4296932287429,1.87307163086409,151.075482135916));
#161017=CARTESIAN_POINT('Ctrl Pts',(33.3685484270922,1.86122192142731,151.081636090093));
#161018=CARTESIAN_POINT('Ctrl Pts',(33.3080428602635,1.84935581311173,151.087725315099));
#161019=CARTESIAN_POINT('Ctrl Pts',(33.151858337036,1.81872553284213,151.103443582925));
#161020=CARTESIAN_POINT('Ctrl Pts',(32.9999349343395,1.78798371775716,151.118730371713));
#161021=CARTESIAN_POINT('Ctrl Pts',(32.8522803581535,1.75713880684416,151.133585536884));
#161022=CARTESIAN_POINT('Ctrl Pts',(32.7725113616133,1.74047513372642,151.1416109002));
#161023=CARTESIAN_POINT('Ctrl Pts',(32.6939882630894,1.7237810339304,151.149510752151));
#161024=CARTESIAN_POINT('Ctrl Pts',(32.6167083927223,1.70706086971309,151.157285460588));
#161025=CARTESIAN_POINT('Ctrl Pts',(32.4691175929587,1.6751283315594,151.172133770124));
#161026=CARTESIAN_POINT('Ctrl Pts',(32.326063748158,1.64309795647864,151.186525396057));
#161027=CARTESIAN_POINT('Ctrl Pts',(32.1875518770369,1.61097868776279,151.20046042161));
#161028=CARTESIAN_POINT('Ctrl Pts',(32.1625711175385,1.60518594436424,151.202973617909));
#161029=CARTESIAN_POINT('Ctrl Pts',(32.1377380044198,1.59939041388421,151.20547197116));
#161030=CARTESIAN_POINT('Ctrl Pts',(32.1130524542536,1.59359228214992,151.207955492803));
#161031=CARTESIAN_POINT('Ctrl Pts',(32.0701298266207,1.58351063326134,151.212273779167));
#161032=CARTESIAN_POINT('Ctrl Pts',(32.027654141952,1.5734204157536,151.216547519342));
#161033=CARTESIAN_POINT('Ctrl Pts',(31.9856243973538,1.56332289564894,151.220776766451));
#161034=CARTESIAN_POINT('Ctrl Pts',(31.9134652058033,1.54598686626355,151.228037792069));
#161035=CARTESIAN_POINT('Ctrl Pts',(31.8426207416885,1.52862903156681,151.235167641275));
#161036=CARTESIAN_POINT('Ctrl Pts',(31.7730929017198,1.51124959459354,151.242165893124));
#161037=CARTESIAN_POINT('Ctrl Pts',(31.7180804361685,1.49749847449226,151.247703115177));
#161038=CARTESIAN_POINT('Ctrl Pts',(31.6638916996835,1.48373423685283,151.253157836866));
#161039=CARTESIAN_POINT('Ctrl Pts',(31.6105266905512,1.4699579771998,151.258530350681));
#161040=CARTESIAN_POINT('Ctrl Pts',(31.583844185985,1.46306984737328,151.261216607589));
#161041=CARTESIAN_POINT('Ctrl Pts',(31.5573676132506,1.45617871594911,151.263882322376));
#161042=CARTESIAN_POINT('Ctrl Pts',(31.5310969721014,1.4492847387293,151.266527586375));
#161043=CARTESIAN_POINT('Ctrl Pts',(31.5179616515267,1.4458377501194,151.267850218375));
#161044=CARTESIAN_POINT('Ctrl Pts',(31.5048778138481,1.44239005024169,151.269167738205));
#161045=CARTESIAN_POINT('Ctrl Pts',(31.491845459033,1.43894165948415,151.270480160329));
#161046=CARTESIAN_POINT('Ctrl Pts',(31.478813104218,1.43549326872661,151.271792582453));
#161047=CARTESIAN_POINT('Ctrl Pts',(31.4671055638423,1.43238393073357,151.272971657411));
#161048=CARTESIAN_POINT('Ctrl Pts',(31.4529028431458,1.4285944355183,151.274402149949));
#161049=CARTESIAN_POINT('Ctrl Pts',(31.439419072415,1.42499676675048,151.275760230125));
#161050=CARTESIAN_POINT('Ctrl Pts',(31.4259888429677,1.42139781441521,151.277112993081));
#161051=CARTESIAN_POINT('Ctrl Pts',(31.4126120387662,1.41779762190945,151.278460446859));
#161052=CARTESIAN_POINT('Ctrl Pts',(31.3021595831912,1.38807078306107,151.28958639117));
#161053=CARTESIAN_POINT('Ctrl Pts',(31.1953530398958,1.35825622082807,151.300349992595));
#161054=CARTESIAN_POINT('Ctrl Pts',(31.0921689282748,1.32834578422234,151.310751710281));
#161055=CARTESIAN_POINT('Ctrl Pts',(31.0250589479275,1.30889231622949,151.3175168901));
#161056=CARTESIAN_POINT('Ctrl Pts',(30.9594803861762,1.28939911894315,151.324129086344));
#161057=CARTESIAN_POINT('Ctrl Pts',(30.8954181725188,1.26987173470207,151.330589355687));
#161058=CARTESIAN_POINT('Ctrl Pts',(30.8033863044817,1.24181866648935,151.339870187893));
#161059=CARTESIAN_POINT('Ctrl Pts',(30.7144866277601,1.21369299570105,151.348837186809));
#161060=CARTESIAN_POINT('Ctrl Pts',(30.6287161567598,1.18548510478732,151.357489458271));
#161061=CARTESIAN_POINT('Ctrl Pts',(30.5609497064191,1.16319831288184,151.364325537372));
#161062=CARTESIAN_POINT('Ctrl Pts',(30.495135598263,1.14086103694648,151.37096525925));
#161063=CARTESIAN_POINT('Ctrl Pts',(30.4312544687237,1.11848251767363,151.377410080749));
#161064=CARTESIAN_POINT('Ctrl Pts',(30.3562068564538,1.09219221176209,151.384981463229));
#161065=CARTESIAN_POINT('Ctrl Pts',(30.2838295069765,1.06584353282845,151.39228360202));
#161066=CARTESIAN_POINT('Ctrl Pts',(30.2141395724523,1.03942730195697,151.399314111018));
#161067=CARTESIAN_POINT('Ctrl Pts',(30.1460731455833,1.01362646774687,151.406180836174));
#161068=CARTESIAN_POINT('Ctrl Pts',(30.0805696770538,0.987761702529661,
151.412788511418));
#161069=CARTESIAN_POINT('Ctrl Pts',(30.0176051661593,0.961850531843709,
151.419139091241));
#161070=CARTESIAN_POINT('Ctrl Pts',(29.9598133948294,0.938068048189028,
151.424967950255));
#161071=CARTESIAN_POINT('Ctrl Pts',(29.9041620617812,0.914245962732354,
151.43058007034));
#161072=CARTESIAN_POINT('Ctrl Pts',(29.8506854606712,0.890378792179376,
151.435971744736));
#161073=CARTESIAN_POINT('Ctrl Pts',(29.7942287314613,0.865181559054073,
151.441663884757));
#161074=CARTESIAN_POINT('Ctrl Pts',(29.7401956613144,0.839934242751313,
151.447110345417));
#161075=CARTESIAN_POINT('Ctrl Pts',(29.6885754213258,0.814656693484691,
151.452312044106));
#161076=CARTESIAN_POINT('Ctrl Pts',(29.6775138468789,0.809240029534481,
151.453426703342));
#161077=CARTESIAN_POINT('Ctrl Pts',(29.6665628971776,0.803822062990689,
151.454530140923));
#161078=CARTESIAN_POINT('Ctrl Pts',(29.6557221979594,0.798403122736736,
151.45562239356));
#161079=CARTESIAN_POINT('Ctrl Pts',(29.6113559591719,0.776225771216936,
151.460092505708));
#161080=CARTESIAN_POINT('Ctrl Pts',(29.5688406215529,0.754030554791447,
151.464374841223));
#161081=CARTESIAN_POINT('Ctrl Pts',(29.5282257151081,0.731821673711811,
151.46846439376));
#161082=CARTESIAN_POINT('Ctrl Pts',(29.4993439715204,0.716028673927752,
151.471372523265));
#161083=CARTESIAN_POINT('Ctrl Pts',(29.4714220361072,0.700229209359056,
151.474183288859));
#161084=CARTESIAN_POINT('Ctrl Pts',(29.444462864748,0.684430100848601,151.476896405429));
#161085=CARTESIAN_POINT('Ctrl Pts',(29.4120388866724,0.66542840598453,151.480159489113));
#161086=CARTESIAN_POINT('Ctrl Pts',(29.381008471491,0.646424010729459,151.483281922171));
#161087=CARTESIAN_POINT('Ctrl Pts',(29.3513265884524,0.627415074671382,
151.486268046272));
#161088=CARTESIAN_POINT('Ctrl Pts',(29.3173570323049,0.605660217680324,
151.489685528586));
#161089=CARTESIAN_POINT('Ctrl Pts',(29.2851569519863,0.583899258394271,
151.492924153563));
#161090=CARTESIAN_POINT('Ctrl Pts',(29.2547537739581,0.562122696882355,
151.495980991589));
#161091=CARTESIAN_POINT('Ctrl Pts',(29.2208105338232,0.537810532672966,
151.499393759396));
#161092=CARTESIAN_POINT('Ctrl Pts',(29.1891065944066,0.513479201977103,
151.502579983994));
#161093=CARTESIAN_POINT('Ctrl Pts',(29.1596123629576,0.489119825777804,
151.505542526122));
#161094=CARTESIAN_POINT('Ctrl Pts',(29.1424940405993,0.474981750847837,
151.507261972558));
#161095=CARTESIAN_POINT('Ctrl Pts',(29.1261188929719,0.460834281051649,
151.508906190981));
#161096=CARTESIAN_POINT('Ctrl Pts',(29.1104734441162,0.446675643663467,
151.510476529098));
#161097=CARTESIAN_POINT('Ctrl Pts',(29.0866568282643,0.425122358054861,
151.512867009551));
#161098=CARTESIAN_POINT('Ctrl Pts',(29.0645346973072,0.403544304906276,
151.515085931265));
#161099=CARTESIAN_POINT('Ctrl Pts',(29.0441608765425,0.381969017990187,
151.517127919829));
#161100=CARTESIAN_POINT('Ctrl Pts',(29.0215281089998,0.358001571771817,
151.519396313815));
#161101=CARTESIAN_POINT('Ctrl Pts',(29.0010521035118,0.334037774725908,
151.521446442291));
#161102=CARTESIAN_POINT('Ctrl Pts',(28.9827472026584,0.310095949764079,
151.523276883032));
#161103=CARTESIAN_POINT('Ctrl Pts',(28.9815204766048,0.308491458120782,
151.523399552331));
#161104=CARTESIAN_POINT('Ctrl Pts',(28.9803034841381,0.306887057857641,
151.523521236678));
#161105=CARTESIAN_POINT('Ctrl Pts',(28.9790962226575,0.305282751370811,
151.523641936329));
#161106=CARTESIAN_POINT('Ctrl Pts',(28.9672218773354,0.2895031629932,151.524829110244));
#161107=CARTESIAN_POINT('Ctrl Pts',(28.9562872886384,0.273736664172069,
151.525920784737));
#161108=CARTESIAN_POINT('Ctrl Pts',(28.9462822664861,0.257961851789511,
151.526918758088));
#161109=CARTESIAN_POINT('Ctrl Pts',(28.9312208536328,0.234214681782191,
151.52842109246));
#161110=CARTESIAN_POINT('Ctrl Pts',(28.9182635854512,0.210451660595227,
151.52971135097));
#161111=CARTESIAN_POINT('Ctrl Pts',(28.907399609783,0.186702762534852,151.530792636163));
#161112=CARTESIAN_POINT('Ctrl Pts',(28.8972468659891,0.164508633538344,
151.53180313286));
#161113=CARTESIAN_POINT('Ctrl Pts',(28.8889215340135,0.142325550128787,
151.532631170926));
#161114=CARTESIAN_POINT('Ctrl Pts',(28.882455295068,0.120150967013752,151.533274861738));
#161115=CARTESIAN_POINT('Ctrl Pts',(28.8820023145399,0.118597567200818,
151.533319954319));
#161116=CARTESIAN_POINT('Ctrl Pts',(28.8815584774549,0.117044201652551,
151.533364140163));
#161117=CARTESIAN_POINT('Ctrl Pts',(28.8811238041125,0.115490866386377,
151.533407417661));
#161118=CARTESIAN_POINT('Ctrl Pts',(28.8771341750942,0.101233651028576,
151.533804638168));
#161119=CARTESIAN_POINT('Ctrl Pts',(28.8738776244795,0.0869157802293588,
151.53412704013));
#161120=CARTESIAN_POINT('Ctrl Pts',(28.871403161365,0.0725743470340143,
151.534370489789));
#161121=CARTESIAN_POINT('Ctrl Pts',(28.8671330035289,0.0478254700020986,
151.534790608588));
#161122=CARTESIAN_POINT('Ctrl Pts',(28.8651944694018,0.0230063130007055,
151.534975330761));
#161123=CARTESIAN_POINT('Ctrl Pts',(28.8655113019717,-0.00161249851495384,
151.534936134653));
#161124=CARTESIAN_POINT('Ctrl Pts',(28.8658249293817,-0.0259822597976901,
151.534897335062));
#161125=CARTESIAN_POINT('Ctrl Pts',(28.8683484094705,-0.0501548456514469,
151.534639070795));
#161126=CARTESIAN_POINT('Ctrl Pts',(28.8729577422789,-0.0738687071900575,
151.534178059856));
#161127=CARTESIAN_POINT('Ctrl Pts',(28.8749169270865,-0.0839482217723661,
151.533982108367));
#161128=CARTESIAN_POINT('Ctrl Pts',(28.8772876173455,-0.0940506262770279,
151.533747584978));
#161129=CARTESIAN_POINT('Ctrl Pts',(28.8800798808754,-0.104168181396869,
151.533473267271));
#161130=CARTESIAN_POINT('Ctrl Pts',(28.8872124503321,-0.130012505849106,
151.532772548992));
#161131=CARTESIAN_POINT('Ctrl Pts',(28.8970928942548,-0.155956749588127,
151.531812409961));
#161132=CARTESIAN_POINT('Ctrl Pts',(28.9096719124097,-0.181976415511025,
151.53059540908));
#161133=CARTESIAN_POINT('Ctrl Pts',(28.9226734556467,-0.208870073453178,
151.529337529541));
#161134=CARTESIAN_POINT('Ctrl Pts',(28.9385601618265,-0.235846111339722,
151.527805178816));
#161135=CARTESIAN_POINT('Ctrl Pts',(28.9573154776245,-0.262844139658197,
151.525996998897));
#161136=CARTESIAN_POINT('Ctrl Pts',(28.9612710740981,-0.26853816831437,
151.525615644076));
#161137=CARTESIAN_POINT('Ctrl Pts',(28.9653543226671,-0.274233000755657,
151.525222008365));
#161138=CARTESIAN_POINT('Ctrl Pts',(28.9695651013876,-0.279927757494856,
151.524816062986));
#161139=CARTESIAN_POINT('Ctrl Pts',(28.990216475843,-0.307857164776068,
151.52282514145));
#161140=CARTESIAN_POINT('Ctrl Pts',(29.0139372600631,-0.335786096141674,
151.520538260894));
#161141=CARTESIAN_POINT('Ctrl Pts',(29.0407751906054,-0.363792963429348,
151.517943728282));
#161142=CARTESIAN_POINT('Ctrl Pts',(29.0625868467577,-0.386554634945706,
151.515835106192));
#161143=CARTESIAN_POINT('Ctrl Pts',(29.0864588872605,-0.409367699882497,
151.513523097419));
#161144=CARTESIAN_POINT('Ctrl Pts',(29.1123853322711,-0.432261641585833,
151.511002129416));
#161145=CARTESIAN_POINT('Ctrl Pts',(29.1183598179163,-0.437537317676879,
151.510421197971));
#161146=CARTESIAN_POINT('Ctrl Pts',(29.1244431952512,-0.442817229452095,
151.509829179544));
#161147=CARTESIAN_POINT('Ctrl Pts',(29.1306349724997,-0.448101625097921,
151.509226027365));
#161148=CARTESIAN_POINT('Ctrl Pts',(29.1337229685925,-0.45073708701009,
151.508925220102));
#161149=CARTESIAN_POINT('Ctrl Pts',(29.1368377473778,-0.453373191351228,
151.508621698255));
#161150=CARTESIAN_POINT('Ctrl Pts',(29.1399791681834,-0.456009862426074,
151.508315472268));
#161151=CARTESIAN_POINT('Ctrl Pts',(29.1672013400079,-0.478858094956928,
151.505661852472));
#161152=CARTESIAN_POINT('Ctrl Pts',(29.1964280103261,-0.501748584700058,
151.502804832625));
#161153=CARTESIAN_POINT('Ctrl Pts',(29.2277046042288,-0.524673176442512,
151.499737506279));
#161154=CARTESIAN_POINT('Ctrl Pts',(29.2563950096037,-0.545702187216171,
151.496923809986));
#161155=CARTESIAN_POINT('Ctrl Pts',(29.2868105924331,-0.566759770075305,
151.493933117712));
#161156=CARTESIAN_POINT('Ctrl Pts',(29.3189434761364,-0.587843653853886,
151.490763942473));
#161157=CARTESIAN_POINT('Ctrl Pts',(29.3386384193971,-0.600766424762658,
151.488821486044));
#161158=CARTESIAN_POINT('Ctrl Pts',(29.3589776579053,-0.613699159231986,
151.486812054609));
#161159=CARTESIAN_POINT('Ctrl Pts',(29.3799496193799,-0.626642513105162,
151.484736204012));
#161160=CARTESIAN_POINT('Ctrl Pts',(29.3862074017992,-0.630504655061366,
151.484116795026));
#161161=CARTESIAN_POINT('Ctrl Pts',(29.3925214591309,-0.634367750309721,
151.483491477977));
#161162=CARTESIAN_POINT('Ctrl Pts',(29.3988921040743,-0.638231764678178,
151.482860205853));
#161163=CARTESIAN_POINT('Ctrl Pts',(29.4373542694222,-0.661560385385414,
151.479048960207));
#161164=CARTESIAN_POINT('Ctrl Pts',(29.4778950245336,-0.684920994007202,
151.475020427045));
#161165=CARTESIAN_POINT('Ctrl Pts',(29.5205233412297,-0.708305371768688,
151.470767695467));
#161166=CARTESIAN_POINT('Ctrl Pts',(29.5360317789473,-0.716812748887632,
151.469220526169));
#161167=CARTESIAN_POINT('Ctrl Pts',(29.5518160652932,-0.725323430418557,
151.467643717436));
#161168=CARTESIAN_POINT('Ctrl Pts',(29.5678749735161,-0.733837605108871,
151.466037065843));
#161169=CARTESIAN_POINT('Ctrl Pts',(29.5979751299764,-0.749796223637019,
151.463025624238));
#161170=CARTESIAN_POINT('Ctrl Pts',(29.6290434575462,-0.765765969075537,
151.459909415387));
#161171=CARTESIAN_POINT('Ctrl Pts',(29.6610799505251,-0.781745744866384,
151.456689214732));
#161172=CARTESIAN_POINT('Ctrl Pts',(29.6694450062028,-0.785918227612744,
151.455848387436));
#161173=CARTESIAN_POINT('Ctrl Pts',(29.6778762175432,-0.790091360891029,
151.455000490086));
#161174=CARTESIAN_POINT('Ctrl Pts',(29.6863732835912,-0.794265205577799,
151.454145548124));
#161175=CARTESIAN_POINT('Ctrl Pts',(29.6941472507123,-0.798083856766365,
151.453363361582));
#161176=CARTESIAN_POINT('Ctrl Pts',(29.7019763378513,-0.801903104352659,
151.452575278723));
#161177=CARTESIAN_POINT('Ctrl Pts',(29.7098608132034,-0.805722856972097,
151.451781269757));
#161178=CARTESIAN_POINT('Ctrl Pts',(29.7206924334612,-0.810970398248478,
151.450690467489));
#161179=CARTESIAN_POINT('Ctrl Pts',(29.7323703843149,-0.816574297045414,
151.449513602825));
#161180=CARTESIAN_POINT('Ctrl Pts',(29.743435278034,-0.821833182059346,
151.448397796475));
#161181=CARTESIAN_POINT('Ctrl Pts',(29.7492281126836,-0.824586380788653,
151.447813635267));
#161182=CARTESIAN_POINT('Ctrl Pts',(29.7548521918546,-0.827245655506408,
151.447246286198));
#161183=CARTESIAN_POINT('Ctrl Pts',(29.7600939225384,-0.829714105783301,
151.446717305305));
#161184=CARTESIAN_POINT('Ctrl Pts',(29.8143646576473,-0.855271430107522,
151.441240453552));
#161185=CARTESIAN_POINT('Ctrl Pts',(29.8707617826373,-0.880693965368612,
151.435527365135));
#161186=CARTESIAN_POINT('Ctrl Pts',(29.9292810232518,-0.905979619620407,
151.429581190326));
#161187=CARTESIAN_POINT('Ctrl Pts',(29.9694586888553,-0.923340039038501,
151.425498713852));
#161188=CARTESIAN_POINT('Ctrl Pts',(30.0106358156893,-0.940636223409451,
151.421306488752));
#161189=CARTESIAN_POINT('Ctrl Pts',(30.052797859214,-0.957873000490626,
151.417007349118));
#161190=CARTESIAN_POINT('Ctrl Pts',(30.1206046968499,-0.985593937314419,
151.410093285217));
#161191=CARTESIAN_POINT('Ctrl Pts',(30.1909599125678,-1.0131606071397,151.402902463072));
#161192=CARTESIAN_POINT('Ctrl Pts',(30.2638971683645,-1.04055242161206,
151.395439389664));
#161193=CARTESIAN_POINT('Ctrl Pts',(30.3293256421008,-1.06512428950344,
151.388744628569));
#161194=CARTESIAN_POINT('Ctrl Pts',(30.3968316209166,-1.08955541881358,
151.381830849012));
#161195=CARTESIAN_POINT('Ctrl Pts',(30.4664085226188,-1.11384839667623,
151.3747062175));
#161196=CARTESIAN_POINT('Ctrl Pts',(30.5166960397161,-1.13140642972634,
151.369556806988));
#161197=CARTESIAN_POINT('Ctrl Pts',(30.5680643958423,-1.14889286986701,
151.364297384591));
#161198=CARTESIAN_POINT('Ctrl Pts',(30.6205264720779,-1.16630003090646,
151.3589300352));
#161199=CARTESIAN_POINT('Ctrl Pts',(30.702058863791,-1.19335285790684,151.350588527115));
#161200=CARTESIAN_POINT('Ctrl Pts',(30.7863430129809,-1.22025950416132,
151.341971502953));
#161201=CARTESIAN_POINT('Ctrl Pts',(30.8732745922089,-1.24698870044844,
151.333095615084));
#161202=CARTESIAN_POINT('Ctrl Pts',(30.8865931759859,-1.25108381804783,
151.331735761078));
#161203=CARTESIAN_POINT('Ctrl Pts',(30.8999738278721,-1.25517483667929,
151.330369840169));
#161204=CARTESIAN_POINT('Ctrl Pts',(30.9134160915004,-1.25926171694156,
151.328997922409));
#161205=CARTESIAN_POINT('Ctrl Pts',(31.0091841405266,-1.28837828243565,
151.319223832948));
#161206=CARTESIAN_POINT('Ctrl Pts',(31.1080822474525,-1.31728187204803,
151.309144968042));
#161207=CARTESIAN_POINT('Ctrl Pts',(31.2100003455261,-1.34592513978652,
151.29878187842));
#161208=CARTESIAN_POINT('Ctrl Pts',(31.2667389223497,-1.36187106379585,
151.293012667968));
#161209=CARTESIAN_POINT('Ctrl Pts',(31.3244128435392,-1.37773694793607,
151.287155455917));
#161210=CARTESIAN_POINT('Ctrl Pts',(31.3829982596841,-1.39351968941024,
151.281214450372));
#161211=CARTESIAN_POINT('Ctrl Pts',(31.4976982021994,-1.42441952180784,
151.269583006246));
#161212=CARTESIAN_POINT('Ctrl Pts',(31.6158937177216,-1.45499843725536,
151.257630094014));
#161213=CARTESIAN_POINT('Ctrl Pts',(31.7374418502422,-1.4852127666234,151.245384988212));
#161214=CARTESIAN_POINT('Ctrl Pts',(31.7826800930041,-1.49645804977578,
151.240827558513));
#161215=CARTESIAN_POINT('Ctrl Pts',(31.8284876727297,-1.50769531262186,
151.236212699029));
#161216=CARTESIAN_POINT('Ctrl Pts',(31.8748630728464,-1.51892424780116,
151.23154056007));
#161217=CARTESIAN_POINT('Ctrl Pts',(32.0044790319385,-1.55030832641151,
151.218482262553));
#161218=CARTESIAN_POINT('Ctrl Pts',(32.1385327792507,-1.58162478851494,
151.204976297435));
#161219=CARTESIAN_POINT('Ctrl Pts',(32.2770208022029,-1.61284339901664,
151.191022982071));
#161220=CARTESIAN_POINT('Ctrl Pts',(32.3247593551313,-1.62360484436055,
151.186213099817));
#161221=CARTESIAN_POINT('Ctrl Pts',(32.3730245291577,-1.63435499617135,
151.181350089714));
#161222=CARTESIAN_POINT('Ctrl Pts',(32.4218152223614,-1.64509372619346,
151.17643406181));
#161223=CARTESIAN_POINT('Ctrl Pts',(32.5709422999114,-1.67791628557194,
151.161408391414));
#161224=CARTESIAN_POINT('Ctrl Pts',(32.7249809288133,-1.71062936617794,
151.145887210082));
#161225=CARTESIAN_POINT('Ctrl Pts',(32.8839286591928,-1.7432042703979,151.129870758828));
#161226=CARTESIAN_POINT('Ctrl Pts',(32.9304179121803,-1.75273182363638,
151.125186244916));
#161227=CARTESIAN_POINT('Ctrl Pts',(32.9773269097341,-1.76224781831153,
151.12045938391));
#161228=CARTESIAN_POINT('Ctrl Pts',(33.024655057861,-1.77175221467368,151.115690235925));
#161229=CARTESIAN_POINT('Ctrl Pts',(33.1946925415478,-1.80589899001445,
151.098555952104));
#161230=CARTESIAN_POINT('Ctrl Pts',(33.3701424850901,-1.83989303878119,
151.080875617481));
#161231=CARTESIAN_POINT('Ctrl Pts',(33.5510039379001,-1.87370666177705,
151.06264936611));
#161232=CARTESIAN_POINT('Ctrl Pts',(33.5950739705717,-1.8819459380132,151.058208223562));
#161233=CARTESIAN_POINT('Ctrl Pts',(33.6394651643436,-1.89017469593504,
151.053734682196));
#161234=CARTESIAN_POINT('Ctrl Pts',(33.6841772240993,-1.8983929244592,151.049228772592));
#161235=CARTESIAN_POINT('Ctrl Pts',(33.8766766519041,-1.9337749734436,151.029829419818));
#161236=CARTESIAN_POINT('Ctrl Pts',(34.0751257124915,-1.96895863336787,
151.009829878581));
#161237=CARTESIAN_POINT('Ctrl Pts',(34.2795258855267,-2.00391606867805,
150.989230097083));
#161238=CARTESIAN_POINT('Ctrl Pts',(34.3233213711462,-2.01140616926206,
150.984816316895));
#161239=CARTESIAN_POINT('Ctrl Pts',(34.3673899602217,-2.01888604109792,
150.980374991118));
#161240=CARTESIAN_POINT('Ctrl Pts',(34.4117314899297,-2.0263556759316,150.975906137351));
#161241=CARTESIAN_POINT('Ctrl Pts',(34.6286104488291,-2.06289042420837,
150.95404851632));
#161242=CARTESIAN_POINT('Ctrl Pts',(34.8520210191477,-2.0991769182693,150.931532132542));
#161243=CARTESIAN_POINT('Ctrl Pts',(35.081967912608,-2.13518612187403,150.908356685189));
#161244=CARTESIAN_POINT('Ctrl Pts',(35.1270713875043,-2.14224923190949,
150.903810882495));
#161245=CARTESIAN_POINT('Ctrl Pts',(35.1724262550042,-2.14930180934974,
150.899239731789));
#161246=CARTESIAN_POINT('Ctrl Pts',(35.2180324233533,-2.15634384026042,
150.894643243842));
#161247=CARTESIAN_POINT('Ctrl Pts',(35.461479387331,-2.19393439231738,150.870107066476));
#161248=CARTESIAN_POINT('Ctrl Pts',(35.7120890568306,-2.23122096837176,
150.844848709685));
#161249=CARTESIAN_POINT('Ctrl Pts',(35.9698699703844,-2.26817242434974,
150.818867584338));
#161250=CARTESIAN_POINT('Ctrl Pts',(36.0165517626946,-2.27486399887224,
150.814162637487));
#161251=CARTESIAN_POINT('Ctrl Pts',(36.0634686593668,-2.28154470235949,
150.809433995305));
#161252=CARTESIAN_POINT('Ctrl Pts',(36.1106206170988,-2.28821451234414,
150.804681663958));
#161253=CARTESIAN_POINT('Ctrl Pts',(36.3830005854587,-2.32674361526947,
150.777229148215));
#161254=CARTESIAN_POINT('Ctrl Pts',(36.6632263673471,-2.36490566108977,
150.748985935835));
#161255=CARTESIAN_POINT('Ctrl Pts',(36.9513109655905,-2.4026665443615,150.719951108414));
#161256=CARTESIAN_POINT('Ctrl Pts',(36.999531099742,-2.40898703101072,150.715091205171));
#161257=CARTESIAN_POINT('Ctrl Pts',(37.0479713555632,-2.41529638232405,
150.710209129317));
#161258=CARTESIAN_POINT('Ctrl Pts',(37.0966317243219,-2.42159456730874,
150.70530488374));
#161259=CARTESIAN_POINT('Ctrl Pts',(37.4004415492397,-2.4609171315701,150.674685346159));
#161260=CARTESIAN_POINT('Ctrl Pts',(37.7128334435774,-2.49980080752529,
150.643201418644));
#161261=CARTESIAN_POINT('Ctrl Pts',(38.0338250764396,-2.53820730959646,
150.610851858719));
#161262=CARTESIAN_POINT('Ctrl Pts',(38.0870104466146,-2.54457091481435,
150.605491833274));
#161263=CARTESIAN_POINT('Ctrl Pts',(38.1404318565342,-2.55092152317193,
150.600108048707));
#161264=CARTESIAN_POINT('Ctrl Pts',(38.1940893220794,-2.55725908700571,
150.594700506049));
#161265=CARTESIAN_POINT('Ctrl Pts',(38.443204417394,-2.58668244501321,150.569594950076));
#161266=CARTESIAN_POINT('Ctrl Pts',(38.6974080777621,-2.61582361277085,
150.543977247674));
#161267=CARTESIAN_POINT('Ctrl Pts',(38.9567113549366,-2.64466260229147,
150.51784656602));
#161268=CARTESIAN_POINT('Ctrl Pts',(38.6142630337744,4.84795799788072,149.772399489946));
#161269=CARTESIAN_POINT('Ctrl Pts',(38.5518738101667,4.84248449990793,149.78368599245));
#161270=CARTESIAN_POINT('Ctrl Pts',(38.0917828938735,4.80166457174124,149.867090324444));
#161271=CARTESIAN_POINT('Ctrl Pts',(37.2666569365713,4.72231206624815,150.018981574206));
#161272=CARTESIAN_POINT('Ctrl Pts',(36.1675657918577,4.60062603149948,150.227154665666));
#161273=CARTESIAN_POINT('Ctrl Pts',(35.1567210374423,4.47267283862507,150.424283081802));
#161274=CARTESIAN_POINT('Ctrl Pts',(34.2242365051105,4.33830124550419,150.611670270562));
#161275=CARTESIAN_POINT('Ctrl Pts',(33.3605599489944,4.19687721453315,150.790698750079));
#161276=CARTESIAN_POINT('Ctrl Pts',(32.55812194511,4.04747828476444,150.962481754923));
#161277=CARTESIAN_POINT('Ctrl Pts',(31.811522135749,3.88898829657608,151.127760878239));
#161278=CARTESIAN_POINT('Ctrl Pts',(31.1168905319017,3.72004699986921,151.286968739904));
#161279=CARTESIAN_POINT('Ctrl Pts',(30.4700694589394,3.53852193518461,151.440596316724));
#161280=CARTESIAN_POINT('Ctrl Pts',(29.8659802889208,3.34090700461296,151.589333187113));
#161281=CARTESIAN_POINT('Ctrl Pts',(29.2983389023891,3.12136266852428,151.734134145579));
#161282=CARTESIAN_POINT('Ctrl Pts',(28.7606569834451,2.87046298671187,151.875930325475));
#161283=CARTESIAN_POINT('Ctrl Pts',(28.2482144210855,2.5734713359096,152.014964503663));
#161284=CARTESIAN_POINT('Ctrl Pts',(27.7590506808759,2.20617884390867,152.150266879811));
#161285=CARTESIAN_POINT('Ctrl Pts',(27.3022338120033,1.73160085833134,152.277303811874));
#161286=CARTESIAN_POINT('Ctrl Pts',(26.9178210953592,1.10518640460507,152.382971972441));
#161287=CARTESIAN_POINT('Ctrl Pts',(26.7013701547781,0.32781599167213,152.441378793244));
#161288=CARTESIAN_POINT('Ctrl Pts',(26.7294258532341,-0.486044842906302,
152.433991979976));
#161289=CARTESIAN_POINT('Ctrl Pts',(26.9753196545374,-1.20956093171679,
152.367647432518));
#161290=CARTESIAN_POINT('Ctrl Pts',(27.3563514766538,-1.78680816949054,
152.262842017495));
#161291=CARTESIAN_POINT('Ctrl Pts',(27.8053848024584,-2.23610566284,152.138110776586));
#161292=CARTESIAN_POINT('Ctrl Pts',(28.2922563302521,-2.59201839787431,
152.003684594481));
#161293=CARTESIAN_POINT('Ctrl Pts',(28.8060678733685,-2.88269490246962,
151.864609851225));
#161294=CARTESIAN_POINT('Ctrl Pts',(29.3380930897801,-3.12545698987924,
151.724680992667));
#161295=CARTESIAN_POINT('Ctrl Pts',(29.8802119089744,-3.3315629367898,151.586658563829));
#161296=CARTESIAN_POINT('Ctrl Pts',(30.4293702747731,-3.5100274763006,151.451374934494));
#161297=CARTESIAN_POINT('Ctrl Pts',(30.9988560924694,-3.67122058696772,
151.315485074222));
#161298=CARTESIAN_POINT('Ctrl Pts',(31.6039184811202,-3.82174819881736,
151.175566611529));
#161299=CARTESIAN_POINT('Ctrl Pts',(32.2586077383285,-3.96547007121551,
151.028836895302));
#161300=CARTESIAN_POINT('Ctrl Pts',(32.9681837842628,-4.10332519117328,
150.874625504658));
#161301=CARTESIAN_POINT('Ctrl Pts',(33.7411366378276,-4.23634581507805,
150.711639357809));
#161302=CARTESIAN_POINT('Ctrl Pts',(34.5880639009387,-4.3652675586447,150.538296513895));
#161303=CARTESIAN_POINT('Ctrl Pts',(35.5178717828348,-4.49005191045627,
150.353503384014));
#161304=CARTESIAN_POINT('Ctrl Pts',(36.5418485696312,-4.61060570740346,
150.155806013892));
#161305=CARTESIAN_POINT('Ctrl Pts',(37.5891726621944,-4.71793954069787,
149.959318019021));
#161306=CARTESIAN_POINT('Ctrl Pts',(38.2969062223127,-4.78144105096855,
149.829878192235));
#161307=CARTESIAN_POINT('Ctrl Pts',(38.6293920146191,-4.80952011478701,
149.769731800995));
#161308=CARTESIAN_POINT('Ctrl Pts',(38.77048515206,3.99237155033352,149.70739623108));
#161309=CARTESIAN_POINT('Ctrl Pts',(38.7084613789342,3.98711866251867,149.716657743131));
#161310=CARTESIAN_POINT('Ctrl Pts',(38.2511016937558,3.94799145212428,149.785077351974));
#161311=CARTESIAN_POINT('Ctrl Pts',(37.4313682141803,3.87256475402832,149.909402246761));
#161312=CARTESIAN_POINT('Ctrl Pts',(36.3408971723696,3.75847478669996,150.079092112684));
#161313=CARTESIAN_POINT('Ctrl Pts',(35.3395862968383,3.63994278190039,150.239102814392));
#161314=CARTESIAN_POINT('Ctrl Pts',(34.4177106792707,3.51681482324974,150.390547977447));
#161315=CARTESIAN_POINT('Ctrl Pts',(33.5659392784651,3.38854381493149,150.534587184947));
#161316=CARTESIAN_POINT('Ctrl Pts',(32.7769825454908,3.25438053296485,150.672144826256));
#161317=CARTESIAN_POINT('Ctrl Pts',(32.0457800700816,3.11346846660751,150.803833167474));
#161318=CARTESIAN_POINT('Ctrl Pts',(31.3688688032241,2.96481053892936,150.930009129647));
#161319=CARTESIAN_POINT('Ctrl Pts',(30.7426202066326,2.80683155589549,151.051068618564));
#161320=CARTESIAN_POINT('Ctrl Pts',(30.1626748117444,2.63691287705065,151.167554517892));
#161321=CARTESIAN_POINT('Ctrl Pts',(29.6237566708724,2.45067062972154,151.280203104165));
#161322=CARTESIAN_POINT('Ctrl Pts',(29.120750370036,2.24107601553824,151.389712767181));
#161323=CARTESIAN_POINT('Ctrl Pts',(28.6505813012899,1.99729222004304,151.49623650419));
#161324=CARTESIAN_POINT('Ctrl Pts',(28.2128464689627,1.70166153211956,151.599012295857));
#161325=CARTESIAN_POINT('Ctrl Pts',(27.8161807852202,1.32746699158294,151.69465045331));
#161326=CARTESIAN_POINT('Ctrl Pts',(27.4929941553154,0.843037147572355,
151.773521688089));
#161327=CARTESIAN_POINT('Ctrl Pts',(27.3153753829609,0.250080563879788,
151.816850273354));
#161328=CARTESIAN_POINT('Ctrl Pts',(27.3381602911532,-0.368260375098352,
151.811374813555));
#161329=CARTESIAN_POINT('Ctrl Pts',(27.5405501748278,-0.921138298860034,
151.762102665396));
#161330=CARTESIAN_POINT('Ctrl Pts',(27.8621521531751,-1.36846846005605,
151.683779547796));
#161331=CARTESIAN_POINT('Ctrl Pts',(28.2530528820034,-1.72323132189192,
151.589792530011));
#161332=CARTESIAN_POINT('Ctrl Pts',(28.6894815018612,-2.00997774512185,
151.487609628313));
#161333=CARTESIAN_POINT('Ctrl Pts',(29.1615492424393,-2.24874069898568,
151.380983484428));
#161334=CARTESIAN_POINT('Ctrl Pts',(29.6597632906639,-2.45160262431465,
151.272850376333));
#161335=CARTESIAN_POINT('Ctrl Pts',(30.174659009331,-2.62637778219187,151.165434742717));
#161336=CARTESIAN_POINT('Ctrl Pts',(30.7016670012872,-2.77960029340225,
151.059494894605));
#161337=CARTESIAN_POINT('Ctrl Pts',(31.252399319238,-2.91947774127626,150.95249406528));
#161338=CARTESIAN_POINT('Ctrl Pts',(31.8410743687168,-3.05138261896036,
150.841757960612));
#161339=CARTESIAN_POINT('Ctrl Pts',(32.481136182803,-3.17850347235832,150.725064225561));
#161340=CARTESIAN_POINT('Ctrl Pts',(33.1775813527336,-3.30154525563299,
150.601848983836));
#161341=CARTESIAN_POINT('Ctrl Pts',(33.938650360441,-3.42135361558111,150.471039189583));
#161342=CARTESIAN_POINT('Ctrl Pts',(34.7747427552922,-3.53856551809312,
150.331310663964));
#161343=CARTESIAN_POINT('Ctrl Pts',(35.6946436705373,-3.65315819682509,
150.181716199341));
#161344=CARTESIAN_POINT('Ctrl Pts',(36.7095268122545,-3.76509101025319,
150.021004038703));
#161345=CARTESIAN_POINT('Ctrl Pts',(37.7491015370053,-3.86600596623728,
149.860611162443));
#161346=CARTESIAN_POINT('Ctrl Pts',(38.4523857919031,-3.92649415040771,
149.754558862934));
#161347=CARTESIAN_POINT('Ctrl Pts',(38.7829212108065,-3.95341047095119,
149.705201381923));
#161348=CARTESIAN_POINT('Ctrl Pts',(38.9778745397249,3.19731394988081,149.999854791912));
#161349=CARTESIAN_POINT('Ctrl Pts',(38.916338543838,3.19148653742588,150.007208430689));
#161350=CARTESIAN_POINT('Ctrl Pts',(38.4626242424191,3.14816774453271,150.061488346695));
#161351=CARTESIAN_POINT('Ctrl Pts',(37.6500871839756,3.06583842590494,150.159510583659));
#161352=CARTESIAN_POINT('Ctrl Pts',(36.5711171193481,2.94425521394458,150.291751315632));
#161353=CARTESIAN_POINT('Ctrl Pts',(35.5825234494193,2.82065903999647,150.414951700963));
#161354=CARTESIAN_POINT('Ctrl Pts',(34.6747959447111,2.69486489432998,150.530092819935));
#161355=CARTESIAN_POINT('Ctrl Pts',(33.8388980789017,2.56638200743654,150.638150615903));
#161356=CARTESIAN_POINT('Ctrl Pts',(33.0679129044516,2.43463445681279,150.739883001722));
#161357=CARTESIAN_POINT('Ctrl Pts',(32.3572325368435,2.29907405188071,150.83578431523));
#161358=CARTESIAN_POINT('Ctrl Pts',(31.7039355846551,2.15917184513954,150.926142175826));
#161359=CARTESIAN_POINT('Ctrl Pts',(31.1050978364374,2.01406199300395,151.011255576643));
#161360=CARTESIAN_POINT('Ctrl Pts',(30.5573171327811,1.86223441262126,151.091505039686));
#161361=CARTESIAN_POINT('Ctrl Pts',(30.0566596083792,1.70110641993527,151.167371325102));
#161362=CARTESIAN_POINT('Ctrl Pts',(29.5998374677493,1.52665042186927,151.239264487423));
#161363=CARTESIAN_POINT('Ctrl Pts',(29.1859665623272,1.33302382532172,151.307204341295));
#161364=CARTESIAN_POINT('Ctrl Pts',(28.8167173246793,1.11106115618616,151.370660148695));
#161365=CARTESIAN_POINT('Ctrl Pts',(28.5001484425048,0.847535532219305,
151.42766752127));
#161366=CARTESIAN_POINT('Ctrl Pts',(28.2584910330725,0.528043369687139,
151.47305101709));
#161367=CARTESIAN_POINT('Ctrl Pts',(28.1325959852217,0.156106146179826,
151.49733827906));
#161368=CARTESIAN_POINT('Ctrl Pts',(28.1484032568081,-0.225985189187506,
151.494279745528));
#161369=CARTESIAN_POINT('Ctrl Pts',(28.2929267047297,-0.575198524295295,
151.466527011508));
#161370=CARTESIAN_POINT('Ctrl Pts',(28.5354640512508,-0.872474748378928,
151.421227158868));
#161371=CARTESIAN_POINT('Ctrl Pts',(28.8490257151681,-1.12360525762868,
151.365000995308));
#161372=CARTESIAN_POINT('Ctrl Pts',(29.2183489384953,-1.33969537808211,
151.301738585388));
#161373=CARTESIAN_POINT('Ctrl Pts',(29.6348883664465,-1.52990712165847,
151.233565391379));
#161374=CARTESIAN_POINT('Ctrl Pts',(30.0881306936774,-1.69914222580924,
151.162422669829));
#161375=CARTESIAN_POINT('Ctrl Pts',(30.5668214215576,-1.85046911839991,
151.089986846565));
#161376=CARTESIAN_POINT('Ctrl Pts',(31.0643743330293,-1.98717476103146,
151.017025604432));
#161377=CARTESIAN_POINT('Ctrl Pts',(31.5901717625383,-2.11511425971908,
150.941982485002));
#161378=CARTESIAN_POINT('Ctrl Pts',(32.1570609251648,-2.23845076038945,
150.863028933192));
#161379=CARTESIAN_POINT('Ctrl Pts',(32.7776793725769,-2.35976633813407,
150.778534659419));
#161380=CARTESIAN_POINT('Ctrl Pts',(33.4566732442955,-2.47947780796869,
150.688021723612));
#161381=CARTESIAN_POINT('Ctrl Pts',(34.2019510060455,-2.59825578166237,
150.590611811557));
#161382=CARTESIAN_POINT('Ctrl Pts',(35.0236487211914,-2.71668226239647,
150.485196195032));
#161383=CARTESIAN_POINT('Ctrl Pts',(35.9303903808119,-2.83476112433965,
150.370913196746));
#161384=CARTESIAN_POINT('Ctrl Pts',(36.9331972181514,-2.95254208528277,
150.246639883757));
#161385=CARTESIAN_POINT('Ctrl Pts',(37.9624832450496,-3.06120977505067,
150.121139581495));
#161386=CARTESIAN_POINT('Ctrl Pts',(38.6598615437989,-3.12787436936935,
150.037294403468));
#161387=CARTESIAN_POINT('Ctrl Pts',(38.9878083070654,-3.15786586028987,
149.998099350049));
#161388=CARTESIAN_POINT('Ctrl Pts',(39.199880276992,2.60290850229811,150.598231409948));
#161389=CARTESIAN_POINT('Ctrl Pts',(39.1388684177732,2.59581268633088,150.604130541553));
#161390=CARTESIAN_POINT('Ctrl Pts',(38.6890711795356,2.54315674757572,150.647607816424));
#161391=CARTESIAN_POINT('Ctrl Pts',(37.8842661670718,2.44431291877113,150.725226751088));
#161392=CARTESIAN_POINT('Ctrl Pts',(36.8176509876494,2.30146778174905,150.827652586784));
#161393=CARTESIAN_POINT('Ctrl Pts',(35.8427165320655,2.1592146055936,150.920837612846));
#161394=CARTESIAN_POINT('Ctrl Pts',(34.9501828329841,2.01731434812146,151.005711001615));
#161395=CARTESIAN_POINT('Ctrl Pts',(34.1313292830445,1.87529202353466,151.08313671715));
#161396=CARTESIAN_POINT('Ctrl Pts',(33.3796385940567,1.73271453214596,151.15375790474));
#161397=CARTESIAN_POINT('Ctrl Pts',(32.6909882310536,1.5893363355764,151.21798315668));
#161398=CARTESIAN_POINT('Ctrl Pts',(32.0630377144728,1.44511906750028,151.276049401746));
#161399=CARTESIAN_POINT('Ctrl Pts',(31.493618217534,1.29993330176996,151.328173959511));
#161400=CARTESIAN_POINT('Ctrl Pts',(30.9803543207786,1.15340323781994,151.374587937643));
#161401=CARTESIAN_POINT('Ctrl Pts',(30.5207516193253,1.00477545505744,151.415524615468));
#161402=CARTESIAN_POINT('Ctrl Pts',(30.1134825478559,0.853098687842271,
151.451100936464));
#161403=CARTESIAN_POINT('Ctrl Pts',(29.7600123204265,0.697738780618519,
151.48118360327));
#161404=CARTESIAN_POINT('Ctrl Pts',(29.4642352602667,0.538466875207633,
151.505455897129));
#161405=CARTESIAN_POINT('Ctrl Pts',(29.2335922986196,0.37639102177926,151.523408878111));
#161406=CARTESIAN_POINT('Ctrl Pts',(29.0793982921488,0.215720507103053,
151.534515800136));
#161407=CARTESIAN_POINT('Ctrl Pts',(29.009002582731,0.0624550682183219,
151.53915455036));
#161408=CARTESIAN_POINT('Ctrl Pts',(29.0173551306939,-0.0842942852346504,
151.538592549696));
#161409=CARTESIAN_POINT('Ctrl Pts',(29.0998481767366,-0.232711058266448,
151.533013599453));
#161410=CARTESIAN_POINT('Ctrl Pts',(29.257620688208,-0.386242434910132,
151.521457861273));
#161411=CARTESIAN_POINT('Ctrl Pts',(29.4882672850763,-0.542907343188585,
151.503354097979));
#161412=CARTESIAN_POINT('Ctrl Pts',(29.7856494770782,-0.69930384591628,
151.478829928837));
#161413=CARTESIAN_POINT('Ctrl Pts',(30.142662556554,-0.852883528720086,
151.448336973339));
#161414=CARTESIAN_POINT('Ctrl Pts',(30.5476985592488,-1.00069164313119,
151.412859979211));
#161415=CARTESIAN_POINT('Ctrl Pts',(30.9875832809003,-1.14058538588907,
151.373612036067));
#161416=CARTESIAN_POINT('Ctrl Pts',(31.4535676558278,-1.27241030149145,
151.331451977501));
#161417=CARTESIAN_POINT('Ctrl Pts',(31.9526434067819,-1.3998935441149,151.285802925616));
#161418=CARTESIAN_POINT('Ctrl Pts',(32.4961877440683,-1.52622614105896,
151.235630670283));
#161419=CARTESIAN_POINT('Ctrl Pts',(33.0959736577827,-1.65355532546756,
151.179824409168));
#161420=CARTESIAN_POINT('Ctrl Pts',(33.7562714775258,-1.78200644940902,
151.117956385245));
#161421=CARTESIAN_POINT('Ctrl Pts',(34.4846336892086,-1.91211751287444,
151.049283390676));
#161422=CARTESIAN_POINT('Ctrl Pts',(35.2909138741665,-2.04446893024473,
150.972831865546));
#161423=CARTESIAN_POINT('Ctrl Pts',(36.1835632153543,-2.17909741643894,
150.887749737191));
#161424=CARTESIAN_POINT('Ctrl Pts',(37.173439452658,-2.31616496109725,150.792946819857));
#161425=CARTESIAN_POINT('Ctrl Pts',(38.191710762274,-2.44539063098136,150.694986976225));
#161426=CARTESIAN_POINT('Ctrl Pts',(38.8827673371149,-2.52633282288444,
150.628254665011));
#161427=CARTESIAN_POINT('Ctrl Pts',(39.2079433948384,-2.56309542069976,
150.596804500242));
#161428=CARTESIAN_POINT('',(38.4389129826201,-4.64342671970106,149.800591313048));
#161429=CARTESIAN_POINT('Origin',(38.959854943863,-4.6434387520303,152.755016385081));
#161430=CARTESIAN_POINT('',(38.4242418866772,4.68124390104629,149.80317851189));
#161431=CARTESIAN_POINT('Origin',(38.9452145702245,4.68126981419974,152.757635929636));
#161432=CARTESIAN_POINT('Ctrl Pts',(38.4242420684175,4.68124390104622,149.803179542593));
#161433=CARTESIAN_POINT('Ctrl Pts',(38.1355463937705,4.62375019091924,149.854084254797));
#161434=CARTESIAN_POINT('Ctrl Pts',(37.8553097256357,4.56605654774142,149.903496984872));
#161435=CARTESIAN_POINT('Ctrl Pts',(37.5837514565077,4.50834271219169,149.951380422406));
#161436=CARTESIAN_POINT('Ctrl Pts',(37.4840243922502,4.48714788205486,149.968965136976));
#161437=CARTESIAN_POINT('Ctrl Pts',(37.3854678247398,4.46595084000668,149.986343492661));
#161438=CARTESIAN_POINT('Ctrl Pts',(37.2880928440942,4.44476214607814,150.003513312933));
#161439=CARTESIAN_POINT('Ctrl Pts',(37.2830066804605,4.44365540219186,150.004410139971));
#161440=CARTESIAN_POINT('Ctrl Pts',(37.2779237405206,4.44254868126253,150.00530639804));
#161441=CARTESIAN_POINT('Ctrl Pts',(37.2728440257589,4.44144198446882,150.006202086926));
#161442=CARTESIAN_POINT('Ctrl Pts',(36.9479699004643,4.37066298019586,150.063486040292));
#161443=CARTESIAN_POINT('Ctrl Pts',(36.6362872813769,4.29997312554706,150.118443805483));
#161444=CARTESIAN_POINT('Ctrl Pts',(36.3363798818645,4.22930880453252,150.171325919929));
#161445=CARTESIAN_POINT('Ctrl Pts',(36.2983021069356,4.22033690148688,150.178040103223));
#161446=CARTESIAN_POINT('Ctrl Pts',(36.2604141924949,4.211365449165,150.18472079319));
#161447=CARTESIAN_POINT('Ctrl Pts',(36.2227132740173,4.20239434386347,150.191368475827));
#161448=CARTESIAN_POINT('Ctrl Pts',(36.2217748164504,4.20217103361018,150.191533951054));
#161449=CARTESIAN_POINT('Ctrl Pts',(36.2208364747502,4.20194772357203,150.19169940583));
#161450=CARTESIAN_POINT('Ctrl Pts',(36.2198982488716,4.20172441374397,150.191864840162));
#161451=CARTESIAN_POINT('Ctrl Pts',(35.948661370091,4.13716654750797,150.239691160866));
#161452=CARTESIAN_POINT('Ctrl Pts',(35.6871028563909,4.07262604597075,150.285810438586));
#161453=CARTESIAN_POINT('Ctrl Pts',(35.4345007616386,4.00808082045874,150.330351422569));
#161454=CARTESIAN_POINT('Ctrl Pts',(35.3746566780167,3.99278938007412,150.340903648482));
#161455=CARTESIAN_POINT('Ctrl Pts',(35.3153153949423,3.97749786840843,150.351367208456));
#161456=CARTESIAN_POINT('Ctrl Pts',(35.2564674929442,3.96220630375595,150.361743678019));
#161457=CARTESIAN_POINT('Ctrl Pts',(35.2539306927745,3.96154711893392,150.362190984191));
#161458=CARTESIAN_POINT('Ctrl Pts',(35.2513948095389,3.96088793403217,150.362638128502));
#161459=CARTESIAN_POINT('Ctrl Pts',(35.2488598423598,3.96022874902138,150.363085111101));
#161460=CARTESIAN_POINT('Ctrl Pts',(35.0033444450969,3.89638568583368,150.406376050384));
#161461=CARTESIAN_POINT('Ctrl Pts',(34.7664193094501,3.83253763047813,150.448151774801));
#161462=CARTESIAN_POINT('Ctrl Pts',(34.5372789566154,3.76859345616774,150.488555818789));
#161463=CARTESIAN_POINT('Ctrl Pts',(34.4822394955994,3.75323407993558,150.498260861033));
#161464=CARTESIAN_POINT('Ctrl Pts',(34.4276493125477,3.73786934673916,150.50788667875));
#161465=CARTESIAN_POINT('Ctrl Pts',(34.37349746577,3.72249829637841,150.517435116911));
#161466=CARTESIAN_POINT('Ctrl Pts',(34.3680530896807,3.72095290533394,150.518395107964));
#161467=CARTESIAN_POINT('Ctrl Pts',(34.3626131447211,3.71940745057952,150.519354316762));
#161468=CARTESIAN_POINT('Ctrl Pts',(34.3571776208378,3.71786193124537,150.520312744973));
#161469=CARTESIAN_POINT('Ctrl Pts',(34.1432816612982,3.65704344381727,150.558028322412));
#161470=CARTESIAN_POINT('Ctrl Pts',(33.9362294158252,3.59612091795574,150.594536600627));
#161471=CARTESIAN_POINT('Ctrl Pts',(33.7354007572472,3.53497828185585,150.629948516004));
#161472=CARTESIAN_POINT('Ctrl Pts',(33.6770619370553,3.51721692608747,150.640235341493));
#161473=CARTESIAN_POINT('Ctrl Pts',(33.6192484739092,3.49943727844189,150.650429544792));
#161474=CARTESIAN_POINT('Ctrl Pts',(33.5619455742565,3.48163708652143,150.660533610237));
#161475=CARTESIAN_POINT('Ctrl Pts',(33.5540695998418,3.47919054617197,150.661922359522));
#161476=CARTESIAN_POINT('Ctrl Pts',(33.5462032696261,3.47674362287509,150.663309406071));
#161477=CARTESIAN_POINT('Ctrl Pts',(33.5383465770558,3.47429632079451,150.664694750628));
#161478=CARTESIAN_POINT('Ctrl Pts',(33.3659094274534,3.42058341409569,150.695100021608));
#161479=CARTESIAN_POINT('Ctrl Pts',(33.1981132959245,3.36668359002243,150.724686334537));
#161480=CARTESIAN_POINT('Ctrl Pts',(33.0348807818954,3.31259713924036,150.753468932572));
#161481=CARTESIAN_POINT('Ctrl Pts',(32.9604300875545,3.28792819482623,150.766596736316));
#161482=CARTESIAN_POINT('Ctrl Pts',(32.8869289989043,3.26322115034888,150.779557198536));
#161483=CARTESIAN_POINT('Ctrl Pts',(32.8143711806231,3.23847930299279,150.792351142007));
#161484=CARTESIAN_POINT('Ctrl Pts',(32.804489410665,3.23510966964793,150.794093570449));
#161485=CARTESIAN_POINT('Ctrl Pts',(32.7946251368876,3.23173938487948,150.795832909881));
#161486=CARTESIAN_POINT('Ctrl Pts',(32.7847783336901,3.22836845726935,150.797569163755));
#161487=CARTESIAN_POINT('Ctrl Pts',(32.6331987059228,3.17647710307769,150.824296692537));
#161488=CARTESIAN_POINT('Ctrl Pts',(32.4857575529114,3.12442888944696,150.850293861247));
#161489=CARTESIAN_POINT('Ctrl Pts',(32.342353896521,3.07220618801423,150.875580055377));
#161490=CARTESIAN_POINT('Ctrl Pts',(32.2698697907833,3.0458099586025,150.8883610905));
#161491=CARTESIAN_POINT('Ctrl Pts',(32.1984174902979,3.01937001141514,150.900960326406));
#161492=CARTESIAN_POINT('Ctrl Pts',(32.1279853768168,2.99288869106745,150.913379472003));
#161493=CARTESIAN_POINT('Ctrl Pts',(32.1165162491167,2.98857648702126,150.915401799031));
#161494=CARTESIAN_POINT('Ctrl Pts',(32.1050741724831,2.98426317007202,150.917419350178));
#161495=CARTESIAN_POINT('Ctrl Pts',(32.0936590979484,2.97994875777987,150.919432131884));
#161496=CARTESIAN_POINT('Ctrl Pts',(31.9628656099427,2.93051438653068,150.942494507794));
#161497=CARTESIAN_POINT('Ctrl Pts',(31.8356156817233,2.88093160537131,150.964931427134));
#161498=CARTESIAN_POINT('Ctrl Pts',(31.7118292366422,2.83117400237597,150.98675851427));
#161499=CARTESIAN_POINT('Ctrl Pts',(31.6402905927357,2.80241809586303,150.999372821217));
#161500=CARTESIAN_POINT('Ctrl Pts',(31.5699090493162,2.773604857122,151.011783287754));
#161501=CARTESIAN_POINT('Ctrl Pts',(31.5006712021453,2.74473655442193,151.023991877041));
#161502=CARTESIAN_POINT('Ctrl Pts',(31.4880120968377,2.73945841683006,151.026224035084));
#161503=CARTESIAN_POINT('Ctrl Pts',(31.4753912219212,2.73417839586638,151.02844944385));
#161504=CARTESIAN_POINT('Ctrl Pts',(31.4628084881326,2.72889652164137,151.030668115196));
#161505=CARTESIAN_POINT('Ctrl Pts',(31.3508495242083,2.68189932884144,151.050409464683));
#161506=CARTESIAN_POINT('Ctrl Pts',(31.241908972707,2.63475070775182,151.069617979236));
#161507=CARTESIAN_POINT('Ctrl Pts',(31.1359196205206,2.58741358020376,151.088306887775));
#161508=CARTESIAN_POINT('Ctrl Pts',(31.0660982212521,2.5562298394357,151.100618367354));
#161509=CARTESIAN_POINT('Ctrl Pts',(30.9975578850339,2.52496554483507,151.112704200039));
#161510=CARTESIAN_POINT('Ctrl Pts',(30.9302822292632,2.49362176653836,151.124566829132));
#161511=CARTESIAN_POINT('Ctrl Pts',(30.9168051726109,2.48734279577305,151.126943221045));
#161512=CARTESIAN_POINT('Ctrl Pts',(30.9033788717754,2.48106052889335,151.129310653308));
#161513=CARTESIAN_POINT('Ctrl Pts',(30.8900031337578,2.47477498992906,151.131669153867));
#161514=CARTESIAN_POINT('Ctrl Pts',(30.794615455276,2.42995032537447,151.148488554239));
#161515=CARTESIAN_POINT('Ctrl Pts',(30.7017981115883,2.38495443743262,151.164854175054));
#161516=CARTESIAN_POINT('Ctrl Pts',(30.61148076225,2.3397290349788,151.180779615583));
#161517=CARTESIAN_POINT('Ctrl Pts',(30.5444869012194,2.30618260841464,151.192592481632));
#161518=CARTESIAN_POINT('Ctrl Pts',(30.4788689138771,2.27251130679068,151.204163016596));
#161519=CARTESIAN_POINT('Ctrl Pts',(30.4146018444979,2.2387090720738,151.215495176014));
#161520=CARTESIAN_POINT('Ctrl Pts',(30.4006476140079,2.23136963402451,151.217955713984));
#161521=CARTESIAN_POINT('Ctrl Pts',(30.3867571048912,2.22402378188774,151.22040500559));
#161522=CARTESIAN_POINT('Ctrl Pts',(30.3729299231136,2.21667147155003,151.222843111905));
#161523=CARTESIAN_POINT('Ctrl Pts',(30.2923702339112,2.17383556722413,151.237047965077));
#161524=CARTESIAN_POINT('Ctrl Pts',(30.2139592078528,2.13077550160407,151.25087347165));
#161525=CARTESIAN_POINT('Ctrl Pts',(30.1376258859355,2.08740279169798,151.264333079088));
#161526=CARTESIAN_POINT('Ctrl Pts',(30.0739645180164,2.05123030537576,151.275558281918));
#161527=CARTESIAN_POINT('Ctrl Pts',(30.011748589835,2.01484184555696,151.286528882051));
#161528=CARTESIAN_POINT('Ctrl Pts',(29.9509417594417,1.97821297095187,151.297250929889));
#161529=CARTESIAN_POINT('Ctrl Pts',(29.9368185427894,1.96970541467192,151.299741271905));
#161530=CARTESIAN_POINT('Ctrl Pts',(29.9227714224001,1.96118449930074,151.302218188322));
#161531=CARTESIAN_POINT('Ctrl Pts',(29.9088002635435,1.95265029282505,151.304681693433));
#161532=CARTESIAN_POINT('Ctrl Pts',(29.8434571913563,1.9127358322189,151.316203500178));
#161533=CARTESIAN_POINT('Ctrl Pts',(29.7797753830253,1.87252556767506,151.327432057101));
#161534=CARTESIAN_POINT('Ctrl Pts',(29.7177587449049,1.83194049750251,151.338367175733));
#161535=CARTESIAN_POINT('Ctrl Pts',(29.6557421067844,1.79135542732997,151.349302294365));
#161536=CARTESIAN_POINT('Ctrl Pts',(29.5953908442221,1.75039647020468,151.359943927662));
#161537=CARTESIAN_POINT('Ctrl Pts',(29.5367111206233,1.70903815109368,151.370290919576));
#161538=CARTESIAN_POINT('Ctrl Pts',(29.5227530457233,1.69920029773504,151.372752146032));
#161539=CARTESIAN_POINT('Ctrl Pts',(29.5088896292455,1.68933928098665,151.375196684953));
#161540=CARTESIAN_POINT('Ctrl Pts',(29.4951218746314,1.67945619377341,151.377624354707));
#161541=CARTESIAN_POINT('Ctrl Pts',(29.4466018999985,1.64462646631817,151.386179887415));
#161542=CARTESIAN_POINT('Ctrl Pts',(29.3992707072912,1.60951838097622,151.39452574677));
#161543=CARTESIAN_POINT('Ctrl Pts',(29.3531993787577,1.57410391004019,151.402649291676));
#161544=CARTESIAN_POINT('Ctrl Pts',(29.3050768470894,1.53711270415614,151.411134515772));
#161545=CARTESIAN_POINT('Ctrl Pts',(29.2583291609921,1.49978748815046,151.419377141862));
#161546=CARTESIAN_POINT('Ctrl Pts',(29.2130253752663,1.46215189586027,151.42736534959));
#161547=CARTESIAN_POINT('Ctrl Pts',(29.1994676460809,1.45088897026082,151.429755921489));
#161548=CARTESIAN_POINT('Ctrl Pts',(29.1860391345271,1.43959859518491,151.432123727751));
#161549=CARTESIAN_POINT('Ctrl Pts',(29.17274143352,1.42828224908261,151.434468503544));
#161550=CARTESIAN_POINT('Ctrl Pts',(29.1594202525859,1.4169459215579,151.436817419537));
#161551=CARTESIAN_POINT('Ctrl Pts',(29.1462315112643,1.40558085731081,151.439143017953));
#161552=CARTESIAN_POINT('Ctrl Pts',(29.1331743741699,1.39418793964176,151.441445464654));
#161553=CARTESIAN_POINT('Ctrl Pts',(29.094039523704,1.36004108753139,151.448346357758));
#161554=CARTESIAN_POINT('Ctrl Pts',(29.0560887417731,1.32564002108451,151.455038804581));
#161555=CARTESIAN_POINT('Ctrl Pts',(29.0193620706213,1.29091789181491,151.461514806543));
#161556=CARTESIAN_POINT('Ctrl Pts',(28.9794896138272,1.25322167389802,151.468545503862));
#161557=CARTESIAN_POINT('Ctrl Pts',(28.9410601559824,1.21514758132632,151.475321066849));
#161558=CARTESIAN_POINT('Ctrl Pts',(28.9040958965794,1.17666455287375,151.481838344625));
#161559=CARTESIAN_POINT('Ctrl Pts',(28.8906638149357,1.16268058056042,151.484206594621));
#161560=CARTESIAN_POINT('Ctrl Pts',(28.8774249307655,1.14864305292917,151.486540804213));
#161561=CARTESIAN_POINT('Ctrl Pts',(28.8643793941046,1.1345518127135,151.488841034459));
#161562=CARTESIAN_POINT('Ctrl Pts',(28.852338354534,1.12154558802187,151.490964148604));
#161563=CARTESIAN_POINT('Ctrl Pts',(28.8404647618265,1.10849009751035,151.493057834043));
#161564=CARTESIAN_POINT('Ctrl Pts',(28.828758333926,1.09538770375143,151.495122225921));
#161565=CARTESIAN_POINT('Ctrl Pts',(28.8002025600444,1.06342671644882,151.500157947165));
#161566=CARTESIAN_POINT('Ctrl Pts',(28.7726447720803,1.03118399445943,151.50501857134));
#161567=CARTESIAN_POINT('Ctrl Pts',(28.7461821275536,0.998625628472416,
151.509685164022));
#161568=CARTESIAN_POINT('Ctrl Pts',(28.7180835161302,0.964054447442926,
151.514640253614));
#161569=CARTESIAN_POINT('Ctrl Pts',(28.6912197808251,0.929127997819401,
151.519376583851));
#161570=CARTESIAN_POINT('Ctrl Pts',(28.665658116513,0.893838741770888,151.523882827191));
#161571=CARTESIAN_POINT('Ctrl Pts',(28.6489002718861,0.870703633562121,
151.526837052894));
#161572=CARTESIAN_POINT('Ctrl Pts',(28.6327010237128,0.847413257758778,
151.529692623667));
#161573=CARTESIAN_POINT('Ctrl Pts',(28.6170686268516,0.823970377008213,
151.532448697277));
#161574=CARTESIAN_POINT('Ctrl Pts',(28.6071426818823,0.80908508805876,151.534198693469));
#161575=CARTESIAN_POINT('Ctrl Pts',(28.5974488492278,0.794137221794272,
151.535907951886));
#161576=CARTESIAN_POINT('Ctrl Pts',(28.5879885995462,0.779134708010062,
151.537576426224));
#161577=CARTESIAN_POINT('Ctrl Pts',(28.5702786751946,0.751049467858327,
151.540699869613));
#161578=CARTESIAN_POINT('Ctrl Pts',(28.5533911385098,0.722772919265728,
151.543679569537));
#161579=CARTESIAN_POINT('Ctrl Pts',(28.5374369545749,0.694380728259057,
151.54649407696));
#161580=CARTESIAN_POINT('Ctrl Pts',(28.5212919358127,0.665648926095429,
151.549342249913));
#161581=CARTESIAN_POINT('Ctrl Pts',(28.5061026110867,0.636798981699141,
151.552021313744));
#161582=CARTESIAN_POINT('Ctrl Pts',(28.4919314200231,0.607905927755162,
151.55451989888));
#161583=CARTESIAN_POINT('Ctrl Pts',(28.477447964955,0.578376211678344,151.55707354066));
#161584=CARTESIAN_POINT('Ctrl Pts',(28.4640278759436,0.548801765921204,
151.559438724222));
#161585=CARTESIAN_POINT('Ctrl Pts',(28.4516850436384,0.519254673332231,
151.561613683379));
#161586=CARTESIAN_POINT('Ctrl Pts',(28.4487242372839,0.512166898230697,
151.562135413945));
#161587=CARTESIAN_POINT('Ctrl Pts',(28.4458251912471,0.505080650072745,
151.562646241913));
#161588=CARTESIAN_POINT('Ctrl Pts',(28.4429876753242,0.497996828474827,
151.563146222405));
#161589=CARTESIAN_POINT('Ctrl Pts',(28.4363698149362,0.481475426084866,
151.564312313162));
#161590=CARTESIAN_POINT('Ctrl Pts',(28.4301044252218,0.464972804317448,
151.565416263435));
#161591=CARTESIAN_POINT('Ctrl Pts',(28.4241829166714,0.448484248438617,
151.566459789768));
#161592=CARTESIAN_POINT('Ctrl Pts',(28.4141536804503,0.42055764486347,151.568227206299));
#161593=CARTESIAN_POINT('Ctrl Pts',(28.4051119101709,0.39267552392786,151.569821089725));
#161594=CARTESIAN_POINT('Ctrl Pts',(28.3970398727197,0.364937280493078,
151.571244286348));
#161595=CARTESIAN_POINT('Ctrl Pts',(28.3885568109504,0.33578661886001,151.572739951468));
#161596=CARTESIAN_POINT('Ctrl Pts',(28.3811440360992,0.306794434072459,
151.574047256385));
#161597=CARTESIAN_POINT('Ctrl Pts',(28.3747692662043,0.278018244558982,
151.575171690596));
#161598=CARTESIAN_POINT('Ctrl Pts',(28.3679646708835,0.247301790829552,
151.576371940942));
#161599=CARTESIAN_POINT('Ctrl Pts',(28.3623418598648,0.216831067506705,
151.577364018936));
#161600=CARTESIAN_POINT('Ctrl Pts',(28.3578616131784,0.18661797755784,151.578154296732));
#161601=CARTESIAN_POINT('Ctrl Pts',(28.3572889513731,0.182756162830784,
151.578255309453));
#161602=CARTESIAN_POINT('Ctrl Pts',(28.3567349677807,0.178898488924442,
151.578353022512));
#161603=CARTESIAN_POINT('Ctrl Pts',(28.356199592719,0.175044923013026,151.578447446375));
#161604=CARTESIAN_POINT('Ctrl Pts',(28.3538069307026,0.157822826872332,
151.57886943912));
#161605=CARTESIAN_POINT('Ctrl Pts',(28.3517923553221,0.140707906652478,
151.579224611498));
#161606=CARTESIAN_POINT('Ctrl Pts',(28.3501553603895,0.123671004711587,
151.579512843201));
#161607=CARTESIAN_POINT('Ctrl Pts',(28.3477486824018,0.0986236841233151,
151.579936595824));
#161608=CARTESIAN_POINT('Ctrl Pts',(28.3461551320974,0.073745843099456,
151.580216238149));
#161609=CARTESIAN_POINT('Ctrl Pts',(28.3452992114535,0.0489932041348807,
151.580366104403));
#161610=CARTESIAN_POINT('Ctrl Pts',(28.3444242118242,0.0236888139759929,
151.580519311265));
#161611=CARTESIAN_POINT('Ctrl Pts',(28.3443202264207,-0.00148569978635055,
151.580536857902));
#161612=CARTESIAN_POINT('Ctrl Pts',(28.3449599427278,-0.0265873899183545,
151.580423929627));
#161613=CARTESIAN_POINT('Ctrl Pts',(28.3456024747252,-0.0517995643143712,
151.580310504301));
#161614=CARTESIAN_POINT('Ctrl Pts',(28.3469954415848,-0.0769392452442724,
151.580065418563));
#161615=CARTESIAN_POINT('Ctrl Pts',(28.3491618389979,-0.102059265144167,
151.579684384792));
#161616=CARTESIAN_POINT('Ctrl Pts',(28.3500423370033,-0.112268900404609,
151.579529519635));
#161617=CARTESIAN_POINT('Ctrl Pts',(28.3510511638344,-0.122475149165934,
151.57935209078));
#161618=CARTESIAN_POINT('Ctrl Pts',(28.3521921649127,-0.132680756132027,
151.579151376766));
#161619=CARTESIAN_POINT('Ctrl Pts',(28.3541677950609,-0.150351646357203,
151.578803842777));
#161620=CARTESIAN_POINT('Ctrl Pts',(28.3564988941821,-0.168027950876555,
151.578393700082));
#161621=CARTESIAN_POINT('Ctrl Pts',(28.3592130136351,-0.185705005592994,
151.577915738267));
#161622=CARTESIAN_POINT('Ctrl Pts',(28.3636447570318,-0.214568941712832,
151.577135299472));
#161623=CARTESIAN_POINT('Ctrl Pts',(28.3690968123005,-0.243436794795253,
151.576174203392));
#161624=CARTESIAN_POINT('Ctrl Pts',(28.375586296123,-0.272386597642406,
151.575029920963));
#161625=CARTESIAN_POINT('Ctrl Pts',(28.3819105022187,-0.300599091061347,
151.573914781745));
#161626=CARTESIAN_POINT('Ctrl Pts',(28.3892210531441,-0.328889780272276,
151.572625452078));
#161627=CARTESIAN_POINT('Ctrl Pts',(28.3975532793529,-0.357287510894987,
151.571155919633));
#161628=CARTESIAN_POINT('Ctrl Pts',(28.4054830898646,-0.384313736198647,
151.569757360168));
#161629=CARTESIAN_POINT('Ctrl Pts',(28.414339212776,-0.411437132340805,
151.568195394969));
#161630=CARTESIAN_POINT('Ctrl Pts',(28.4241555309917,-0.438638844865651,
151.566464358249));
#161631=CARTESIAN_POINT('Ctrl Pts',(28.4309737242029,-0.457532540811235,
151.56526201919));
#161632=CARTESIAN_POINT('Ctrl Pts',(28.438246110612,-0.476505520160626,
151.563979708771));
#161633=CARTESIAN_POINT('Ctrl Pts',(28.4459628434618,-0.495499582166659,
151.562619400363));
#161634=CARTESIAN_POINT('Ctrl Pts',(28.4579981129699,-0.525123343898964,
151.56049781878));
#161635=CARTESIAN_POINT('Ctrl Pts',(28.4711159948491,-0.554796776916299,
151.558186201867));
#161636=CARTESIAN_POINT('Ctrl Pts',(28.4853086342612,-0.584441168488999,
151.55568470758));
#161637=CARTESIAN_POINT('Ctrl Pts',(28.4992664688762,-0.61359511954932,
151.553224598328));
#161638=CARTESIAN_POINT('Ctrl Pts',(28.5142638513556,-0.642720753405762,
151.550580795653));
#161639=CARTESIAN_POINT('Ctrl Pts',(28.5302441252966,-0.671744059448906,
151.547762810325));
#161640=CARTESIAN_POINT('Ctrl Pts',(28.5444347335186,-0.69751698217131,
151.545260417318));
#161641=CARTESIAN_POINT('Ctrl Pts',(28.5593997749469,-0.723209106787243,
151.542620773781));
#161642=CARTESIAN_POINT('Ctrl Pts',(28.5750658528408,-0.748771480970023,
151.539857312333));
#161643=CARTESIAN_POINT('Ctrl Pts',(28.5873730698822,-0.768853194420763,
151.537686346502));
#161644=CARTESIAN_POINT('Ctrl Pts',(28.6001545842406,-0.788851285535069,
151.535431631614));
#161645=CARTESIAN_POINT('Ctrl Pts',(28.6133751259987,-0.808770178727065,
151.533100099107));
#161646=CARTESIAN_POINT('Ctrl Pts',(28.6404673054132,-0.849588946820708,
151.528322208901));
#161647=CARTESIAN_POINT('Ctrl Pts',(28.6694038328263,-0.890073648743999,
151.523221589708));
#161648=CARTESIAN_POINT('Ctrl Pts',(28.7002046692454,-0.930291659501632,
151.517791423635));
#161649=CARTESIAN_POINT('Ctrl Pts',(28.7267366815885,-0.964935678362477,
151.513113848282));
#161650=CARTESIAN_POINT('Ctrl Pts',(28.7546521213732,-0.999381024742059,
151.508191709033));
#161651=CARTESIAN_POINT('Ctrl Pts',(28.7839279689917,-1.03369193195231,
151.503028897144));
#161652=CARTESIAN_POINT('Ctrl Pts',(28.788638257889,-1.03921232840313,151.502198235096));
#161653=CARTESIAN_POINT('Ctrl Pts',(28.7933836764714,-1.04472930869436,
151.501361363159));
#161654=CARTESIAN_POINT('Ctrl Pts',(28.7981640235505,-1.05024322169471,
151.50051832233));
#161655=CARTESIAN_POINT('Ctrl Pts',(28.8158944374376,-1.07069444793768,
151.497391465103));
#161656=CARTESIAN_POINT('Ctrl Pts',(28.83411887679,-1.0910920270257,151.494177326023));
#161657=CARTESIAN_POINT('Ctrl Pts',(28.8528112558912,-1.11144444760841,
151.490881046906));
#161658=CARTESIAN_POINT('Ctrl Pts',(28.8868664466705,-1.14852402758114,
151.484875636169));
#161659=CARTESIAN_POINT('Ctrl Pts',(28.9224751947787,-1.18545262339267,
151.478597567753));
#161660=CARTESIAN_POINT('Ctrl Pts',(28.9596250610351,-1.22218491422455,
151.472047517969));
#161661=CARTESIAN_POINT('Ctrl Pts',(28.9942912862789,-1.25646148089941,
151.465935369419));
#161662=CARTESIAN_POINT('Ctrl Pts',(29.0302992476044,-1.29056663370428,
151.459586407157));
#161663=CARTESIAN_POINT('Ctrl Pts',(29.0676137132796,-1.32450220720318,
151.453006594243));
#161664=CARTESIAN_POINT('Ctrl Pts',(29.0745937530851,-1.33085019181332,
151.451775775171));
#161665=CARTESIAN_POINT('Ctrl Pts',(29.0816194390092,-1.33719236984751,
151.450536894129));
#161666=CARTESIAN_POINT('Ctrl Pts',(29.0886904426302,-1.34352893841016,
151.449290012448));
#161667=CARTESIAN_POINT('Ctrl Pts',(29.1120739001454,-1.36448365569211,
151.445166636703));
#161668=CARTESIAN_POINT('Ctrl Pts',(29.1359606208211,-1.38536449157222,
151.44095439532));
#161669=CARTESIAN_POINT('Ctrl Pts',(29.1603176844792,-1.40617450552468,
151.436659366932));
#161670=CARTESIAN_POINT('Ctrl Pts',(29.204187252997,-1.4436554739107,151.428923580518));
#161671=CARTESIAN_POINT('Ctrl Pts',(29.2495829757347,-1.48090508051263,
151.420919216224));
#161672=CARTESIAN_POINT('Ctrl Pts',(29.2963865595,-1.51783781305876,151.412666627315));
#161673=CARTESIAN_POINT('Ctrl Pts',(29.3431901432653,-1.55477054560488,
151.404414038406));
#161674=CARTESIAN_POINT('Ctrl Pts',(29.3914012702663,-1.59138588765514,
151.395913272225));
#161675=CARTESIAN_POINT('Ctrl Pts',(29.4408862584704,-1.62765597376399,
151.387187715802));
#161676=CARTESIAN_POINT('Ctrl Pts',(29.4697729320755,-1.64882849854538,
151.382094205435));
#161677=CARTESIAN_POINT('Ctrl Pts',(29.4990964040957,-1.66987327465208,
151.376923623045));
#161678=CARTESIAN_POINT('Ctrl Pts',(29.5288210851771,-1.69079349879652,
151.371682274741));
#161679=CARTESIAN_POINT('Ctrl Pts',(29.583881306592,-1.7295448707721,151.361973514624));
#161680=CARTESIAN_POINT('Ctrl Pts',(29.6403183269796,-1.76786694464797,
151.352021960529));
#161681=CARTESIAN_POINT('Ctrl Pts',(29.6979412888232,-1.80568579260789,
151.341861469206));
#161682=CARTESIAN_POINT('Ctrl Pts',(29.7453791455287,-1.83681999732234,
151.333496888213));
#161683=CARTESIAN_POINT('Ctrl Pts',(29.7936205341707,-1.8676140656969,151.324990737202));
#161684=CARTESIAN_POINT('Ctrl Pts',(29.8425576044251,-1.89805327876354,
151.316361925641));
#161685=CARTESIAN_POINT('Ctrl Pts',(29.8762442931379,-1.91900664376693,
151.310422132198));
#161686=CARTESIAN_POINT('Ctrl Pts',(29.9102614845754,-1.93978414451622,
151.304424061161));
#161687=CARTESIAN_POINT('Ctrl Pts',(29.9445834524753,-1.96039441044776,
151.298372151826));
#161688=CARTESIAN_POINT('Ctrl Pts',(30.0160630182559,-2.00331773185241,
151.2857683334));
#161689=CARTESIAN_POINT('Ctrl Pts',(30.0888641235138,-2.04551315584805,
151.27293115869));
#161690=CARTESIAN_POINT('Ctrl Pts',(30.1627771933051,-2.08695944696762,
151.259898287955));
#161691=CARTESIAN_POINT('Ctrl Pts',(30.2013677697836,-2.10859887111432,
151.253093726917));
#161692=CARTESIAN_POINT('Ctrl Pts',(30.24026157973,-2.13003494085121,151.246235777382));
#161693=CARTESIAN_POINT('Ctrl Pts',(30.2794297577773,-2.1512701895881,151.239329476774));
#161694=CARTESIAN_POINT('Ctrl Pts',(30.3170942296121,-2.17169019551711,
151.232688316075));
#161695=CARTESIAN_POINT('Ctrl Pts',(30.3550119234677,-2.19192082334998,
151.226002530369));
#161696=CARTESIAN_POINT('Ctrl Pts',(30.3931414253752,-2.21196230894521,
151.219279278749));
#161697=CARTESIAN_POINT('Ctrl Pts',(30.4752143388864,-2.25510116551577,
151.204807627633));
#161698=CARTESIAN_POINT('Ctrl Pts',(30.5582681288881,-2.29736068686337,
151.190162591056));
#161699=CARTESIAN_POINT('Ctrl Pts',(30.6418972610801,-2.33867977594509,
151.175416540789));
#161700=CARTESIAN_POINT('Ctrl Pts',(30.6743627499852,-2.35472017231165,
151.169692007738));
#161701=CARTESIAN_POINT('Ctrl Pts',(30.7069150439222,-2.37061940436573,
151.163952214052));
#161702=CARTESIAN_POINT('Ctrl Pts',(30.7395308275734,-2.3863759309605,151.158201245153));
#161703=CARTESIAN_POINT('Ctrl Pts',(30.7807271122191,-2.40627765589118,
151.150937321825));
#161704=CARTESIAN_POINT('Ctrl Pts',(30.8220259218793,-2.42594287864325,
151.143655355438));
#161705=CARTESIAN_POINT('Ctrl Pts',(30.863562833521,-2.44545103297551,151.136331292355));
#161706=CARTESIAN_POINT('Ctrl Pts',(30.945172341805,-2.48377961398125,151.121941363897));
#161707=CARTESIAN_POINT('Ctrl Pts',(31.0276994465686,-2.52150490099597,
151.107389275528));
#161708=CARTESIAN_POINT('Ctrl Pts',(31.112191669517,-2.55913493840193,151.09249101624));
#161709=CARTESIAN_POINT('Ctrl Pts',(31.1471908701709,-2.57472242307004,
151.086319712562));
#161710=CARTESIAN_POINT('Ctrl Pts',(31.1825275816439,-2.59029299310569,
151.080088938532));
#161711=CARTESIAN_POINT('Ctrl Pts',(31.2182775590854,-2.60588061303104,
151.073785315971));
#161712=CARTESIAN_POINT('Ctrl Pts',(31.2634312776054,-2.62556842972012,
151.065823576716));
#161713=CARTESIAN_POINT('Ctrl Pts',(31.3092419322252,-2.64528679282138,
151.057746041459));
#161714=CARTESIAN_POINT('Ctrl Pts',(31.3557214141397,-2.66503620428409,
151.049550455661));
#161715=CARTESIAN_POINT('Ctrl Pts',(31.4731874039566,-2.71494820997369,
151.028838034649));
#161716=CARTESIAN_POINT('Ctrl Pts',(31.5949248965874,-2.76505561399907,
151.007371934376));
#161717=CARTESIAN_POINT('Ctrl Pts',(31.7211181180094,-2.81530679931872,
150.98512086285));
#161718=CARTESIAN_POINT('Ctrl Pts',(31.7285406554425,-2.81826251516373,
150.983812080893));
#161719=CARTESIAN_POINT('Ctrl Pts',(31.7359786106392,-2.82121874361973,
150.982500581475));
#161720=CARTESIAN_POINT('Ctrl Pts',(31.7434320221541,-2.82417548019535,
150.98118635752));
#161721=CARTESIAN_POINT('Ctrl Pts',(31.7957981714862,-2.84494890840955,
150.971952888028));
#161722=CARTESIAN_POINT('Ctrl Pts',(31.8489268182686,-2.8657461266685,150.962585025477));
#161723=CARTESIAN_POINT('Ctrl Pts',(31.9027999515756,-2.88655862667242,
150.953085748909));
#161724=CARTESIAN_POINT('Ctrl Pts',(32.0241632686974,-2.93344422405697,
150.931686144991));
#161725=CARTESIAN_POINT('Ctrl Pts',(32.1493046661099,-2.9804044103554,150.909619836333));
#161726=CARTESIAN_POINT('Ctrl Pts',(32.2780098009442,-3.02731403789428,
150.886925789182));
#161727=CARTESIAN_POINT('Ctrl Pts',(32.2932592768915,-3.03287206973018,
150.884236911798));
#161728=CARTESIAN_POINT('Ctrl Pts',(32.308558787786,-3.0384294518267,150.881539216878));
#161729=CARTESIAN_POINT('Ctrl Pts',(32.3239079825989,-3.04398602555797,
150.878832764762));
#161730=CARTESIAN_POINT('Ctrl Pts',(32.3837616995455,-3.06565371532004,
150.868279037293));
#161731=CARTESIAN_POINT('Ctrl Pts',(32.4443708346114,-3.08730579589398,
150.857592178118));
#161732=CARTESIAN_POINT('Ctrl Pts',(32.5057826768735,-3.10895759434287,
150.846763625539));
#161733=CARTESIAN_POINT('Ctrl Pts',(32.6520415155047,-3.16052365682793,
150.82097427505));
#161734=CARTESIAN_POINT('Ctrl Pts',(32.8028522891403,-3.21208759517891,
150.794381722189));
#161735=CARTESIAN_POINT('Ctrl Pts',(32.9588518239448,-3.26379216756449,
150.766875021505));
#161736=CARTESIAN_POINT('Ctrl Pts',(33.0267189636895,-3.28628609002349,
150.754908312107));
#161737=CARTESIAN_POINT('Ctrl Pts',(33.095567935825,-3.30880544892256,150.742768561037));
#161738=CARTESIAN_POINT('Ctrl Pts',(33.1654559814257,-3.33136269090447,
150.730445423497));
#161739=CARTESIAN_POINT('Ctrl Pts',(33.3236650123146,-3.38242663700293,
150.702548926592));
#161740=CARTESIAN_POINT('Ctrl Pts',(33.4871980878252,-3.43368438659886,
150.673713065512));
#161741=CARTESIAN_POINT('Ctrl Pts',(33.6567152282543,-3.48522689816105,
150.643822845968));
#161742=CARTESIAN_POINT('Ctrl Pts',(33.7342656058241,-3.50880646788727,
150.630148725432));
#161743=CARTESIAN_POINT('Ctrl Pts',(33.8130680689335,-3.5324448583529,150.616253928583));
#161744=CARTESIAN_POINT('Ctrl Pts',(33.8931663711956,-3.55614539415555,
150.602130447634));
#161745=CARTESIAN_POINT('Ctrl Pts',(34.0654983557839,-3.6071372411152,150.571743692455));
#161746=CARTESIAN_POINT('Ctrl Pts',(34.2438282940683,-3.65841587270872,
150.540298707114));
#161747=CARTESIAN_POINT('Ctrl Pts',(34.4285857022663,-3.70997574003565,
150.507721218515));
#161748=CARTESIAN_POINT('Ctrl Pts',(34.5174378428953,-3.73477152293401,
150.492054298164));
#161749=CARTESIAN_POINT('Ctrl Pts',(34.6077762076357,-3.75963167638948,
150.476125439459));
#161750=CARTESIAN_POINT('Ctrl Pts',(34.6996284915187,-3.78455204436383,
150.459929416915));
#161751=CARTESIAN_POINT('Ctrl Pts',(34.8875451472379,-3.83553555844819,
150.42679466769));
#161752=CARTESIAN_POINT('Ctrl Pts',(35.0817980643923,-3.88676991673767,
150.392541997972));
#161753=CARTESIAN_POINT('Ctrl Pts',(35.2826173101892,-3.93819091351075,
150.357132371598));
#161754=CARTESIAN_POINT('Ctrl Pts',(35.3841707649635,-3.96419429704864,
150.33922587127));
#161755=CARTESIAN_POINT('Ctrl Pts',(35.4874032666831,-3.99024409064252,
150.321023457094));
#161756=CARTESIAN_POINT('Ctrl Pts',(35.5923818810437,-4.01634509594526,
150.302512907189));
#161757=CARTESIAN_POINT('Ctrl Pts',(35.7964653212263,-4.06708669685938,
150.266527514095));
#161758=CARTESIAN_POINT('Ctrl Pts',(36.0071475076086,-4.11802152632512,
150.229377874438));
#161759=CARTESIAN_POINT('Ctrl Pts',(36.2249165241759,-4.16915107162306,
150.190979540965));
#161760=CARTESIAN_POINT('Ctrl Pts',(36.3407061067015,-4.19633707263501,
150.170562830303));
#161761=CARTESIAN_POINT('Ctrl Pts',(36.4584992550742,-4.223574957414,150.149793018105));
#161762=CARTESIAN_POINT('Ctrl Pts',(36.5785563414473,-4.25090433708211,
150.128623742154));
#161763=CARTESIAN_POINT('Ctrl Pts',(36.8004411562673,-4.30141342846524,
150.089499513706));
#161764=CARTESIAN_POINT('Ctrl Pts',(37.0300583269974,-4.35223731265307,
150.049011151743));
#161765=CARTESIAN_POINT('Ctrl Pts',(37.2690508250992,-4.40356217142764,
150.006870546684));
#161766=CARTESIAN_POINT('Ctrl Pts',(37.4018946875305,-4.432091068914,149.983446712105));
#161767=CARTESIAN_POINT('Ctrl Pts',(37.5376345268245,-4.46077723240068,
149.959512436394));
#161768=CARTESIAN_POINT('Ctrl Pts',(37.6761845465022,-4.48957184343251,
149.935082274819));
#161769=CARTESIAN_POINT('Ctrl Pts',(37.9217607278213,-4.5406095165863,149.891780470875));
#161770=CARTESIAN_POINT('Ctrl Pts',(38.1761656186326,-4.59198577347407,
149.846920932356));
#161771=CARTESIAN_POINT('Ctrl Pts',(38.4389130596078,-4.64342671970294,
149.800591749672));
#161772=CARTESIAN_POINT('Ctrl Pts',(38.2563686252732,-5.2146737148978,149.893918127215));
#161773=CARTESIAN_POINT('Ctrl Pts',(39.0894774938447,-5.33014235717708,
149.737171640936));
#161774=CARTESIAN_POINT('Ctrl Pts',(41.0081884734667,-5.57912789308956,
149.379459681224));
#161775=CARTESIAN_POINT('Ctrl Pts',(43.8076126339424,-5.89407254053238,
148.867077378471));
#161776=CARTESIAN_POINT('Ctrl Pts',(45.7742555008851,-6.08603592631556,
148.51299562346));
#161777=CARTESIAN_POINT('Ctrl Pts',(46.6545489230723,-6.16674235624256,
148.355562055461));
#161778=CARTESIAN_POINT('Ctrl Pts',(38.4107421964028,-4.21574620337288,
149.656528322788));
#161779=CARTESIAN_POINT('Ctrl Pts',(39.2410978032759,-4.326693041109,149.517014569386));
#161780=CARTESIAN_POINT('Ctrl Pts',(41.1541027316362,-4.56669801382285,
149.198100963248));
#161781=CARTESIAN_POINT('Ctrl Pts',(43.9467860391103,-4.87254124748984,
148.739774565811));
#161782=CARTESIAN_POINT('Ctrl Pts',(45.9095185461389,-5.06048947264209,
148.422110282307));
#161783=CARTESIAN_POINT('Ctrl Pts',(46.7881932180747,-5.13981749100654,
148.280699000599));
#161784=CARTESIAN_POINT('Ctrl Pts',(38.6491896496085,-3.24092093422417,
149.922799308253));
#161785=CARTESIAN_POINT('Ctrl Pts',(39.4753249802897,-3.35550158914587,
149.800373415778));
#161786=CARTESIAN_POINT('Ctrl Pts',(41.3795854643966,-3.60487788190061,
149.519415986963));
#161787=CARTESIAN_POINT('Ctrl Pts',(44.1619431823615,-3.92708203095172,
149.112469591543));
#161788=CARTESIAN_POINT('Ctrl Pts',(46.1186883385217,-4.12806188523935,
148.828465887092));
#161789=CARTESIAN_POINT('Ctrl Pts',(46.9948848783835,-4.21348716646631,
148.701686738985));
#161790=CARTESIAN_POINT('Ctrl Pts',(38.9139099282385,-2.52650125174993,
150.628185440083));
#161791=CARTESIAN_POINT('Ctrl Pts',(39.735380987824,-2.6519904870564,150.51856033928));
#161792=CARTESIAN_POINT('Ctrl Pts',(41.6299783390877,-2.92681832032616,
150.265516112064));
#161793=CARTESIAN_POINT('Ctrl Pts',(44.4009287142964,-3.28687973238183,
149.894819002744));
#161794=CARTESIAN_POINT('Ctrl Pts',(46.3510608975163,-3.51477906248343,
149.633559463568));
#161795=CARTESIAN_POINT('Ctrl Pts',(47.224520637165,-3.61229926883204,149.516475381658));
#161796=CARTESIAN_POINT('Origin',(47.1132772922885,-6.0105076275006,151.317336462008));
#161797=CARTESIAN_POINT('Origin',(80.6089045065798,1.68883371573741,142.364600992296));
#161798=CARTESIAN_POINT('Ctrl Pts',(46.5372798889843,-6.18969355892611,
148.377359242795));
#161799=CARTESIAN_POINT('Ctrl Pts',(46.5530418433047,-6.17420698012464,
148.374439381584));
#161800=CARTESIAN_POINT('Ctrl Pts',(46.5891375270505,-6.14390732156202,
148.366955781747));
#161801=CARTESIAN_POINT('Ctrl Pts',(46.6370786313459,-6.12575715622293,
148.353663770989));
#161802=CARTESIAN_POINT('Ctrl Pts',(46.6799969179442,-6.14247380870429,
148.336241564642));
#161803=CARTESIAN_POINT('Ctrl Pts',(46.7141598403172,-6.19433188653137,
148.314694318236));
#161804=CARTESIAN_POINT('Ctrl Pts',(46.740186434731,-6.28393425976963,148.286265932497));
#161805=CARTESIAN_POINT('Ctrl Pts',(46.7562543404266,-6.41410945175322,
148.247747808364));
#161806=CARTESIAN_POINT('Ctrl Pts',(46.7588839610926,-6.58557960151583,
148.195575967713));
#161807=CARTESIAN_POINT('Ctrl Pts',(46.7429079185317,-6.79517545380282,
148.126545779614));
#161808=CARTESIAN_POINT('Ctrl Pts',(46.7025952223824,-7.02972718747325,
148.040949139118));
#161809=CARTESIAN_POINT('Ctrl Pts',(46.6390661764921,-7.25532850484998,
147.950480251073));
#161810=CARTESIAN_POINT('Ctrl Pts',(46.5838544263694,-7.39557475298945,
147.891484586532));
#161811=CARTESIAN_POINT('Ctrl Pts',(46.5562789209077,-7.45747517935645,
147.865484750416));
#161812=CARTESIAN_POINT('Ctrl Pts',(46.6614159728208,-4.66729930170419,
148.257452201144));
#161813=CARTESIAN_POINT('Ctrl Pts',(46.7082864496826,-4.65394890463263,
148.259742715989));
#161814=CARTESIAN_POINT('Ctrl Pts',(46.8220720189848,-4.63185018237409,
148.258397988294));
#161815=CARTESIAN_POINT('Ctrl Pts',(46.9900857215236,-4.63807663592174,
148.228394581823));
#161816=CARTESIAN_POINT('Ctrl Pts',(47.1476688845866,-4.69207724165032,
148.16235802505));
#161817=CARTESIAN_POINT('Ctrl Pts',(47.268966626375,-4.78579128608015,148.069473219709));
#161818=CARTESIAN_POINT('Ctrl Pts',(47.3488929397349,-4.9165280755285,147.953204928739));
#161819=CARTESIAN_POINT('Ctrl Pts',(47.3795139884807,-5.08012483101266,
147.820397899541));
#161820=CARTESIAN_POINT('Ctrl Pts',(47.3553608942353,-5.27046229206427,
147.680852284493));
#161821=CARTESIAN_POINT('Ctrl Pts',(47.2751162928573,-5.47954989994779,
147.546633237318));
#161822=CARTESIAN_POINT('Ctrl Pts',(47.1459322366506,-5.69408256980547,
147.432441796637));
#161823=CARTESIAN_POINT('Ctrl Pts',(46.9940609684127,-5.8891790323644,147.352132634224));
#161824=CARTESIAN_POINT('Ctrl Pts',(46.8866314685821,-6.00813031043961,
147.315693823849));
#161825=CARTESIAN_POINT('Ctrl Pts',(46.8367952618753,-6.06059112023815,
147.301954032457));
#161826=CARTESIAN_POINT('Ctrl Pts',(46.8710872569602,-3.43668272451928,
149.145776253864));
#161827=CARTESIAN_POINT('Ctrl Pts',(46.9688797033509,-3.43299183240254,
149.149417466047));
#161828=CARTESIAN_POINT('Ctrl Pts',(47.208707877535,-3.436874534301,149.143294412863));
#161829=CARTESIAN_POINT('Ctrl Pts',(47.57336636799,-3.49322218855088,149.073387019189));
#161830=CARTESIAN_POINT('Ctrl Pts',(47.9321847007078,-3.61121601093276,
148.924034453737));
#161831=CARTESIAN_POINT('Ctrl Pts',(48.2304282189886,-3.77344247675182,
148.713447706702));
#161832=CARTESIAN_POINT('Ctrl Pts',(48.4598429050887,-3.97434236430038,
148.445541633467));
#161833=CARTESIAN_POINT('Ctrl Pts',(48.6048887356042,-4.20444485705,148.130362491661));
#161834=CARTESIAN_POINT('Ctrl Pts',(48.6528396833208,-4.45151086311779,
147.783563554233));
#161835=CARTESIAN_POINT('Ctrl Pts',(48.596201214212,-4.7015403993278,147.425907696623));
#161836=CARTESIAN_POINT('Ctrl Pts',(48.4387335772696,-4.93613819975849,
147.087807525499));
#161837=CARTESIAN_POINT('Ctrl Pts',(48.2157364293847,-5.13002728547283,
146.811790570649));
#161838=CARTESIAN_POINT('Ctrl Pts',(48.0410663087532,-5.23832449722567,
146.663304223064));
#161839=CARTESIAN_POINT('Ctrl Pts',(47.9571770914129,-5.28424701090955,
146.602254477145));
#161840=CARTESIAN_POINT('Ctrl Pts',(47.067244768031,-3.07918861709148,150.622686022086));
#161841=CARTESIAN_POINT('Ctrl Pts',(47.211717029689,-3.0881173910915,150.623180181704));
#161842=CARTESIAN_POINT('Ctrl Pts',(47.5663978459836,-3.12348834816712,
150.603618892545));
#161843=CARTESIAN_POINT('Ctrl Pts',(48.1113780735535,-3.23202446786912,
150.489465612828));
#161844=CARTESIAN_POINT('Ctrl Pts',(48.6629381266314,-3.41049029579194,
150.261453965642));
#161845=CARTESIAN_POINT('Ctrl Pts',(49.1443489753141,-3.635520285376,149.942403436868));
#161846=CARTESIAN_POINT('Ctrl Pts',(49.5482221961931,-3.90246681878571,
149.530695579774));
#161847=CARTESIAN_POINT('Ctrl Pts',(49.8535100390613,-4.20074183020728,
149.031213928958));
#161848=CARTESIAN_POINT('Ctrl Pts',(50.0383897472154,-4.51559898034788,
148.455188846487));
#161849=CARTESIAN_POINT('Ctrl Pts',(50.0820805354509,-4.82867960015004,
147.821400051784));
#161850=CARTESIAN_POINT('Ctrl Pts',(49.9702782955123,-5.11394793309396,
147.169851980777));
#161851=CARTESIAN_POINT('Ctrl Pts',(49.7269715640286,-5.33649748624922,
146.584712317804));
#161852=CARTESIAN_POINT('Ctrl Pts',(49.501802503755,-5.44981452949935,146.242505436702));
#161853=CARTESIAN_POINT('Ctrl Pts',(49.3881546506291,-5.49518876667419,
146.096925017937));
#161854=CARTESIAN_POINT('Ctrl Pts',(46.5324438218759,7.52248810062492,147.869391743406));
#161855=CARTESIAN_POINT('Ctrl Pts',(46.5603292779128,7.46045053430261,147.89544515674));
#161856=CARTESIAN_POINT('Ctrl Pts',(46.6159580166382,7.32046069363766,147.95431904588));
#161857=CARTESIAN_POINT('Ctrl Pts',(46.6798388267066,7.09643606942087,148.044098887596));
#161858=CARTESIAN_POINT('Ctrl Pts',(46.7208885772989,6.86371624916407,148.129036809144));
#161859=CARTESIAN_POINT('Ctrl Pts',(46.7379483378916,6.65435052142963,148.198035168892));
#161860=CARTESIAN_POINT('Ctrl Pts',(46.7361607135675,6.48128066160652,148.250639358319));
#161861=CARTESIAN_POINT('Ctrl Pts',(46.7205136063572,6.34960404611417,148.289497564637));
#161862=CARTESIAN_POINT('Ctrl Pts',(46.694714023938,6.2593031987902,148.31804002652));
#161863=CARTESIAN_POINT('Ctrl Pts',(46.6606708856686,6.20711170250637,148.339617470557));
#161864=CARTESIAN_POINT('Ctrl Pts',(46.6177995501911,6.19016220445405,148.357048251876));
#161865=CARTESIAN_POINT('Ctrl Pts',(46.5686258931354,6.20853508983156,148.370685212542));
#161866=CARTESIAN_POINT('Ctrl Pts',(46.5308147637076,6.24060354711479,148.378440266552));
#161867=CARTESIAN_POINT('Ctrl Pts',(46.513318796367,6.25810836185102,148.381614882767));
#161868=CARTESIAN_POINT('Ctrl Pts',(46.817140996116,6.12671552903897,147.305203746767));
#161869=CARTESIAN_POINT('Ctrl Pts',(46.8673279171114,6.07422688234627,147.318945502478));
#161870=CARTESIAN_POINT('Ctrl Pts',(46.9750608726876,5.95569480282076,147.355269739942));
#161871=CARTESIAN_POINT('Ctrl Pts',(47.1266195294122,5.76226877571011,147.434925106998));
#161872=CARTESIAN_POINT('Ctrl Pts',(47.255865560854,5.54983848865781,147.547759376126));
#161873=CARTESIAN_POINT('Ctrl Pts',(47.3376267684437,5.34161667880711,147.680939984286));
#161874=CARTESIAN_POINT('Ctrl Pts',(47.3636311271785,5.14998292950563,147.821022835015));
#161875=CARTESIAN_POINT('Ctrl Pts',(47.3338957106381,4.98465908606635,147.954869946796));
#161876=CARTESIAN_POINT('Ctrl Pts',(47.254316429973,4.85285295357408,148.071673571935));
#161877=CARTESIAN_POINT('Ctrl Pts',(47.1331847450447,4.75839853982045,148.164772631859));
#161878=CARTESIAN_POINT('Ctrl Pts',(46.9757466504496,4.70373740704304,148.230884782075));
#161879=CARTESIAN_POINT('Ctrl Pts',(46.8036079323038,4.69670712590793,148.261696412376));
#161880=CARTESIAN_POINT('Ctrl Pts',(46.6850631980176,4.72028365496785,148.262424896767));
#161881=CARTESIAN_POINT('Ctrl Pts',(46.633692194392,4.73559534664208,148.259359050582));
#161882=CARTESIAN_POINT('Ctrl Pts',(47.9396334410783,5.35422595109969,146.60462115314));
#161883=CARTESIAN_POINT('Ctrl Pts',(48.0239970756342,5.30839102285964,146.665822950002));
#161884=CARTESIAN_POINT('Ctrl Pts',(48.1989133885865,5.20066734658126,146.814095843857));
#161885=CARTESIAN_POINT('Ctrl Pts',(48.4212132744159,5.00858483897843,147.088194437697));
#161886=CARTESIAN_POINT('Ctrl Pts',(48.5791529552626,4.7764715436373,147.422999102021));
#161887=CARTESIAN_POINT('Ctrl Pts',(48.6387109314665,4.52773568939189,147.778764100921));
#161888=CARTESIAN_POINT('Ctrl Pts',(48.5934003704984,4.27903982375646,148.12740068613));
#161889=CARTESIAN_POINT('Ctrl Pts',(48.4490402052191,4.04632339032457,148.44525754295));
#161890=CARTESIAN_POINT('Ctrl Pts',(48.2197557951557,3.84350785940696,148.714483555535));
#161891=CARTESIAN_POINT('Ctrl Pts',(47.9216132493413,3.67976832257381,148.925589113316));
#161892=CARTESIAN_POINT('Ctrl Pts',(47.5630635699461,3.56038028428392,149.075112755935));
#161893=CARTESIAN_POINT('Ctrl Pts',(47.1895622382968,3.50130545071206,149.146868532606));
#161894=CARTESIAN_POINT('Ctrl Pts',(46.9401269640137,3.49770213436046,149.151755253245));
#161895=CARTESIAN_POINT('Ctrl Pts',(46.8332290949316,3.50247108819423,149.146543148058));
#161896=CARTESIAN_POINT('Ctrl Pts',(49.3696542944107,5.56994442846003,146.098600073015));
#161897=CARTESIAN_POINT('Ctrl Pts',(49.4839247680716,5.52472479241387,146.244613426018));
#161898=CARTESIAN_POINT('Ctrl Pts',(49.7093660752448,5.41205425801527,146.586448596255));
#161899=CARTESIAN_POINT('Ctrl Pts',(49.9520523257794,5.19142551199444,147.1677028901));
#161900=CARTESIAN_POINT('Ctrl Pts',(50.0656281080245,4.90895494508271,147.81369289954));
#161901=CARTESIAN_POINT('Ctrl Pts',(50.0265670092713,4.5971859703998,148.445295281496));
#161902=CARTESIAN_POINT('Ctrl Pts',(49.8445238848551,4.27988597809273,149.025039624157));
#161903=CARTESIAN_POINT('Ctrl Pts',(49.5391514088654,3.97786793806996,149.529000627391));
#161904=CARTESIAN_POINT('Ctrl Pts',(49.1349573323231,3.70808382583412,149.94280572139));
#161905=CARTESIAN_POINT('Ctrl Pts',(48.6535017677747,3.48076734080204,150.262656238905));
#161906=CARTESIAN_POINT('Ctrl Pts',(48.102301047001,3.30021419891055,150.490917802173));
#161907=CARTESIAN_POINT('Ctrl Pts',(47.5441635048093,3.18703933991356,150.60804513497));
#161908=CARTESIAN_POINT('Ctrl Pts',(47.1755136133758,3.15040805459456,150.626310541581));
#161909=CARTESIAN_POINT('Ctrl Pts',(47.0176680117271,3.1412650586095,150.624060276346));
#161910=CARTESIAN_POINT('Origin',(47.0941826981424,6.07477576504754,151.320735005098));
#161911=CARTESIAN_POINT('Ctrl Pts',(46.6350328996003,6.23120586969005,148.359003259099));
#161912=CARTESIAN_POINT('Ctrl Pts',(45.724353855216,6.14473278514312,148.521871668148));
#161913=CARTESIAN_POINT('Ctrl Pts',(43.6840233800751,5.93846932051504,148.889307660513));
#161914=CARTESIAN_POINT('Ctrl Pts',(40.885700375115,5.61210790098104,149.401962579257));
#161915=CARTESIAN_POINT('Ctrl Pts',(38.998434282127,5.35951593354733,149.754100140409));
#161916=CARTESIAN_POINT('Ctrl Pts',(38.2399008107496,5.25187133532221,149.896819266026));
#161917=CARTESIAN_POINT('Ctrl Pts',(46.771908326183,5.20474630002223,148.283570245222));
#161918=CARTESIAN_POINT('Ctrl Pts',(45.8628998835332,5.11971407145539,148.429859227114));
#161919=CARTESIAN_POINT('Ctrl Pts',(43.8266248407972,4.91768494165792,148.759481314297));
#161920=CARTESIAN_POINT('Ctrl Pts',(41.0350814900977,4.6006665917656,149.217962899385));
#161921=CARTESIAN_POINT('Ctrl Pts',(39.1534552270697,4.35707271562612,149.531851254533));
#161922=CARTESIAN_POINT('Ctrl Pts',(38.3974166265721,4.25356346129957,149.658875621596));
#161923=CARTESIAN_POINT('Ctrl Pts',(46.9815148757575,4.27883604249698,148.7040456843));
#161924=CARTESIAN_POINT('Ctrl Pts',(46.0750906810986,4.18751069795957,148.835189525106));
#161925=CARTESIAN_POINT('Ctrl Pts',(44.0450879043102,3.97201764509772,149.129836463091));
#161926=CARTESIAN_POINT('Ctrl Pts',(41.2640257099561,3.63882464480218,149.536736352468));
#161927=CARTESIAN_POINT('Ctrl Pts',(39.3911145657453,3.3861418555883,149.813150958076));
#161928=CARTESIAN_POINT('Ctrl Pts',(38.6389304649779,3.27934325045187,149.924608447612));
#161929=CARTESIAN_POINT('Ctrl Pts',(47.2130425126618,3.67792196340846,149.518503505342));
#161930=CARTESIAN_POINT('Ctrl Pts',(46.3094897731806,3.57409502453192,149.639607775137));
#161931=CARTESIAN_POINT('Ctrl Pts',(44.2864556564767,3.33070353610726,149.910596530947));
#161932=CARTESIAN_POINT('Ctrl Pts',(41.5170354178634,2.95973900927576,150.281010112081));
#161933=CARTESIAN_POINT('Ctrl Pts',(39.6538020779683,2.68208351620199,150.529810313275));
#161934=CARTESIAN_POINT('Ctrl Pts',(38.9058977491478,2.56536822628038,150.629602322079));
#161935=CARTESIAN_POINT('Origin',(82.0458803142802,-1.76619892465473,142.111155740591));
#161936=CARTESIAN_POINT('Origin',(26.7764851389615,-2.04263841746052E-14,
151.856993361954));
#221635=UNCERTAINTY_MEASURE_WITH_UNIT(LENGTH_MEASURE(0.01),#221663,
'DISTANCE_ACCURACY_VALUE',
'Maximum model space distance between geometric entities at asserted c
onnectivities');
#221647=UNCERTAINTY_MEASURE_WITH_UNIT(LENGTH_MEASURE(0.01),#221663,
'DISTANCE_ACCURACY_VALUE',
'Maximum model space distance between geometric entities at asserted c
onnectivities');
#221650=(
GEOMETRIC_REPRESENTATION_CONTEXT(3)
GLOBAL_UNCERTAINTY_ASSIGNED_CONTEXT((#221635))
GLOBAL_UNIT_ASSIGNED_CONTEXT((#221663,#221665,#221666))
REPRESENTATION_CONTEXT('','3D')
);
#221662=(
GEOMETRIC_REPRESENTATION_CONTEXT(3)
GLOBAL_UNCERTAINTY_ASSIGNED_CONTEXT((#221647))
GLOBAL_UNIT_ASSIGNED_CONTEXT((#221663,#221665,#221666))
REPRESENTATION_CONTEXT('','3D')
);
#221663=(
LENGTH_UNIT()
NAMED_UNIT(*)
SI_UNIT(.MILLI.,.METRE.)
);
#221665=(
NAMED_UNIT(*)
PLANE_ANGLE_UNIT()
SI_UNIT($,.RADIAN.)
);
#221666=(
NAMED_UNIT(*)
SI_UNIT($,.STERADIAN.)
SOLID_ANGLE_UNIT()
);
#221669=SHAPE_DEFINITION_REPRESENTATION(#221683,#221710);
#221683=PRODUCT_DEFINITION_SHAPE('',$,#221725);
#221710=SHAPE_REPRESENTATION('',(#80379),#221650);
#221722=PRODUCT_DEFINITION_CONTEXT('part definition',#221766,'design');
#221725=PRODUCT_DEFINITION('2026-10-05-23-02-27-655','Control Handle',#221739,
#221722);
#221739=PRODUCT_DEFINITION_FORMATION('',$,#221770);
#221766=APPLICATION_CONTEXT(
'Core Data for Automotive Mechanical Design Process');
#221767=PRODUCT_CONTEXT('part definition',#221766,'mechanical');
#221770=PRODUCT('2026-10-05-23-02-27-655','Control Handle',$,(#221767));
#221783=PRESENTATION_STYLE_ASSIGNMENT((#221785));
#221785=SURFACE_STYLE_USAGE(.BOTH.,#221787);
#221787=SURFACE_SIDE_STYLE('',(#221789));
#221789=SURFACE_STYLE_FILL_AREA(#221791);
#221791=FILL_AREA_STYLE('Opaque(202,209,238)',(#221793));
#221793=FILL_AREA_STYLE_COLOUR('Opaque(202,209,238)',#221795);
#221795=COLOUR_RGB('Opaque(202,209,238)', 0.09019608, 0.27058824, 0.51372549);
ENDSEC;
END-ISO-10303-21;
